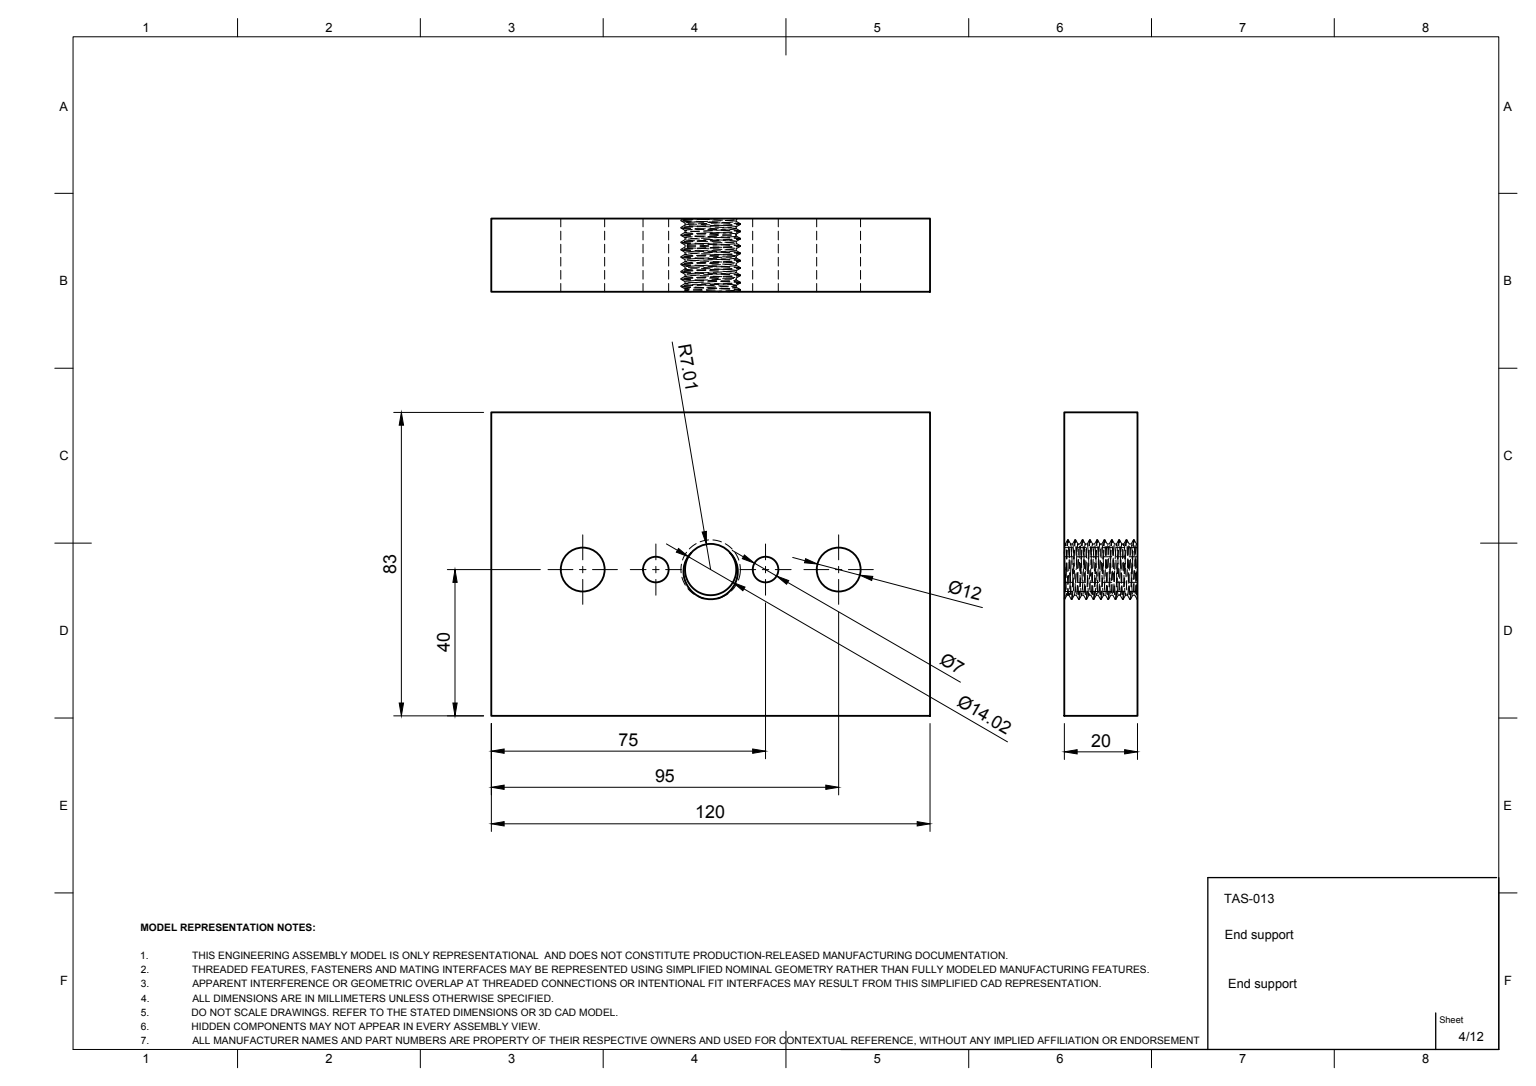
ISO-10303-21;
HEADER;
/* Generated by software containing ST-Developer
 * from STEP Tools, Inc. (www.steptools.com) 
 */

FILE_DESCRIPTION(
/* description */ (
'Independent guided parallel-jaw bracket clamp. Two12mm guide rods, re
placeable bronze sleeves, captured swiveling spindle, replaceable jaw 
pads and modeled M16x2 screw. Native slider/revolute joints linked2mm 
per revolution. Nominal opening0..122 with initial28mm. Base and two i
dentical supports welded. Standard fits, weld details and clamp load r
equire engineering selection.'),
/* implementation_level */ '2;1');

FILE_NAME(
/* name */ 'End support.step',
/* time_stamp */ '2026-11-14T09:15:44-08:00',
/* author */ (''),
/* organization */ (''),
/* preprocessor_version */ 'ST-DEVELOPER v20.2',
/* originating_system */ 'Autodesk Translation Framework v15.17.0.0',
/* authorisation */ '');

FILE_SCHEMA (('AUTOMOTIVE_DESIGN { 1 0 10303 214 3 1 1 }'));
ENDSEC;

DATA;
#10=MECHANICAL_DESIGN_GEOMETRIC_PRESENTATION_REPRESENTATION('',(#920),#105806);
#97=B_SPLINE_SURFACE_WITH_KNOTS('',3,3,((#78284,#78285,#78286,#78287,#78288,
#78289,#78290,#78291,#78292,#78293,#78294,#78295,#78296,#78297,#78298,#78299,
#78300,#78301,#78302,#78303,#78304,#78305,#78306,#78307,#78308,#78309,#78310,
#78311,#78312,#78313,#78314,#78315,#78316,#78317,#78318,#78319,#78320,#78321,
#78322,#78323,#78324,#78325,#78326,#78327,#78328,#78329,#78330,#78331,#78332,
#78333,#78334,#78335,#78336,#78337,#78338,#78339,#78340,#78341,#78342,#78343,
#78344,#78345,#78346,#78347,#78348,#78349,#78350,#78351,#78352,#78353,#78354,
#78355,#78356,#78357,#78358,#78359,#78360,#78361,#78362,#78363,#78364,#78365,
#78366,#78367,#78368,#78369,#78370,#78371,#78372,#78373,#78374,#78375,#78376,
#78377,#78378,#78379,#78380,#78381,#78382,#78383,#78384,#78385,#78386,#78387,
#78388,#78389,#78390,#78391,#78392,#78393,#78394,#78395,#78396,#78397,#78398,
#78399,#78400,#78401,#78402,#78403,#78404,#78405,#78406,#78407,#78408,#78409,
#78410,#78411,#78412,#78413,#78414,#78415,#78416),(#78417,#78418,#78419,
#78420,#78421,#78422,#78423,#78424,#78425,#78426,#78427,#78428,#78429,#78430,
#78431,#78432,#78433,#78434,#78435,#78436,#78437,#78438,#78439,#78440,#78441,
#78442,#78443,#78444,#78445,#78446,#78447,#78448,#78449,#78450,#78451,#78452,
#78453,#78454,#78455,#78456,#78457,#78458,#78459,#78460,#78461,#78462,#78463,
#78464,#78465,#78466,#78467,#78468,#78469,#78470,#78471,#78472,#78473,#78474,
#78475,#78476,#78477,#78478,#78479,#78480,#78481,#78482,#78483,#78484,#78485,
#78486,#78487,#78488,#78489,#78490,#78491,#78492,#78493,#78494,#78495,#78496,
#78497,#78498,#78499,#78500,#78501,#78502,#78503,#78504,#78505,#78506,#78507,
#78508,#78509,#78510,#78511,#78512,#78513,#78514,#78515,#78516,#78517,#78518,
#78519,#78520,#78521,#78522,#78523,#78524,#78525,#78526,#78527,#78528,#78529,
#78530,#78531,#78532,#78533,#78534,#78535,#78536,#78537,#78538,#78539,#78540,
#78541,#78542,#78543,#78544,#78545,#78546,#78547,#78548,#78549),(#78550,
#78551,#78552,#78553,#78554,#78555,#78556,#78557,#78558,#78559,#78560,#78561,
#78562,#78563,#78564,#78565,#78566,#78567,#78568,#78569,#78570,#78571,#78572,
#78573,#78574,#78575,#78576,#78577,#78578,#78579,#78580,#78581,#78582,#78583,
#78584,#78585,#78586,#78587,#78588,#78589,#78590,#78591,#78592,#78593,#78594,
#78595,#78596,#78597,#78598,#78599,#78600,#78601,#78602,#78603,#78604,#78605,
#78606,#78607,#78608,#78609,#78610,#78611,#78612,#78613,#78614,#78615,#78616,
#78617,#78618,#78619,#78620,#78621,#78622,#78623,#78624,#78625,#78626,#78627,
#78628,#78629,#78630,#78631,#78632,#78633,#78634,#78635,#78636,#78637,#78638,
#78639,#78640,#78641,#78642,#78643,#78644,#78645,#78646,#78647,#78648,#78649,
#78650,#78651,#78652,#78653,#78654,#78655,#78656,#78657,#78658,#78659,#78660,
#78661,#78662,#78663,#78664,#78665,#78666,#78667,#78668,#78669,#78670,#78671,
#78672,#78673,#78674,#78675,#78676,#78677,#78678,#78679,#78680,#78681,#78682),
(#78683,#78684,#78685,#78686,#78687,#78688,#78689,#78690,#78691,#78692,
#78693,#78694,#78695,#78696,#78697,#78698,#78699,#78700,#78701,#78702,#78703,
#78704,#78705,#78706,#78707,#78708,#78709,#78710,#78711,#78712,#78713,#78714,
#78715,#78716,#78717,#78718,#78719,#78720,#78721,#78722,#78723,#78724,#78725,
#78726,#78727,#78728,#78729,#78730,#78731,#78732,#78733,#78734,#78735,#78736,
#78737,#78738,#78739,#78740,#78741,#78742,#78743,#78744,#78745,#78746,#78747,
#78748,#78749,#78750,#78751,#78752,#78753,#78754,#78755,#78756,#78757,#78758,
#78759,#78760,#78761,#78762,#78763,#78764,#78765,#78766,#78767,#78768,#78769,
#78770,#78771,#78772,#78773,#78774,#78775,#78776,#78777,#78778,#78779,#78780,
#78781,#78782,#78783,#78784,#78785,#78786,#78787,#78788,#78789,#78790,#78791,
#78792,#78793,#78794,#78795,#78796,#78797,#78798,#78799,#78800,#78801,#78802,
#78803,#78804,#78805,#78806,#78807,#78808,#78809,#78810,#78811,#78812,#78813,
#78814,#78815)),.UNSPECIFIED.,.F.,.F.,.F.,(4,4),(4,1,1,1,1,1,1,1,1,1,1,
1,1,1,1,1,1,1,1,1,1,1,1,1,1,1,1,1,1,1,1,1,1,1,1,1,1,1,1,1,1,1,1,1,1,1,1,
1,1,1,1,1,1,1,1,1,1,1,1,1,1,1,1,1,1,1,1,1,1,1,1,1,1,1,1,1,1,1,1,1,1,1,1,
1,1,1,1,1,1,1,1,1,1,1,1,1,1,1,1,1,1,1,1,1,1,1,1,1,1,1,1,1,1,1,1,1,1,1,1,
1,1,1,1,1,1,1,1,1,1,1,4),(-8.529467209505E-5,0.128694174119411),(11.8548225190662,
12.3537726257656,12.8526374377929,13.3515022498203,13.8503670618476,14.3492318738749,
14.8480966859023,15.3469614979296,15.8458263099569,16.3446911219842,16.8435559340116,
17.3424207460389,17.8412855580662,18.3401503700936,18.8390151821209,19.3378799941482,
19.8367448061755,20.3356096182029,20.8344744302302,21.3333392422575,21.8322040542849,
22.3310688663122,22.8299336783395,23.3287984903668,23.8276633023942,24.3265281144215,
24.8253929264488,25.3242577384762,25.8231225505035,26.3219873625308,26.8208521745581,
27.3197169865855,27.8185817986128,28.3174466106401,28.8163114226675,29.3151762346948,
29.8140410467221,30.3129058587495,30.8117706707768,31.3106354828041,31.8095002948314,
32.3083651068588,32.8072299188861,33.3060947309134,33.8049595429408,34.3038243549681,
34.8026891669954,35.3015539790227,35.8004187910501,36.2992836030774,36.7981484151047,
37.2970132271321,37.7958780391594,38.2947428511867,38.793607663214,39.2924724752414,
39.7913372872687,40.290202099296,40.7890669113234,41.2879317233507,41.786796535378,
42.2856613474054,42.7845261594327,43.28339097146,43.7822557834873,44.2811205955147,
44.779985407542,45.2788502195693,45.7777150315967,46.276579843624,46.7754446556513,
47.2743094676786,47.773174279706,48.2720390917333,48.7709039037606,49.269768715788,
49.7686335278153,50.2674983398426,50.76636315187,51.2652279638973,51.7640927759246,
52.2629575879519,52.7618223999793,53.2606872120066,53.7595520240339,54.2584168360613,
54.7572816480886,55.2561464601159,55.7550112721432,56.2538760841706,56.7527408961979,
57.2516057082252,57.7504705202526,58.2493353322799,58.7482001443072,59.2470649563345,
59.7459297683619,60.2447945803892,60.7436593924165,61.2425242044439,61.7413890164712,
62.2402538284985,62.7391186405258,63.2379834525532,63.7368482645805,64.2357130766078,
64.7345778886352,65.2334427006625,65.7323075126898,66.2311723247172,66.7300371367445,
67.2289019487718,67.7277667607991,68.2266315728265,68.7254963848538,69.2243611968811,
69.7232260089085,70.2220908209358,70.7209556329631,71.2198204449904,71.7186852570178,
72.2175500690451,72.7164148810724,73.2152796930998,73.7141445051271,74.2130093171544,
74.7118741291818,75.2107389412091,75.7096037532364,76.2084685652637,76.7073333772911),
 .UNSPECIFIED.);
#98=B_SPLINE_SURFACE_WITH_KNOTS('',3,3,((#79039,#79040,#79041,#79042,#79043,
#79044,#79045,#79046,#79047,#79048,#79049,#79050,#79051,#79052,#79053,#79054,
#79055,#79056,#79057,#79058,#79059,#79060,#79061,#79062,#79063,#79064,#79065,
#79066,#79067,#79068,#79069,#79070,#79071,#79072,#79073,#79074,#79075,#79076,
#79077,#79078,#79079,#79080,#79081,#79082,#79083,#79084,#79085,#79086,#79087,
#79088,#79089,#79090,#79091,#79092,#79093,#79094,#79095,#79096,#79097,#79098,
#79099,#79100,#79101,#79102,#79103,#79104,#79105,#79106,#79107,#79108,#79109,
#79110,#79111,#79112,#79113,#79114,#79115,#79116,#79117,#79118,#79119,#79120,
#79121,#79122,#79123,#79124,#79125,#79126,#79127,#79128,#79129,#79130,#79131,
#79132,#79133,#79134,#79135,#79136,#79137,#79138,#79139,#79140,#79141,#79142,
#79143,#79144,#79145,#79146,#79147,#79148,#79149,#79150,#79151,#79152,#79153,
#79154,#79155,#79156,#79157,#79158,#79159,#79160,#79161,#79162,#79163,#79164,
#79165,#79166,#79167,#79168,#79169,#79170,#79171),(#79172,#79173,#79174,
#79175,#79176,#79177,#79178,#79179,#79180,#79181,#79182,#79183,#79184,#79185,
#79186,#79187,#79188,#79189,#79190,#79191,#79192,#79193,#79194,#79195,#79196,
#79197,#79198,#79199,#79200,#79201,#79202,#79203,#79204,#79205,#79206,#79207,
#79208,#79209,#79210,#79211,#79212,#79213,#79214,#79215,#79216,#79217,#79218,
#79219,#79220,#79221,#79222,#79223,#79224,#79225,#79226,#79227,#79228,#79229,
#79230,#79231,#79232,#79233,#79234,#79235,#79236,#79237,#79238,#79239,#79240,
#79241,#79242,#79243,#79244,#79245,#79246,#79247,#79248,#79249,#79250,#79251,
#79252,#79253,#79254,#79255,#79256,#79257,#79258,#79259,#79260,#79261,#79262,
#79263,#79264,#79265,#79266,#79267,#79268,#79269,#79270,#79271,#79272,#79273,
#79274,#79275,#79276,#79277,#79278,#79279,#79280,#79281,#79282,#79283,#79284,
#79285,#79286,#79287,#79288,#79289,#79290,#79291,#79292,#79293,#79294,#79295,
#79296,#79297,#79298,#79299,#79300,#79301,#79302,#79303,#79304),(#79305,
#79306,#79307,#79308,#79309,#79310,#79311,#79312,#79313,#79314,#79315,#79316,
#79317,#79318,#79319,#79320,#79321,#79322,#79323,#79324,#79325,#79326,#79327,
#79328,#79329,#79330,#79331,#79332,#79333,#79334,#79335,#79336,#79337,#79338,
#79339,#79340,#79341,#79342,#79343,#79344,#79345,#79346,#79347,#79348,#79349,
#79350,#79351,#79352,#79353,#79354,#79355,#79356,#79357,#79358,#79359,#79360,
#79361,#79362,#79363,#79364,#79365,#79366,#79367,#79368,#79369,#79370,#79371,
#79372,#79373,#79374,#79375,#79376,#79377,#79378,#79379,#79380,#79381,#79382,
#79383,#79384,#79385,#79386,#79387,#79388,#79389,#79390,#79391,#79392,#79393,
#79394,#79395,#79396,#79397,#79398,#79399,#79400,#79401,#79402,#79403,#79404,
#79405,#79406,#79407,#79408,#79409,#79410,#79411,#79412,#79413,#79414,#79415,
#79416,#79417,#79418,#79419,#79420,#79421,#79422,#79423,#79424,#79425,#79426,
#79427,#79428,#79429,#79430,#79431,#79432,#79433,#79434,#79435,#79436,#79437),
(#79438,#79439,#79440,#79441,#79442,#79443,#79444,#79445,#79446,#79447,
#79448,#79449,#79450,#79451,#79452,#79453,#79454,#79455,#79456,#79457,#79458,
#79459,#79460,#79461,#79462,#79463,#79464,#79465,#79466,#79467,#79468,#79469,
#79470,#79471,#79472,#79473,#79474,#79475,#79476,#79477,#79478,#79479,#79480,
#79481,#79482,#79483,#79484,#79485,#79486,#79487,#79488,#79489,#79490,#79491,
#79492,#79493,#79494,#79495,#79496,#79497,#79498,#79499,#79500,#79501,#79502,
#79503,#79504,#79505,#79506,#79507,#79508,#79509,#79510,#79511,#79512,#79513,
#79514,#79515,#79516,#79517,#79518,#79519,#79520,#79521,#79522,#79523,#79524,
#79525,#79526,#79527,#79528,#79529,#79530,#79531,#79532,#79533,#79534,#79535,
#79536,#79537,#79538,#79539,#79540,#79541,#79542,#79543,#79544,#79545,#79546,
#79547,#79548,#79549,#79550,#79551,#79552,#79553,#79554,#79555,#79556,#79557,
#79558,#79559,#79560,#79561,#79562,#79563,#79564,#79565,#79566,#79567,#79568,
#79569,#79570)),.UNSPECIFIED.,.F.,.F.,.F.,(4,4),(4,1,1,1,1,1,1,1,1,1,1,
1,1,1,1,1,1,1,1,1,1,1,1,1,1,1,1,1,1,1,1,1,1,1,1,1,1,1,1,1,1,1,1,1,1,1,1,
1,1,1,1,1,1,1,1,1,1,1,1,1,1,1,1,1,1,1,1,1,1,1,1,1,1,1,1,1,1,1,1,1,1,1,1,
1,1,1,1,1,1,1,1,1,1,1,1,1,1,1,1,1,1,1,1,1,1,1,1,1,1,1,1,1,1,1,1,1,1,1,1,
1,1,1,1,1,1,1,1,1,1,1,4),(-6.05230187934505E-5,0.12871890615391),(14.3988535768129,
14.8977183888402,15.3965832008676,15.8954480128949,16.3943128249222,16.8931776369496,
17.3920424489769,17.8909072610042,18.3897720730315,18.8886368850589,19.3875016970862,
19.8863665091135,20.3852313211409,20.8840961331682,21.3829609451955,21.8818257572228,
22.3806905692502,22.8795553812775,23.3784201933048,23.8772850053322,24.3761498173595,
24.8750146293868,25.3738794414141,25.8727442534415,26.3716090654688,26.8704738774961,
27.3693386895235,27.8682035015508,28.3670683135781,28.8659331256054,29.3647979376328,
29.8636627496601,30.3625275616874,30.8613923737148,31.3602571857421,31.8591219977694,
32.3579868097967,32.8568516218241,33.3557164338514,33.8545812458787,34.3534460579061,
34.8523108699334,35.3511756819607,35.8500404939881,36.3489053060154,36.8477701180427,
37.34663493007,37.8454997420974,38.3443645541247,38.843229366152,39.3420941781794,
39.8409589902067,40.339823802234,40.8386886142613,41.3375534262887,41.836418238316,
42.3352830503433,42.8341478623707,43.333012674398,43.8318774864253,44.3307422984526,
44.82960711048,45.3284719225073,45.8273367345346,46.326201546562,46.8250663585893,
47.3239311706166,47.8227959826439,48.3216607946713,48.8205256066986,49.3193904187259,
49.8182552307533,50.3171200427806,50.8159848548079,51.3148496668353,51.8137144788626,
52.3125792908899,52.8114441029172,53.3103089149446,53.8091737269719,54.3080385389992,
54.8069033510266,55.3057681630539,55.8046329750812,56.3034977871085,56.8023625991359,
57.3012274111632,57.8000922231905,58.2989570352179,58.7978218472452,59.2966866592725,
59.7955514712998,60.2944162833272,60.7932810953545,61.2921459073818,61.7910107194092,
62.2898755314365,62.7887403434638,63.2876051554911,63.7864699675185,64.2853347795458,
64.7841995915731,65.2830644036005,65.7819292156278,66.2807940276551,66.7796588396825,
67.2785236517098,67.7773884637371,68.2762532757644,68.7751180877918,69.2739828998191,
69.7728477118464,70.2717125238738,70.7705773359011,71.2694421479284,71.7683069599557,
72.2671717719831,72.7660365840104,73.2649013960377,73.7637662080651,74.2626310200924,
74.7614958321197,75.260360644147,75.7592254561744,76.2580902682017,76.756955080229,
77.2558198922564,77.7546847042837,78.253549516311,78.7524143283383,79.2513644065442),
 .UNSPECIFIED.);
#564=B_SPLINE_CURVE_WITH_KNOTS('',3,(#71903,#71904,#71905,#71906,#71907,
#71908,#71909,#71910),.UNSPECIFIED.,.F.,.F.,(4,1,1,1,1,4),(74.4819856391522,
74.7118741291818,75.2107389412091,75.7096037532364,76.2084685652637,76.7073333772911),
 .UNSPECIFIED.);
#565=B_SPLINE_CURVE_WITH_KNOTS('',3,(#71913,#71914,#71915,#71916,#71917,
#71918,#71919,#71920,#71921),.UNSPECIFIED.,.F.,.F.,(4,1,1,1,1,1,4),(74.4820002615382,
74.7614958321197,75.260360644147,75.7592254561744,76.2580902682017,76.756955080229,
77.2307066486088),.UNSPECIFIED.);
#566=B_SPLINE_CURVE_WITH_KNOTS('',3,(#71927,#71928,#71929,#71930,#71931,
#71932,#71933,#71934,#71935,#71936,#71937,#71938,#71939,#71940,#71941,#71942,
#71943,#71944,#71945,#71946,#71947,#71948,#71949,#71950,#71951,#71952,#71953,
#71954,#71955,#71956,#71957,#71958,#71959,#71960,#71961,#71962,#71963,#71964,
#71965,#71966,#71967,#71968,#71969,#71970,#71971,#71972,#71973,#71974,#71975,
#71976,#71977,#71978,#71979,#71980,#71981,#71982,#71983,#71984,#71985,#71986,
#71987,#71988,#71989,#71990,#71991,#71992,#71993,#71994,#71995,#71996,#71997,
#71998,#71999,#72000,#72001,#72002,#72003,#72004,#72005,#72006,#72007,#72008,
#72009,#72010,#72011,#72012,#72013,#72014,#72015,#72016,#72017,#72018,#72019,
#72020,#72021,#72022,#72023,#72024,#72025,#72026,#72027,#72028,#72029,#72030,
#72031,#72032,#72033,#72034,#72035,#72036,#72037,#72038,#72039,#72040,#72041,
#72042,#72043,#72044,#72045,#72046,#72047,#72048,#72049,#72050,#72051,#72052,
#72053,#72054,#72055,#72056,#72057,#72058,#72059,#72060,#72061,#72062,#72063,
#72064,#72065,#72066,#72067,#72068,#72069,#72070,#72071,#72072,#72073,#72074,
#72075,#72076,#72077,#72078,#72079,#72080,#72081,#72082,#72083,#72084,#72085,
#72086,#72087,#72088,#72089,#72090,#72091,#72092,#72093,#72094,#72095,#72096,
#72097,#72098,#72099,#72100,#72101),.UNSPECIFIED.,.F.,.F.,(4,3,3,3,3,3,
3,3,3,3,3,3,3,3,3,3,3,3,3,3,3,3,3,3,3,3,3,3,3,3,3,3,3,3,3,3,3,3,3,3,3,3,
3,3,3,3,3,3,3,3,3,3,3,3,3,3,3,3,4),(68.1987975186712,68.2266315728265,68.3041236122402,
68.3816013676368,68.4590704189412,68.5365456775087,68.6140206493277,68.6915121862316,
68.7254963848538,68.8029883992075,68.8804661294451,68.9579351555709,69.0354103891201,
69.1128853360578,69.1903768484489,69.2243611968811,69.3018532647296,69.3793310486332,
69.456800128424,69.5342754152362,69.6117504151087,69.6892419796001,69.7232260089085,
69.800717988916,69.8781956847726,69.9556646765945,70.0331398762059,70.1106147894785,
70.1881062688295,70.2220908209358,70.2995828974163,70.3770606897927,70.4545297778736,
70.5320050726442,70.6094800802699,70.6869716521594,70.7209556329631,70.7984477160451,
70.8759255156548,70.9533946115695,71.0308699150024,71.1083449317504,71.1858365133831,
71.2198204449904,71.2973121319933,71.3747895331616,71.4522582295674,71.5297331348839,
71.6072077550478,71.684698944971,71.7186852570178,71.7961782868195,71.8736570365031,
71.9511270827911,72.0286033299696,72.1060792849236,72.1835717903897,72.2175500690451,
72.2566310325652),.UNSPECIFIED.);
#567=B_SPLINE_CURVE_WITH_KNOTS('',3,(#72102,#72103,#72104,#72105,#72106,
#72107,#72108,#72109),.UNSPECIFIED.,.F.,.F.,(4,1,1,1,1,4),(72.2566310687215,
72.7164148810724,73.2152796930998,73.7141445051271,74.2130093171544,74.4819856391522),
 .UNSPECIFIED.);
#568=B_SPLINE_CURVE_WITH_KNOTS('',3,(#72111,#72112,#72113,#72114,#72115,
#72116,#72117,#72118,#72119),.UNSPECIFIED.,.F.,.F.,(4,1,1,1,1,1,4),(72.2566310325652,
72.2671717719831,72.7660365840104,73.2649013960377,73.7637662080651,74.2626310200924,
74.4820002615382),.UNSPECIFIED.);
#569=B_SPLINE_CURVE_WITH_KNOTS('',3,(#72120,#72121,#72122,#72123,#72124,
#72125,#72126,#72127,#72128,#72129,#72130,#72131,#72132,#72133,#72134,#72135,
#72136,#72137,#72138,#72139,#72140,#72141,#72142,#72143,#72144,#72145,#72146,
#72147,#72148,#72149,#72150,#72151,#72152,#72153,#72154,#72155,#72156,#72157,
#72158,#72159,#72160,#72161,#72162,#72163,#72164,#72165,#72166,#72167,#72168,
#72169,#72170,#72171,#72172,#72173,#72174,#72175,#72176,#72177,#72178,#72179,
#72180,#72181,#72182,#72183,#72184,#72185,#72186,#72187,#72188,#72189,#72190,
#72191,#72192,#72193,#72194,#72195,#72196,#72197,#72198,#72199,#72200,#72201,
#72202,#72203,#72204,#72205,#72206,#72207,#72208,#72209,#72210,#72211,#72212,
#72213,#72214,#72215,#72216,#72217,#72218,#72219,#72220,#72221,#72222,#72223,
#72224,#72225,#72226,#72227,#72228,#72229,#72230,#72231,#72232,#72233,#72234,
#72235,#72236,#72237,#72238,#72239,#72240,#72241,#72242,#72243,#72244,#72245,
#72246,#72247,#72248,#72249,#72250,#72251,#72252,#72253,#72254,#72255,#72256,
#72257,#72258,#72259,#72260,#72261,#72262,#72263,#72264,#72265,#72266,#72267,
#72268,#72269,#72270,#72271,#72272,#72273,#72274,#72275,#72276,#72277,#72278,
#72279,#72280,#72281,#72282,#72283,#72284,#72285,#72286,#72287,#72288,#72289,
#72290,#72291),.UNSPECIFIED.,.F.,.F.,(4,3,3,3,3,3,3,3,3,3,3,3,3,3,3,3,3,
3,3,3,3,3,3,3,3,3,3,3,3,3,3,3,3,3,3,3,3,3,3,3,3,3,3,3,3,3,3,3,3,3,3,3,3,
3,3,3,3,4),(68.1987898047183,68.2762532757644,68.3537453085195,68.4312230572261,
68.5086921018308,68.586167353733,68.6636423189185,68.7411338492811,68.7751180877918,
68.8526101196304,68.9300878674179,69.0075569111027,69.0850321620932,69.1625071263726,
69.2399986558434,69.2739828998191,69.3514749330283,69.4289526821889,69.5064217272455,
69.5838969795948,69.6613719452233,69.7388634760199,69.7728477118464,69.8503397438658,
69.9278174918377,70.0052865357114,70.0827617868932,70.1602367513658,70.2377282810308,
70.2717125238738,70.3492045547049,70.4266823014742,70.5041513441335,70.5816265940954,
70.6591015573465,70.736593085796,70.7705773359011,70.8480693754309,70.9255471309442,
71.0030161823662,71.0804914410497,71.1579664129848,71.2354579500022,71.2694421479284,
71.3469341620217,71.4244118919975,71.5018809178624,71.5793561511515,71.6568310978316,
71.7343226099682,71.7683069599557,71.8457247371354,71.9231279927475,72.0005225461464,
72.077923117042,72.15532396466,72.2327409413495,72.2566310325652),
 .UNSPECIFIED.);
#570=B_SPLINE_CURVE_WITH_KNOTS('',3,(#72297,#72298,#72299,#72300,#72301,
#72302,#72303,#72304,#72305,#72306,#72307,#72308),.UNSPECIFIED.,.F.,.F.,
(4,1,1,1,1,1,1,1,1,4),(61.9156408615241,62.2402538284985,62.7391186405258,
63.2379834525532,63.7368482645805,64.2357130766078,64.7345778886352,65.2334427006625,
65.7323075126898,65.9734457190118),.UNSPECIFIED.);
#571=B_SPLINE_CURVE_WITH_KNOTS('',3,(#72309,#72310,#72311,#72312,#72313,
#72314,#72315,#72316,#72317,#72318,#72319,#72320,#72321,#72322,#72323,#72324,
#72325,#72326,#72327,#72328,#72329,#72330,#72331,#72332,#72333,#72334,#72335,
#72336,#72337,#72338,#72339,#72340,#72341,#72342,#72343,#72344,#72345,#72346,
#72347,#72348,#72349,#72350,#72351,#72352,#72353,#72354,#72355,#72356,#72357,
#72358,#72359,#72360,#72361,#72362,#72363,#72364,#72365,#72366,#72367,#72368,
#72369,#72370,#72371,#72372,#72373,#72374,#72375,#72376,#72377,#72378,#72379,
#72380,#72381,#72382,#72383,#72384,#72385,#72386,#72387,#72388,#72389,#72390,
#72391,#72392,#72393,#72394,#72395,#72396,#72397,#72398,#72399,#72400,#72401,
#72402),.UNSPECIFIED.,.F.,.F.,(4,3,3,3,3,3,3,3,3,3,3,3,3,3,3,3,3,3,3,3,
3,3,3,3,3,3,3,3,3,3,3,4),(65.9734457253856,66.051752866185,66.1300656952307,
66.2083969560539,66.2311723247172,66.3086643565655,66.3861421043627,66.4636111480579,
66.5410863990578,66.6185613633469,66.6960528928273,66.7300371367445,66.8075291699426,
66.8850069190923,66.9624759641383,67.0399512164768,67.1174261820946,67.1949177128806,
67.2289019487718,67.3063939807927,67.3838717287663,67.4613407726409,67.5388160238239,
67.6162909882975,67.6937825179636,67.7277667607991,67.8052584948873,67.8827358464432,
67.9617512645002,68.0392239583848,68.119010738528,68.1987975186712),
 .UNSPECIFIED.);
#572=B_SPLINE_CURVE_WITH_KNOTS('',3,(#72404,#72405,#72406,#72407,#72408,
#72409,#72410,#72411,#72412,#72413,#72414,#72415,#72416,#72417,#72418,#72419,
#72420,#72421,#72422,#72423,#72424,#72425,#72426,#72427,#72428,#72429,#72430,
#72431,#72432,#72433,#72434,#72435,#72436,#72437,#72438,#72439,#72440,#72441,
#72442,#72443,#72444,#72445,#72446,#72447,#72448,#72449,#72450,#72451,#72452,
#72453,#72454,#72455,#72456,#72457,#72458,#72459,#72460,#72461,#72462,#72463,
#72464,#72465,#72466,#72467,#72468,#72469,#72470,#72471,#72472,#72473,#72474,
#72475,#72476,#72477,#72478,#72479,#72480,#72481,#72482,#72483,#72484,#72485,
#72486,#72487,#72488,#72489,#72490,#72491,#72492,#72493,#72494,#72495,#72496,
#72497),.UNSPECIFIED.,.F.,.F.,(4,3,3,3,3,3,3,3,3,3,3,3,3,3,3,3,3,3,3,3,
3,3,3,3,3,3,3,3,3,3,3,4),(65.9734457253856,66.05113864352,66.1288303647685,
66.2065431816206,66.2807940276551,66.3582860600736,66.4357638084426,66.5132328527091,
66.5907081042758,66.6681830691279,66.7456745991621,66.7796588396825,66.8571508721125,
66.934628620493,67.0120976647703,67.0895729163482,67.1670478812115,67.2445394112565,
67.2785236517098,67.3560156841782,67.433493432597,67.5109624769137,67.5884377285306,
67.6659126934328,67.7434042235161,67.7773884637371,67.8548798500932,67.9323566782865,
68.0098309919021,68.0873000058441,68.1647781672896,68.1987898047183),
 .UNSPECIFIED.);
#573=B_SPLINE_CURVE_WITH_KNOTS('',3,(#72498,#72499,#72500,#72501,#72502,
#72503,#72504,#72505,#72506,#72507,#72508,#72509),.UNSPECIFIED.,.F.,.F.,
(4,1,1,1,1,1,1,1,1,4),(61.9156464171414,62.2898755314365,62.7887403434638,
63.2876051554911,63.7864699675185,64.2853347795458,64.7841995915731,65.2830644036005,
65.7819292156278,65.9734456898724),.UNSPECIFIED.);
#574=B_SPLINE_CURVE_WITH_KNOTS('',3,(#72515,#72516,#72517,#72518,#72519,
#72520,#72521,#72522,#72523,#72524,#72525,#72526,#72527,#72528,#72529,#72530,
#72531,#72532,#72533,#72534,#72535,#72536,#72537,#72538,#72539,#72540,#72541,
#72542,#72543,#72544,#72545,#72546,#72547,#72548,#72549,#72550,#72551,#72552,
#72553,#72554,#72555,#72556,#72557,#72558,#72559,#72560,#72561,#72562,#72563,
#72564,#72565,#72566,#72567,#72568,#72569,#72570,#72571,#72572,#72573,#72574,
#72575,#72576,#72577,#72578,#72579,#72580,#72581,#72582,#72583,#72584,#72585,
#72586,#72587,#72588,#72589,#72590,#72591,#72592,#72593,#72594,#72595,#72596,
#72597,#72598,#72599,#72600,#72601,#72602,#72603,#72604,#72605,#72606,#72607,
#72608,#72609,#72610,#72611,#72612,#72613,#72614,#72615,#72616,#72617,#72618,
#72619,#72620,#72621,#72622,#72623,#72624,#72625,#72626,#72627,#72628,#72629,
#72630,#72631,#72632,#72633,#72634,#72635,#72636,#72637,#72638,#72639,#72640,
#72641,#72642,#72643,#72644,#72645,#72646,#72647,#72648,#72649,#72650,#72651,
#72652,#72653,#72654,#72655,#72656,#72657,#72658,#72659,#72660,#72661,#72662,
#72663,#72664,#72665,#72666,#72667,#72668,#72669,#72670,#72671,#72672,#72673,
#72674,#72675,#72676,#72677,#72678,#72679,#72680,#72681,#72682,#72683,#72684,
#72685,#72686),.UNSPECIFIED.,.F.,.F.,(4,3,3,3,3,3,3,3,3,3,3,3,3,3,3,3,3,
3,3,3,3,3,3,3,3,3,3,3,3,3,3,3,3,3,3,3,3,3,3,3,3,3,3,3,3,3,3,3,3,3,3,3,3,
3,3,3,3,4),(55.6324185145553,55.7099104487287,55.7550112721432,55.8325033045725,
55.9099810529522,55.9874500972293,56.0649253488068,56.1424003136698,56.2198918437144,
56.2538760841706,56.3313681165998,56.4088458649798,56.4863149092575,56.5637901608348,
56.6412651256974,56.718756655742,56.7527408961979,56.830232928627,56.9077106770066,
56.985179721284,57.0626549728614,57.1401299377238,57.2176214677687,57.2516057082252,
57.3290977406545,57.4065754890343,57.484044533311,57.5615197848885,57.6389947497512,
57.7164862797957,57.7504705202526,57.8279625526819,57.9054403010617,57.9829093453387,
58.0603845969162,58.1378595617786,58.2153510918235,58.2493353322799,58.3268273647091,
58.404305113089,58.4817741573666,58.5592494089439,58.6367243738066,58.7142159038511,
58.7482001443072,58.8256921767366,58.9031699251163,58.9806389693927,59.05811422097,
59.1355891858328,59.2130807158776,59.2470649563345,59.3242792098715,59.4014782880975,
59.4786774007806,59.5558721176712,59.6330828530534,59.6902604182061),
 .UNSPECIFIED.);
#575=B_SPLINE_CURVE_WITH_KNOTS('',3,(#72687,#72688,#72689,#72690,#72691,
#72692,#72693,#72694,#72695),.UNSPECIFIED.,.F.,.F.,(4,1,1,1,1,1,4),(59.6902604182061,
59.7459297683619,60.2447945803892,60.7436593924165,61.2425242044439,61.7413890164712,
61.9156408615241),.UNSPECIFIED.);
#576=B_SPLINE_CURVE_WITH_KNOTS('',3,(#72697,#72698,#72699,#72700,#72701,
#72702,#72703,#72704,#72705),.UNSPECIFIED.,.F.,.F.,(4,1,1,1,1,1,4),(59.6902604182061,
59.7955514712998,60.2944162833272,60.7932810953545,61.2921459073818,61.7910107194092,
61.9156464171414),.UNSPECIFIED.);
#577=B_SPLINE_CURVE_WITH_KNOTS('',3,(#72706,#72707,#72708,#72709,#72710,
#72711,#72712,#72713,#72714,#72715,#72716,#72717,#72718,#72719,#72720,#72721,
#72722,#72723,#72724,#72725,#72726,#72727,#72728,#72729,#72730,#72731,#72732,
#72733,#72734,#72735,#72736,#72737,#72738,#72739,#72740,#72741,#72742,#72743,
#72744,#72745,#72746,#72747,#72748,#72749,#72750,#72751,#72752,#72753,#72754,
#72755,#72756,#72757,#72758,#72759,#72760,#72761,#72762,#72763,#72764,#72765,
#72766,#72767,#72768,#72769,#72770,#72771,#72772,#72773,#72774,#72775,#72776,
#72777,#72778,#72779,#72780,#72781,#72782,#72783,#72784,#72785,#72786,#72787,
#72788,#72789,#72790,#72791,#72792,#72793,#72794,#72795,#72796,#72797,#72798,
#72799,#72800,#72801,#72802,#72803,#72804,#72805,#72806,#72807,#72808,#72809,
#72810,#72811,#72812,#72813,#72814,#72815,#72816,#72817,#72818,#72819,#72820,
#72821,#72822,#72823,#72824,#72825,#72826,#72827,#72828,#72829,#72830,#72831,
#72832,#72833,#72834,#72835,#72836,#72837,#72838,#72839,#72840,#72841,#72842,
#72843,#72844,#72845,#72846,#72847,#72848,#72849,#72850,#72851,#72852,#72853,
#72854,#72855,#72856,#72857,#72858,#72859,#72860,#72861,#72862,#72863,#72864,
#72865,#72866,#72867,#72868,#72869,#72870,#72871,#72872,#72873,#72874,#72875,
#72876,#72877),.UNSPECIFIED.,.F.,.F.,(4,3,3,3,3,3,3,3,3,3,3,3,3,3,3,3,3,
3,3,3,3,3,3,3,3,3,3,3,3,3,3,3,3,3,3,3,3,3,3,3,3,3,3,3,3,3,3,3,3,3,3,3,3,
3,3,3,3,4),(55.6324228066038,55.7098984440576,55.787389714901,55.8046329750812,
55.8821250075104,55.9596027558903,56.0370718001674,56.1145470517449,56.1920220166075,
56.2695135466522,56.3034977871085,56.3809898195378,56.4584675679174,56.5359366121958,
56.6134118637733,56.6908868286361,56.7683783586809,56.8023625991359,56.879854631565,
56.9573323799445,57.0348014242223,57.1122766757997,57.1897516406624,57.2672431707073,
57.3012274111632,57.3787194435924,57.4561971919722,57.5336662362496,57.611141487827,
57.6886164526896,57.7661079827342,57.8000922231905,57.8775842556198,57.9550620039998,
58.0325310482768,58.1100062998543,58.1874812647173,58.2649727947617,58.2989570352179,
58.3764490676469,58.4539268160264,58.5313958603032,58.6088711118807,58.6863460767432,
58.7638376067878,58.7978218472452,58.8753138796745,58.952791628054,59.0302606723321,
59.1077359239092,59.1852108887716,59.262702418816,59.2966866592725,59.3738879299902,
59.4529810520442,59.5301632256214,59.6102118219137,59.6902604182061),
 .UNSPECIFIED.);
#578=B_SPLINE_CURVE_WITH_KNOTS('',3,(#72883,#72884,#72885,#72886,#72887,
#72888,#72889,#72890,#72891,#72892,#72893,#72894,#72895,#72896,#72897,#72898,
#72899,#72900,#72901,#72902,#72903,#72904,#72905,#72906,#72907,#72908,#72909,
#72910,#72911,#72912,#72913,#72914,#72915,#72916,#72917,#72918,#72919,#72920,
#72921,#72922,#72923,#72924,#72925,#72926,#72927,#72928,#72929,#72930,#72931,
#72932,#72933,#72934,#72935,#72936,#72937,#72938,#72939,#72940,#72941,#72942,
#72943,#72944,#72945,#72946,#72947,#72948,#72949,#72950,#72951,#72952,#72953,
#72954,#72955,#72956,#72957,#72958,#72959,#72960,#72961,#72962,#72963,#72964,
#72965,#72966,#72967,#72968,#72969,#72970,#72971,#72972,#72973,#72974,#72975,
#72976,#72977,#72978,#72979,#72980,#72981,#72982,#72983,#72984,#72985,#72986,
#72987,#72988,#72989,#72990,#72991,#72992,#72993,#72994,#72995,#72996,#72997,
#72998,#72999,#73000,#73001,#73002,#73003,#73004,#73005,#73006,#73007,#73008,
#73009,#73010,#73011,#73012,#73013,#73014,#73015,#73016,#73017,#73018,#73019,
#73020,#73021,#73022,#73023,#73024,#73025,#73026,#73027,#73028,#73029,#73030,
#73031,#73032,#73033,#73034,#73035,#73036,#73037,#73038,#73039,#73040,#73041,
#73042,#73043,#73044,#73045,#73046,#73047,#73048,#73049,#73050,#73051,#73052,
#73053,#73054),.UNSPECIFIED.,.F.,.F.,(4,3,3,3,3,3,3,3,3,3,3,3,3,3,3,3,3,
3,3,3,3,3,3,3,3,3,3,3,3,3,3,3,3,3,3,3,3,3,3,3,3,3,3,3,3,3,3,3,3,3,3,3,3,
3,3,3,3,4),(49.3492660090855,49.4267434618947,49.5042123549391,49.5816875286347,
49.6591625602837,49.7366540371569,49.7686335278153,49.8461255602445,49.9236033086243,
50.0010723529015,50.078547604479,50.1560225693416,50.2335140993863,50.2674983398426,
50.3449903722719,50.4224681206516,50.4999371649288,50.5774124165063,50.654887381369,
50.7323789114136,50.76636315187,50.8438551842993,50.921332932679,50.9988019769563,
51.0762772285338,51.1537521933964,51.2312437234411,51.2652279638973,51.3427199963265,
51.4201977447062,51.4976667889834,51.5751420405608,51.6526170054234,51.730108535468,
51.7640927759246,51.8415848083539,51.9190625567337,51.9965316010112,52.0740068525886,
52.1514818174514,52.228973347496,52.2629575879519,52.3404496203811,52.4179273687608,
52.4953964130381,52.5728716646155,52.6503466294781,52.7278381595228,52.7618223999793,
52.8393144324086,52.9167921807885,52.9942612250656,53.0717364766431,53.1492114415058,
53.2267029715505,53.2606872120066,53.3414563463415,53.4070751109153),
 .UNSPECIFIED.);
#579=B_SPLINE_CURVE_WITH_KNOTS('',3,(#73055,#73056,#73057,#73058,#73059,
#73060,#73061,#73062,#73063,#73064,#73065,#73066,#73067,#73068,#73069,#73070,
#73071,#73072,#73073,#73074,#73075,#73076,#73077,#73078,#73079,#73080,#73081,
#73082,#73083,#73084,#73085,#73086,#73087,#73088,#73089,#73090,#73091,#73092,
#73093,#73094,#73095,#73096,#73097,#73098,#73099,#73100,#73101,#73102,#73103,
#73104,#73105,#73106,#73107,#73108,#73109,#73110,#73111,#73112,#73113,#73114,
#73115,#73116,#73117,#73118,#73119,#73120,#73121,#73122,#73123,#73124,#73125,
#73126,#73127,#73128,#73129,#73130,#73131,#73132,#73133,#73134,#73135,#73136,
#73137,#73138,#73139,#73140,#73141,#73142,#73143,#73144,#73145,#73146,#73147,
#73148),.UNSPECIFIED.,.F.,.F.,(4,3,3,3,3,3,3,3,3,3,3,3,3,3,3,3,3,3,3,3,
3,3,3,3,3,3,3,3,3,3,3,4),(53.4070751110265,53.4844112691831,53.5617528045003,
53.6390933869444,53.716451872362,53.7595520240339,53.8370440564632,53.9145218048428,
53.9919908491204,54.0694661006978,54.1469410655606,54.2244325956052,54.2584168360613,
54.3359088684906,54.4133866168704,54.4908556611472,54.5683309127246,54.6458058775878,
54.7232974076326,54.7572816480886,54.8347736805178,54.9122514288974,54.9897204731745,
55.0671957247518,55.1446706896146,55.2221622196592,55.2561464601159,55.3336377293316,
55.4111196629735,55.4885910423118,55.5660683959404,55.6324185145553),
 .UNSPECIFIED.);
#580=B_SPLINE_CURVE_WITH_KNOTS('',3,(#73150,#73151,#73152,#73153,#73154,
#73155,#73156,#73157,#73158,#73159,#73160,#73161,#73162,#73163,#73164,#73165,
#73166,#73167,#73168,#73169,#73170,#73171,#73172,#73173,#73174,#73175,#73176,
#73177,#73178,#73179,#73180,#73181,#73182,#73183,#73184,#73185,#73186,#73187,
#73188,#73189,#73190,#73191,#73192,#73193,#73194,#73195,#73196,#73197,#73198,
#73199,#73200,#73201,#73202,#73203,#73204,#73205,#73206,#73207,#73208,#73209,
#73210,#73211,#73212,#73213,#73214,#73215,#73216,#73217,#73218,#73219,#73220,
#73221,#73222,#73223,#73224,#73225,#73226,#73227,#73228,#73229,#73230,#73231,
#73232,#73233,#73234,#73235,#73236,#73237,#73238,#73239,#73240,#73241,#73242,
#73243,#73244,#73245,#73246),.UNSPECIFIED.,.F.,.F.,(4,3,3,3,3,3,3,3,3,3,
3,3,3,3,3,3,3,3,3,3,3,3,3,3,3,3,3,3,3,3,3,3,4),(53.4070751110912,53.4842508434172,
53.5614165780464,53.638587389558,53.7157587866332,53.7929466274777,53.8091737269719,
53.8866657594011,53.9641435077811,54.0416125520584,54.119087803636,54.1965627684987,
54.2740542985434,54.3080385389992,54.3855305714285,54.4630083198084,54.5404773640861,
54.6179526156636,54.6954275805259,54.7729191105704,54.8069033510266,54.884395383456,
54.9618731318356,55.0393421761127,55.1168174276899,55.1942923925525,55.2717839225971,
55.3057681630539,55.3832595234145,55.4607387422742,55.5382077764871,55.6156767556165,
55.6324228066038),.UNSPECIFIED.);
#581=B_SPLINE_CURVE_WITH_KNOTS('',3,(#73247,#73248,#73249,#73250,#73251,
#73252,#73253,#73254,#73255,#73256,#73257,#73258,#73259,#73260,#73261,#73262,
#73263,#73264,#73265,#73266,#73267,#73268,#73269,#73270,#73271,#73272,#73273,
#73274,#73275,#73276,#73277,#73278,#73279,#73280,#73281,#73282,#73283,#73284,
#73285,#73286,#73287,#73288,#73289,#73290,#73291,#73292,#73293,#73294,#73295,
#73296,#73297,#73298,#73299,#73300,#73301,#73302,#73303,#73304,#73305,#73306,
#73307,#73308,#73309,#73310,#73311,#73312,#73313,#73314,#73315,#73316,#73317,
#73318,#73319,#73320,#73321,#73322,#73323,#73324,#73325,#73326,#73327,#73328,
#73329,#73330,#73331,#73332,#73333,#73334,#73335,#73336,#73337,#73338,#73339,
#73340,#73341,#73342,#73343,#73344,#73345,#73346,#73347,#73348,#73349,#73350,
#73351,#73352,#73353,#73354,#73355,#73356,#73357,#73358,#73359,#73360,#73361,
#73362,#73363,#73364,#73365,#73366,#73367,#73368,#73369,#73370,#73371,#73372,
#73373,#73374,#73375,#73376,#73377,#73378,#73379,#73380,#73381,#73382,#73383,
#73384,#73385,#73386,#73387,#73388,#73389,#73390,#73391,#73392,#73393,#73394,
#73395,#73396,#73397,#73398,#73399,#73400,#73401,#73402,#73403,#73404,#73405,
#73406,#73407,#73408,#73409,#73410,#73411,#73412,#73413,#73414,#73415,#73416,
#73417,#73418),.UNSPECIFIED.,.F.,.F.,(4,3,3,3,3,3,3,3,3,3,3,3,3,3,3,3,3,
3,3,3,3,3,3,3,3,3,3,3,3,3,3,3,3,3,3,3,3,3,3,3,3,3,3,3,3,3,3,3,3,3,3,3,3,
3,3,3,3,4),(49.3492586328116,49.4267444987807,49.5042182319584,49.5827274816571,
49.6602019486695,49.7392285897114,49.8182552307533,49.8957472631825,49.9732250115623,
50.0506940558395,50.128169307417,50.2056442722796,50.2831358023243,50.3171200427806,
50.3946120752099,50.4720898235896,50.5495588678669,50.6270341194443,50.704509084307,
50.7820006143517,50.8159848548079,50.8934768872372,50.970954635617,51.0484236798943,
51.1258989314718,51.2033738963344,51.2808654263791,51.3148496668353,51.3923416992646,
51.4698194476443,51.5472884919217,51.6247637434991,51.7022387083619,51.7797302384065,
51.8137144788626,51.8912065112918,51.9686842596716,52.0461533039487,52.1236285555262,
52.2011035203887,52.2785950504333,52.3125792908899,52.3900713233191,52.467549071699,
52.5450181159764,52.6224933675538,52.6999683324166,52.7774598624612,52.8114441029172,
52.8889361353464,52.966413883726,53.043882928003,53.1213581795804,53.198833144443,
53.2763246744876,53.3103089149446,53.3927667121797,53.4070751110265),
 .UNSPECIFIED.);
#582=B_SPLINE_CURVE_WITH_KNOTS('',3,(#73424,#73425,#73426,#73427,#73428,
#73429,#73430,#73431,#73432,#73433,#73434,#73435,#73436,#73437,#73438,#73439,
#73440,#73441,#73442,#73443,#73444,#73445,#73446,#73447,#73448,#73449,#73450,
#73451,#73452,#73453,#73454,#73455,#73456,#73457,#73458,#73459,#73460,#73461,
#73462,#73463,#73464,#73465,#73466,#73467,#73468,#73469,#73470,#73471,#73472,
#73473,#73474,#73475,#73476,#73477,#73478,#73479,#73480,#73481,#73482,#73483,
#73484,#73485,#73486,#73487,#73488,#73489,#73490,#73491,#73492,#73493,#73494,
#73495,#73496,#73497,#73498,#73499,#73500,#73501,#73502,#73503,#73504,#73505,
#73506,#73507,#73508,#73509,#73510,#73511,#73512,#73513,#73514,#73515,#73516,
#73517,#73518,#73519,#73520,#73521,#73522,#73523,#73524,#73525,#73526,#73527,
#73528,#73529,#73530,#73531,#73532,#73533,#73534,#73535,#73536,#73537,#73538,
#73539,#73540,#73541,#73542,#73543,#73544,#73545,#73546,#73547,#73548,#73549,
#73550,#73551,#73552,#73553,#73554,#73555,#73556,#73557,#73558,#73559,#73560,
#73561,#73562,#73563,#73564,#73565,#73566,#73567,#73568,#73569,#73570,#73571,
#73572,#73573,#73574,#73575,#73576,#73577,#73578,#73579,#73580,#73581,#73582,
#73583,#73584,#73585,#73586,#73587,#73588,#73589,#73590,#73591,#73592,#73593,
#73594,#73595),.UNSPECIFIED.,.F.,.F.,(4,3,3,3,3,3,3,3,3,3,3,3,3,3,3,3,3,
3,3,3,3,3,3,3,3,3,3,3,3,3,3,3,3,3,3,3,3,3,3,3,3,3,3,3,3,3,3,3,3,3,3,3,3,
3,3,3,3,4),(43.066058970899,43.1435333918981,43.2210263208101,43.28339097146,
43.3608830038894,43.4383607522689,43.5158297965461,43.5933050481236,43.6707800129862,
43.7482715430309,43.7822557834873,43.8597478159166,43.9372255642961,44.0146946085731,
44.0921698601506,44.1696448250135,44.247136355058,44.2811205955147,44.3586126279439,
44.4360903763234,44.5135594206003,44.5910346721779,44.6685096370401,44.7460011670846,
44.779985407542,44.8574774399711,44.934955188351,45.0124242326282,45.0898994842056,
45.1673744490675,45.2448659791124,45.2788502195693,45.3563422519987,45.4338200003786,
45.5112890446562,45.5887642962336,45.6662392610963,45.7437307911408,45.7777150315967,
45.8552070640259,45.9326848124057,46.010153856683,46.08762910826,46.1651040731226,
46.2425956031668,46.276579843624,46.354071876053,46.4315496244331,46.5090186687113,
46.5864939202887,46.6639688851504,46.7414604151948,46.7754446556513,46.8528264263137,
46.9301963796882,47.0075557276487,47.0849176157589,47.1238898038469),
 .UNSPECIFIED.);
#583=B_SPLINE_CURVE_WITH_KNOTS('',3,(#73596,#73597,#73598,#73599,#73600,
#73601,#73602,#73603,#73604,#73605,#73606,#73607,#73608,#73609,#73610,#73611,
#73612,#73613,#73614,#73615,#73616,#73617,#73618,#73619,#73620,#73621,#73622,
#73623,#73624,#73625,#73626,#73627,#73628,#73629,#73630,#73631,#73632,#73633,
#73634,#73635,#73636,#73637,#73638,#73639,#73640,#73641,#73642,#73643,#73644,
#73645,#73646,#73647,#73648,#73649,#73650,#73651,#73652,#73653,#73654,#73655,
#73656,#73657,#73658,#73659,#73660,#73661,#73662,#73663,#73664,#73665,#73666,
#73667,#73668,#73669,#73670,#73671,#73672,#73673,#73674,#73675,#73676,#73677,
#73678,#73679,#73680,#73681,#73682,#73683,#73684,#73685,#73686,#73687,#73688,
#73689),.UNSPECIFIED.,.F.,.F.,(4,3,3,3,3,3,3,3,3,3,3,3,3,3,3,3,3,3,3,3,
3,3,3,3,3,3,3,3,3,3,3,4),(47.1238898039682,47.2045406527714,47.2743094676786,
47.3518015001079,47.4292792484876,47.5067482927648,47.5842235443423,47.661698509205,
47.7391900392496,47.773174279706,47.8506663121353,47.928144060515,48.005613104792,
48.0830883563694,48.1605633212322,48.2380548512768,48.2720390917333,48.3495311241625,
48.4270088725422,48.5044779168194,48.5819531683968,48.6594281332595,48.7369196633042,
48.7709039037606,48.8483959361898,48.9258736845696,49.0033427288469,49.0808179804244,
49.158292945287,49.2357844753317,49.269768715788,49.3492660090855),
 .UNSPECIFIED.);
#584=B_SPLINE_CURVE_WITH_KNOTS('',3,(#73691,#73692,#73693,#73694,#73695,
#73696,#73697,#73698,#73699,#73700,#73701,#73702,#73703,#73704,#73705,#73706,
#73707,#73708,#73709,#73710,#73711,#73712,#73713,#73714,#73715,#73716,#73717,
#73718,#73719,#73720,#73721,#73722,#73723,#73724,#73725,#73726,#73727,#73728,
#73729,#73730,#73731,#73732,#73733,#73734,#73735,#73736,#73737,#73738,#73739,
#73740,#73741,#73742,#73743,#73744,#73745,#73746,#73747,#73748,#73749,#73750,
#73751,#73752,#73753,#73754,#73755,#73756,#73757,#73758,#73759,#73760,#73761,
#73762,#73763,#73764,#73765,#73766,#73767,#73768,#73769,#73770,#73771,#73772,
#73773,#73774,#73775,#73776,#73777,#73778,#73779,#73780,#73781,#73782,#73783,
#73784,#73785,#73786,#73787),.UNSPECIFIED.,.F.,.F.,(4,3,3,3,3,3,3,3,3,3,
3,3,3,3,3,3,3,3,3,3,3,3,3,3,3,3,3,3,3,3,3,3,4),(47.1238898039176,47.2032584038848,
47.2826529753093,47.3239311706166,47.4014232030459,47.4789009514257,47.5563699957031,
47.6338452472805,47.7113202121431,47.7888117421879,47.8227959826439,47.9002880150732,
47.9777657634529,48.05523480773,48.1327100593075,48.2101850241701,48.2876765542147,
48.3216607946713,48.3991528271006,48.4766305754802,48.5540996197574,48.6315748713349,
48.7090498361976,48.7865413662423,48.8205256066986,48.8980176391279,48.9754953875076,
49.0529644317848,49.1304396833623,49.207914648225,49.2854061782696,49.3193904187259,
49.3492586328116),.UNSPECIFIED.);
#585=B_SPLINE_CURVE_WITH_KNOTS('',3,(#73788,#73789,#73790,#73791,#73792,
#73793,#73794,#73795,#73796,#73797,#73798,#73799,#73800,#73801,#73802,#73803,
#73804,#73805,#73806,#73807,#73808,#73809,#73810,#73811,#73812,#73813,#73814,
#73815,#73816,#73817,#73818,#73819,#73820,#73821,#73822,#73823,#73824,#73825,
#73826,#73827,#73828,#73829,#73830,#73831,#73832,#73833,#73834,#73835,#73836,
#73837,#73838,#73839,#73840,#73841,#73842,#73843,#73844,#73845,#73846,#73847,
#73848,#73849,#73850,#73851,#73852,#73853,#73854,#73855,#73856,#73857,#73858,
#73859,#73860,#73861,#73862,#73863,#73864,#73865,#73866,#73867,#73868,#73869,
#73870,#73871,#73872,#73873,#73874,#73875,#73876,#73877,#73878,#73879,#73880,
#73881,#73882,#73883,#73884,#73885,#73886,#73887,#73888,#73889,#73890,#73891,
#73892,#73893,#73894,#73895,#73896,#73897,#73898,#73899,#73900,#73901,#73902,
#73903,#73904,#73905,#73906,#73907,#73908,#73909,#73910,#73911,#73912,#73913,
#73914,#73915,#73916,#73917,#73918,#73919,#73920,#73921,#73922,#73923,#73924,
#73925,#73926,#73927,#73928,#73929,#73930,#73931,#73932,#73933,#73934,#73935,
#73936,#73937,#73938,#73939,#73940,#73941,#73942,#73943,#73944,#73945,#73946,
#73947,#73948,#73949,#73950,#73951,#73952,#73953,#73954,#73955,#73956,#73957,
#73958,#73959),.UNSPECIFIED.,.F.,.F.,(4,3,3,3,3,3,3,3,3,3,3,3,3,3,3,3,3,
3,3,3,3,3,3,3,3,3,3,3,3,3,3,3,3,3,3,3,3,3,3,3,3,3,3,3,3,3,3,3,3,3,3,3,3,
3,3,3,3,4),(43.0660676533433,43.143542925694,43.2210178738762,43.2985094186679,
43.333012674398,43.4105047068272,43.4879824552068,43.5654514994841,43.6429267510615,
43.720401715924,43.7978932459686,43.8318774864253,43.9093695188546,43.9868472672343,
44.0643163115116,44.1417915630891,44.2192665279518,44.2967580579965,44.3307422984526,
44.4082343308818,44.4857120792616,44.5631811235388,44.6406563751163,44.718131339979,
44.7956228700236,44.82960711048,44.9070991429092,44.984576891289,45.0620459355663,
45.1395211871438,45.2169961520065,45.2944876820511,45.3284719225073,45.4059639549365,
45.4834417033163,45.5609107475936,45.6383859991711,45.7158609640337,45.7933524940783,
45.8273367345346,45.9048287669638,45.9823065153436,46.0597755596211,46.1372508111986,
46.2147257760612,46.2922173061059,46.326201546562,46.4036935789912,46.481171327371,
46.5586403716484,46.6361156232258,46.7135905880888,46.7910821181334,46.8250663585893,
46.9028676038855,46.9806524488782,47.058431481866,47.1238898038469),
 .UNSPECIFIED.);
#586=B_SPLINE_CURVE_WITH_KNOTS('',3,(#73965,#73966,#73967,#73968,#73969,
#73970,#73971,#73972,#73973,#73974,#73975,#73976,#73977),.UNSPECIFIED.,
 .F.,.F.,(4,1,1,1,1,1,1,1,1,1,4),(36.7828738679604,36.7981484151047,37.2970132271321,
37.7958780391594,38.2947428511867,38.793607663214,39.2924724752414,39.7913372872687,
40.290202099296,40.7890669113234,40.8407044966673),.UNSPECIFIED.);
#587=B_SPLINE_CURVE_WITH_KNOTS('',3,(#73978,#73979,#73980,#73981,#73982,
#73983,#73984,#73985,#73986,#73987,#73988,#73989,#73990,#73991,#73992,#73993,
#73994,#73995,#73996,#73997,#73998,#73999,#74000,#74001,#74002,#74003,#74004,
#74005,#74006,#74007,#74008,#74009,#74010,#74011,#74012,#74013,#74014,#74015,
#74016,#74017,#74018,#74019,#74020,#74021,#74022,#74023,#74024,#74025,#74026,
#74027,#74028,#74029,#74030,#74031,#74032,#74033,#74034,#74035,#74036,#74037,
#74038,#74039,#74040,#74041,#74042,#74043,#74044,#74045,#74046,#74047,#74048,
#74049,#74050,#74051,#74052,#74053,#74054,#74055,#74056,#74057,#74058,#74059,
#74060,#74061,#74062,#74063,#74064,#74065,#74066,#74067,#74068,#74069,#74070,
#74071),.UNSPECIFIED.,.F.,.F.,(4,3,3,3,3,3,3,3,3,3,3,3,3,3,3,3,3,3,3,3,
3,3,3,3,3,3,3,3,3,3,3,4),(40.8407044966673,40.9179251802868,40.995132453893,
41.0723426888697,41.149549938454,41.2267761550704,41.2879317233507,41.36542375578,
41.4429015041596,41.5203705484367,41.5978458000141,41.6753207648766,41.7528122949213,
41.786796535378,41.8642885678073,41.9417663161871,42.0192353604645,42.0967106120418,
42.1741855769045,42.2516771069493,42.2856613474054,42.3631533798346,42.4406311282143,
42.5181001724917,42.5955754240691,42.673050388932,42.7505419189767,42.7845261594327,
42.8620191530837,42.9394967034995,43.0169700726562,43.066058970899),
 .UNSPECIFIED.);
#588=B_SPLINE_CURVE_WITH_KNOTS('',3,(#74073,#74074,#74075,#74076,#74077,
#74078,#74079,#74080,#74081,#74082,#74083,#74084,#74085,#74086,#74087,#74088,
#74089,#74090,#74091,#74092,#74093,#74094,#74095,#74096,#74097,#74098,#74099,
#74100,#74101,#74102,#74103,#74104,#74105,#74106,#74107,#74108,#74109,#74110,
#74111,#74112,#74113,#74114,#74115,#74116,#74117,#74118,#74119,#74120,#74121,
#74122,#74123,#74124,#74125,#74126,#74127,#74128,#74129,#74130,#74131,#74132,
#74133,#74134,#74135,#74136,#74137,#74138,#74139,#74140,#74141,#74142,#74143,
#74144,#74145,#74146,#74147,#74148,#74149,#74150,#74151,#74152,#74153,#74154,
#74155,#74156,#74157,#74158,#74159,#74160,#74161,#74162,#74163,#74164,#74165,
#74166),.UNSPECIFIED.,.F.,.F.,(4,3,3,3,3,3,3,3,3,3,3,3,3,3,3,3,3,3,3,3,
3,3,3,3,3,3,3,3,3,3,3,4),(40.8407044966673,40.9181815167146,40.9956442072441,
41.073098197011,41.1505583692719,41.2280183712181,41.3054948721939,41.3375534262887,
41.415045458718,41.4925232070977,41.5699922513747,41.6474675029522,41.7249424678148,
41.8024339978594,41.836418238316,41.9139102707452,41.991388019125,42.0688570634023,
42.1463323149798,42.2238072798424,42.3012988098871,42.3352830503433,42.4127750827726,
42.4902528311523,42.5677218754295,42.6451971270069,42.7226720918697,42.8001636219143,
42.8341478623707,42.9116395331415,42.9891221306656,43.0660676533433),
 .UNSPECIFIED.);
#589=B_SPLINE_CURVE_WITH_KNOTS('',3,(#74167,#74168,#74169,#74170,#74171,
#74172,#74173,#74174,#74175,#74176,#74177,#74178,#74179,#74180,#74181,#74182,
#74183,#74184,#74185,#74186,#74187,#74188,#74189,#74190,#74191,#74192,#74193,
#74194,#74195,#74196,#74197,#74198,#74199,#74200,#74201,#74202,#74203,#74204,
#74205,#74206,#74207,#74208,#74209,#74210,#74211,#74212,#74213,#74214,#74215,
#74216,#74217,#74218,#74219,#74220,#74221,#74222,#74223,#74224,#74225,#74226,
#74227,#74228,#74229,#74230,#74231,#74232,#74233,#74234,#74235,#74236,#74237,
#74238,#74239,#74240,#74241,#74242,#74243,#74244,#74245,#74246,#74247,#74248,
#74249,#74250,#74251,#74252,#74253,#74254,#74255,#74256,#74257,#74258,#74259,
#74260,#74261,#74262,#74263,#74264,#74265,#74266,#74267,#74268,#74269,#74270,
#74271,#74272,#74273,#74274,#74275,#74276,#74277,#74278,#74279,#74280,#74281,
#74282,#74283,#74284,#74285,#74286,#74287,#74288,#74289,#74290,#74291,#74292,
#74293,#74294,#74295,#74296,#74297,#74298,#74299,#74300,#74301,#74302,#74303,
#74304,#74305,#74306,#74307,#74308,#74309,#74310,#74311,#74312,#74313,#74314,
#74315,#74316,#74317,#74318,#74319,#74320,#74321,#74322,#74323,#74324,#74325,
#74326,#74327,#74328,#74329,#74330,#74331,#74332,#74333,#74334,#74335,#74336,
#74337,#74338,#74339,#74340,#74341),.UNSPECIFIED.,.F.,.F.,(4,3,3,3,3,3,
3,3,3,3,3,3,3,3,3,3,3,3,3,3,3,3,3,3,3,3,3,3,3,3,3,3,3,3,3,3,3,3,3,3,3,3,
3,3,3,3,3,3,3,3,3,3,3,3,3,3,3,3,4),(36.782864454183,36.8477701180427,36.925262150472,
37.0027398988517,37.0802089431291,37.1576841947065,37.235159159569,37.3126506896138,
37.34663493007,37.4241269624992,37.501604710879,37.5790737551564,37.6565490067337,
37.7340239715966,37.8115155016411,37.8454997420974,37.9229917745268,38.0004695229064,
38.0779385671842,38.1554138187617,38.2328887836243,38.310380313669,38.3443645541247,
38.4218565865539,38.499334334934,38.5768033792115,38.6542786307892,38.7317535956524,
38.8092451256973,38.843229366152,38.9207213985812,38.998199146961,39.0756681912389,
39.1531434428164,39.2306184076787,39.3081099377237,39.3420941781794,39.4195862106086,
39.4970639589884,39.5745330032661,39.6520082548436,39.7294832197065,39.8069747497514,
39.8409589902067,39.9184510226361,39.9959287710154,40.0733978152927,40.1508730668702,
40.2283480317326,40.3058395617773,40.339823802234,40.4173158346631,40.4947935830427,
40.5722626273201,40.6497378788975,40.7272128437605,40.8047043738045,40.8386886142613,
40.8407044964987),.UNSPECIFIED.);
#590=B_SPLINE_CURVE_WITH_KNOTS('',3,(#74347,#74348,#74349,#74350,#74351,
#74352,#74353,#74354,#74355,#74356,#74357,#74358,#74359,#74360,#74361,#74362,
#74363,#74364,#74365,#74366,#74367,#74368,#74369,#74370,#74371,#74372,#74373,
#74374,#74375,#74376,#74377,#74378,#74379,#74380,#74381,#74382,#74383,#74384,
#74385,#74386,#74387,#74388,#74389,#74390,#74391,#74392,#74393,#74394,#74395,
#74396,#74397,#74398,#74399,#74400,#74401,#74402,#74403,#74404,#74405,#74406,
#74407,#74408,#74409,#74410,#74411,#74412,#74413,#74414,#74415,#74416,#74417,
#74418,#74419,#74420,#74421,#74422,#74423,#74424,#74425,#74426,#74427,#74428,
#74429,#74430,#74431,#74432,#74433,#74434,#74435,#74436,#74437,#74438,#74439,
#74440,#74441,#74442,#74443,#74444,#74445,#74446,#74447,#74448,#74449,#74450,
#74451,#74452,#74453,#74454,#74455,#74456,#74457,#74458,#74459,#74460,#74461,
#74462,#74463,#74464,#74465,#74466,#74467,#74468,#74469,#74470,#74471,#74472,
#74473,#74474,#74475,#74476,#74477,#74478,#74479,#74480,#74481,#74482,#74483,
#74484,#74485,#74486,#74487,#74488,#74489,#74490,#74491,#74492,#74493,#74494,
#74495,#74496,#74497,#74498,#74499,#74500,#74501,#74502,#74503,#74504,#74505,
#74506,#74507,#74508,#74509,#74510,#74511,#74512,#74513,#74514,#74515,#74516,
#74517,#74518),.UNSPECIFIED.,.F.,.F.,(4,3,3,3,3,3,3,3,3,3,3,3,3,3,3,3,3,
3,3,3,3,3,3,3,3,3,3,3,3,3,3,3,3,3,3,3,3,3,3,3,3,3,3,3,3,3,3,3,3,3,3,3,3,
3,3,3,3,4),(30.4997043503953,30.5777209304906,30.6551953822583,30.7334830265175,
30.8117706707768,30.889262703206,30.9667404515857,31.0442094958629,31.1216847474403,
31.1991597123029,31.2766512423475,31.3106354828041,31.3881275152334,31.4656052636131,
31.5430743078904,31.6205495594679,31.6980245243305,31.7755160543752,31.8095002948314,
31.8869923272607,31.9644700756404,32.0419391199176,32.1194143714951,32.1968893363578,
32.2743808664024,32.3083651068588,32.385857139288,32.4633348876678,32.5408039319451,
32.6182791835225,32.6957541483852,32.7732456784298,32.8072299188861,32.8847219513153,
32.9621996996951,33.0396687439724,33.1171439955498,33.1946189604125,33.2721104904572,
33.3060947309134,33.3835867633426,33.4610645117224,33.5385335559996,33.6160088075771,
33.6934837724398,33.7709753024844,33.8049595429408,33.8824515753701,33.9599293237497,
34.0373983680268,34.1148736196042,34.1923485844669,34.2698401145116,34.3038243549681,
34.3822177070359,34.4605943978029,34.5389569593193,34.5575191894877),
 .UNSPECIFIED.);
#591=B_SPLINE_CURVE_WITH_KNOTS('',3,(#74519,#74520,#74521,#74522,#74523,
#74524,#74525,#74526),.UNSPECIFIED.,.F.,.F.,(4,1,1,1,1,4),(34.5575191926081,
34.8026891669954,35.3015539790227,35.8004187910501,36.2992836030774,36.7828738679604),
 .UNSPECIFIED.);
#592=B_SPLINE_CURVE_WITH_KNOTS('',3,(#74528,#74529,#74530,#74531,#74532,
#74533,#74534,#74535,#74536,#74537,#74538,#74539,#74540,#74541,#74542,#74543,
#74544,#74545,#74546,#74547,#74548,#74549,#74550,#74551,#74552,#74553,#74554,
#74555,#74556,#74557,#74558,#74559,#74560,#74561,#74562,#74563,#74564,#74565,
#74566,#74567,#74568,#74569,#74570,#74571,#74572,#74573,#74574,#74575,#74576,
#74577,#74578,#74579,#74580,#74581,#74582,#74583,#74584,#74585,#74586,#74587,
#74588,#74589,#74590,#74591,#74592,#74593,#74594,#74595,#74596,#74597,#74598,
#74599,#74600,#74601,#74602,#74603,#74604,#74605,#74606,#74607,#74608,#74609,
#74610,#74611,#74612,#74613,#74614,#74615,#74616,#74617,#74618,#74619,#74620,
#74621),.UNSPECIFIED.,.F.,.F.,(4,3,3,3,3,3,3,3,3,3,3,3,3,3,3,3,3,3,3,3,
3,3,3,3,3,3,3,3,3,3,3,4),(34.5575191894877,34.6353433852827,34.7131680802738,
34.7910131120779,34.8523108699334,34.9298029023626,35.0072806507426,35.0847496950204,
35.1622249465979,35.2396999114606,35.3171914415054,35.3511756819607,35.4286677143899,
35.5061454627699,35.5836145070471,35.6610897586247,35.7385647234876,35.8160562535323,
35.8500404939881,35.9275325264173,36.0050102747971,36.0824793190741,36.1599545706517,
36.2374295355144,36.314921065559,36.3489053060154,36.4263967590605,36.5038736983943,
36.5813489641976,36.6588188367758,36.7362996359494,36.782864454183),
 .UNSPECIFIED.);
#593=B_SPLINE_CURVE_WITH_KNOTS('',3,(#74622,#74623,#74624,#74625,#74626,
#74627,#74628,#74629,#74630,#74631,#74632,#74633,#74634,#74635,#74636,#74637,
#74638,#74639,#74640,#74641,#74642,#74643,#74644,#74645,#74646,#74647,#74648,
#74649,#74650,#74651,#74652,#74653,#74654,#74655,#74656,#74657,#74658,#74659,
#74660,#74661,#74662,#74663,#74664,#74665,#74666,#74667,#74668,#74669,#74670,
#74671,#74672,#74673,#74674,#74675,#74676,#74677,#74678,#74679,#74680,#74681,
#74682,#74683,#74684,#74685,#74686,#74687,#74688,#74689,#74690,#74691,#74692,
#74693,#74694,#74695,#74696,#74697,#74698,#74699,#74700,#74701,#74702,#74703,
#74704,#74705,#74706,#74707,#74708,#74709,#74710,#74711,#74712,#74713,#74714,
#74715,#74716,#74717,#74718,#74719,#74720,#74721,#74722,#74723,#74724,#74725,
#74726,#74727,#74728,#74729,#74730,#74731,#74732,#74733,#74734,#74735,#74736,
#74737,#74738,#74739,#74740,#74741,#74742,#74743,#74744,#74745,#74746,#74747,
#74748,#74749,#74750,#74751,#74752,#74753,#74754,#74755,#74756,#74757,#74758,
#74759,#74760,#74761,#74762,#74763,#74764,#74765,#74766,#74767,#74768,#74769,
#74770,#74771,#74772,#74773,#74774,#74775,#74776,#74777,#74778,#74779,#74780,
#74781,#74782,#74783,#74784,#74785,#74786,#74787,#74788,#74789,#74790,#74791,
#74792,#74793),.UNSPECIFIED.,.F.,.F.,(4,3,3,3,3,3,3,3,3,3,3,3,3,3,3,3,3,
3,3,3,3,3,3,3,3,3,3,3,3,3,3,3,3,3,3,3,3,3,3,3,3,3,3,3,3,3,3,3,3,3,3,3,3,
3,3,3,3,4),(30.4997098142701,30.5771803637444,30.6546564701863,30.732131006469,
30.8096232719206,30.8613923737148,30.9388844061442,31.016362154524,31.0938311988014,
31.1713064503789,31.2487814152417,31.3262729452865,31.3602571857421,31.4377492181713,
31.5152269665509,31.5926960108281,31.6701712624054,31.747646227268,31.8251377573126,
31.8591219977694,31.9366140301987,32.0140917785784,32.0915608228557,32.1690360744331,
32.2465110392958,32.3240025693406,32.3579868097967,32.4354788422259,32.5129565906057,
32.590425634883,32.6679008864605,32.7453758513231,32.8228673813677,32.8568516218241,
32.9343436542533,33.0118214026331,33.0892904469103,33.1667656984877,33.2442406633505,
33.3217321933952,33.3557164338514,33.4332084662806,33.5106862146603,33.5881552589374,
33.6656305105148,33.7431054753776,33.8205970054223,33.8545812458787,33.9320732783079,
34.0095510266875,34.0870200709647,34.1644953225422,34.2419702874047,34.3194618174493,
34.3534460579061,34.4327535366758,34.5120401040698,34.5575191894205),
 .UNSPECIFIED.);
#594=B_SPLINE_CURVE_WITH_KNOTS('',3,(#74799,#74800,#74801,#74802,#74803,
#74804,#74805,#74806,#74807,#74808,#74809,#74810),.UNSPECIFIED.,.F.,.F.,
(4,1,1,1,1,1,1,1,1,4),(24.2164828558523,24.3265281144215,24.8253929264488,
25.3242577384762,25.8231225505035,26.3219873625308,26.8208521745581,27.3197169865855,
27.8185817986128,28.2743338450134),.UNSPECIFIED.);
#595=B_SPLINE_CURVE_WITH_KNOTS('',3,(#74811,#74812,#74813,#74814,#74815,
#74816,#74817,#74818,#74819,#74820,#74821,#74822,#74823,#74824,#74825,#74826,
#74827,#74828,#74829,#74830,#74831,#74832,#74833,#74834,#74835,#74836,#74837,
#74838,#74839,#74840,#74841,#74842,#74843,#74844,#74845,#74846,#74847,#74848,
#74849,#74850,#74851,#74852,#74853,#74854,#74855,#74856,#74857,#74858,#74859,
#74860,#74861,#74862,#74863,#74864,#74865,#74866,#74867,#74868,#74869,#74870,
#74871,#74872,#74873,#74874,#74875,#74876,#74877,#74878,#74879,#74880,#74881,
#74882,#74883,#74884,#74885,#74886,#74887,#74888,#74889,#74890,#74891,#74892,
#74893,#74894,#74895,#74896,#74897,#74898,#74899,#74900,#74901,#74902,#74903,
#74904,#74905,#74906,#74907),.UNSPECIFIED.,.F.,.F.,(4,3,3,3,3,3,3,3,3,3,
3,3,3,3,3,3,3,3,3,3,3,3,3,3,3,3,3,3,3,3,3,3,4),(28.2743338823081,28.3174466106401,
28.3949386430695,28.4724163914493,28.5498854357268,28.6273606873043,28.7048356521673,
28.7823271822121,28.8163114226675,28.8938034550967,28.9712812034763,29.0487502477537,
29.1262254993311,29.2037004641937,29.2811919942383,29.3151762346948,29.3926682671241,
29.4701460155037,29.547615059781,29.6250903113584,29.7025652762211,29.7800568062657,
29.8140410467221,29.8915330791514,29.969010827531,30.0464798718082,30.1239551233857,
30.2014300882484,30.2789216182931,30.3129058587495,30.3903971270004,30.4678751330957,
30.4997043503953),.UNSPECIFIED.);
#596=B_SPLINE_CURVE_WITH_KNOTS('',3,(#74909,#74910,#74911,#74912,#74913,
#74914,#74915,#74916,#74917,#74918,#74919,#74920,#74921,#74922,#74923,#74924,
#74925,#74926,#74927,#74928,#74929,#74930,#74931,#74932,#74933,#74934,#74935,
#74936,#74937,#74938,#74939,#74940,#74941,#74942,#74943,#74944,#74945,#74946,
#74947,#74948,#74949,#74950,#74951,#74952,#74953,#74954,#74955,#74956,#74957,
#74958,#74959,#74960,#74961,#74962,#74963,#74964,#74965,#74966,#74967,#74968,
#74969,#74970,#74971,#74972,#74973,#74974,#74975,#74976,#74977,#74978,#74979,
#74980,#74981,#74982,#74983,#74984,#74985,#74986,#74987,#74988,#74989,#74990,
#74991,#74992,#74993,#74994,#74995,#74996,#74997,#74998,#74999,#75000,#75001,
#75002,#75003,#75004,#75005),.UNSPECIFIED.,.F.,.F.,(4,3,3,3,3,3,3,3,3,3,
3,3,3,3,3,3,3,3,3,3,3,3,3,3,3,3,3,3,3,3,3,3,4),(28.2743338823081,28.3569496379083,
28.3670683135781,28.4445603460099,28.5220380943922,28.5995071386723,28.6769823902524,
28.7544573551178,28.8319488851651,28.8659331256054,28.9434251580338,29.0209029064128,
29.098371950689,29.1758472022655,29.2533221671273,29.3308136971711,29.3647979376328,
29.4422899700621,29.5197677184421,29.5972367627195,29.674712014297,29.7521869791598,
29.8296785092045,29.8636627496601,29.9411547820895,30.0186325304694,30.0961015747468,
30.1735768263243,30.2510517911872,30.328543321232,30.3625275616874,30.4400203072111,
30.4997098142701),.UNSPECIFIED.);
#597=B_SPLINE_CURVE_WITH_KNOTS('',3,(#75006,#75007,#75008,#75009,#75010,
#75011,#75012,#75013,#75014,#75015,#75016,#75017,#75018,#75019,#75020,#75021,
#75022,#75023,#75024,#75025,#75026,#75027,#75028,#75029,#75030,#75031,#75032,
#75033,#75034,#75035,#75036,#75037,#75038,#75039,#75040,#75041,#75042,#75043,
#75044,#75045,#75046,#75047,#75048,#75049,#75050,#75051,#75052,#75053,#75054,
#75055,#75056,#75057,#75058,#75059,#75060,#75061,#75062,#75063,#75064,#75065,
#75066,#75067,#75068,#75069,#75070,#75071,#75072,#75073,#75074,#75075,#75076,
#75077,#75078,#75079,#75080,#75081,#75082,#75083,#75084,#75085,#75086,#75087,
#75088,#75089,#75090,#75091,#75092,#75093,#75094,#75095,#75096,#75097,#75098,
#75099,#75100,#75101,#75102,#75103,#75104,#75105,#75106,#75107,#75108,#75109,
#75110,#75111,#75112,#75113,#75114,#75115,#75116,#75117,#75118,#75119,#75120,
#75121,#75122,#75123,#75124,#75125,#75126,#75127,#75128,#75129,#75130,#75131,
#75132,#75133,#75134,#75135,#75136,#75137,#75138,#75139,#75140,#75141,#75142,
#75143,#75144,#75145,#75146,#75147,#75148,#75149,#75150,#75151,#75152,#75153,
#75154,#75155,#75156,#75157,#75158,#75159,#75160,#75161,#75162,#75163,#75164,
#75165,#75166,#75167,#75168,#75169,#75170,#75171,#75172,#75173,#75174,#75175,
#75176,#75177),.UNSPECIFIED.,.F.,.F.,(4,3,3,3,3,3,3,3,3,3,3,3,3,3,3,3,3,
3,3,3,3,3,3,3,3,3,3,3,3,3,3,3,3,3,3,3,3,3,3,3,3,3,3,3,3,3,3,3,3,3,3,3,3,
3,3,3,3,4),(24.2164947951915,24.2963223062755,24.3761498173595,24.4536418492143,
24.5311195970121,24.6085886407024,24.6860638916884,24.7635388559585,24.8410303854126,
24.8750146293868,24.9525066621344,25.0299844108363,25.1074534554392,25.1849287073434,
25.2624036725332,25.3398952029039,25.3738794414141,25.4513714737075,25.5288492219499,
25.6063182660886,25.6837935175271,25.7612684822504,25.8387600121567,25.8727442534415,
25.9502362859097,26.0277140343293,26.1051830786465,26.1826583302636,26.2601332951656,
26.3376248252496,26.3716090654688,26.4491010978985,26.5265788462786,26.6040478905561,
26.6815231421342,26.7589981069978,26.8364896370432,26.8704738774961,26.9479659099148,
27.0254436582844,27.1029127025519,27.1803879541189,27.2578629189705,27.3353544490048,
27.3693386895235,27.4468307219618,27.5243084703507,27.6017775146373,27.679252766224,
27.756727731096,27.83421926115,27.8682035015508,27.9453872774562,28.0225556395814,
28.0997214532917,28.1768831987141,28.2540554491615,28.2743338822298),
 .UNSPECIFIED.);
#598=B_SPLINE_CURVE_WITH_KNOTS('',3,(#75183,#75184,#75185,#75186,#75187,
#75188,#75189,#75190,#75191),.UNSPECIFIED.,.F.,.F.,(4,1,1,1,1,1,4),(15.7079632679489,
15.8954480128949,16.3943128249222,16.8931776369496,17.3920424489769,17.8909072610042,
17.9333372203403),.UNSPECIFIED.);
#599=B_SPLINE_CURVE_WITH_KNOTS('',3,(#75193,#75194,#75195,#75196,#75197,
#75198),.UNSPECIFIED.,.F.,.F.,(4,1,1,4),(14.3988535768129,14.8977183888402,
15.3965832008676,15.7079632679489),.UNSPECIFIED.);
#600=B_SPLINE_CURVE_WITH_KNOTS('',3,(#75202,#75203,#75204,#75205,#75206,
#75207,#75208),.UNSPECIFIED.,.F.,.F.,(4,1,1,1,4),(13.8754803054952,14.3492318738749,
14.8480966859023,15.3469614979296,15.7079632679489),.UNSPECIFIED.);
#601=B_SPLINE_CURVE_WITH_KNOTS('',3,(#75209,#75210,#75211,#75212,#75213,
#75214,#75215,#75216,#75217),.UNSPECIFIED.,.F.,.F.,(4,1,1,1,1,1,4),(15.7079632679489,
15.8458263099569,16.3446911219842,16.8435559340116,17.3424207460389,17.8412855580662,
17.9333477466581),.UNSPECIFIED.);
#602=B_SPLINE_CURVE_WITH_KNOTS('',3,(#75223,#75224,#75225,#75226,#75227,
#75228,#75229,#75230),.UNSPECIFIED.,.F.,.F.,(4,2,2,4),(-0.249826015691648,
-0.174054989991414,-0.112681174836296,-5.98438861682063E-5),
 .UNSPECIFIED.);
#603=B_SPLINE_CURVE_WITH_KNOTS('',3,(#75233,#75234,#75235,#75236,#75237,
#75238,#75239,#75240,#75241,#75242,#75243,#75244,#75245,#75246,#75247,#75248,
#75249,#75250,#75251,#75252,#75253,#75254,#75255,#75256,#75257,#75258,#75259,
#75260,#75261,#75262,#75263,#75264,#75265,#75266,#75267,#75268,#75269,#75270,
#75271,#75272,#75273,#75274,#75275,#75276),.UNSPECIFIED.,.F.,.F.,(4,2,2,
2,2,2,2,2,2,2,2,2,2,2,2,2,2,2,2,2,2,4),(-6.11671048338158,-5.96153956264804,
-5.84115877786849,-5.80007352684886,-5.76536661656876,-5.67608165850516,
-5.61674511723677,-5.47922466329569,-5.43073195824578,-5.37491543409902,
-5.30049496163558,-5.27011467092952,-5.19890052636434,-5.12206091177934,
-5.10075658906977,-5.06249072850121,-4.97963646160468,-4.90348514082996,
-4.81921126869143,-4.74227675282595,-4.70012783424564,-4.66100346190723),
 .UNSPECIFIED.);
#604=B_SPLINE_CURVE_WITH_KNOTS('',3,(#75281,#75282,#75283,#75284,#75285,
#75286,#75287,#75288,#75289,#75290,#75291,#75292,#75293,#75294,#75295,#75296,
#75297,#75298,#75299,#75300,#75301,#75302,#75303,#75304,#75305,#75306,#75307,
#75308,#75309,#75310,#75311,#75312,#75313,#75314,#75315,#75316,#75317,#75318,
#75319,#75320,#75321,#75322,#75323,#75324,#75325,#75326,#75327,#75328,#75329,
#75330,#75331,#75332,#75333,#75334,#75335,#75336,#75337,#75338,#75339,#75340,
#75341,#75342,#75343,#75344,#75345,#75346,#75347,#75348,#75349,#75350,#75351,
#75352,#75353,#75354,#75355,#75356,#75357,#75358,#75359,#75360,#75361,#75362,
#75363,#75364,#75365,#75366,#75367,#75368,#75369,#75370,#75371,#75372,#75373,
#75374,#75375,#75376,#75377,#75378,#75379,#75380,#75381,#75382,#75383,#75384,
#75385,#75386,#75387,#75388,#75389,#75390,#75391,#75392,#75393,#75394,#75395,
#75396,#75397,#75398,#75399,#75400,#75401,#75402,#75403,#75404),
 .UNSPECIFIED.,.F.,.F.,(4,2,2,2,2,2,2,2,2,2,2,2,2,2,2,2,2,2,2,2,2,2,2,2,
2,2,2,2,2,2,2,2,2,2,2,2,2,2,2,2,2,2,2,2,2,2,2,2,2,2,2,2,2,2,2,2,2,2,2,2,
2,4),(-4.661040529428,-4.59250079239981,-4.5588280390274,-4.51925590365334,
-4.43950198910759,-4.38022384530102,-4.25820358191914,-4.20180510591333,
-4.12533749912705,-4.03567785246762,-3.96195778728872,-3.89280199334527,
-3.8472816427279,-3.77297244856651,-3.68479577805155,-3.54299662275098,
-3.49717304314424,-3.42207112732758,-3.32867078560331,-3.20988293964267,
-3.15147510198992,-3.07331444426717,-2.98453912420175,-2.91189784048555,
-2.81952245029366,-2.78141079113058,-2.69821153880586,-2.62153686814335,
-2.52615111761924,-2.45542875263231,-2.40669530834557,-2.26969074547352,
-2.18194656422033,-2.1068040420648,-2.06129408857846,-1.99216352691328,
-1.91846521303171,-1.82948024871057,-1.75180578992144,-1.69202736926351,
-1.58198232863079,-1.50512564938352,-1.42139742612079,-1.38353349166211,
-1.29151110712416,-1.21814585852054,-1.15910144667136,-1.07820422203281,
-1.03844509860151,-0.999978242961427,-0.872257699284099,-0.841905751085272,
-0.77267566309266,-0.703753678947113,-0.652879246690581,-0.52137716917312,
-0.491309869279923,-0.421533932405962,-0.357554499970899,-0.324129770168331,
-0.273276533780277,-0.249826015691648),.UNSPECIFIED.);
#605=B_SPLINE_CURVE_WITH_KNOTS('',3,(#75405,#75406,#75407,#75408,#75409,
#75410,#75411,#75412,#75413,#75414,#75415,#75416,#75417,#75418,#75419,#75420,
#75421,#75422,#75423,#75424,#75425,#75426,#75427,#75428,#75429,#75430,#75431,
#75432,#75433,#75434,#75435,#75436,#75437,#75438,#75439,#75440,#75441,#75442,
#75443,#75444,#75445,#75446,#75447,#75448,#75449,#75450,#75451,#75452,#75453,
#75454,#75455,#75456,#75457,#75458,#75459,#75460,#75461,#75462,#75463,#75464,
#75465,#75466,#75467,#75468,#75469,#75470,#75471,#75472,#75473,#75474,#75475,
#75476,#75477,#75478,#75479,#75480,#75481,#75482,#75483,#75484,#75485,#75486,
#75487,#75488,#75489,#75490,#75491,#75492,#75493,#75494,#75495,#75496,#75497,
#75498,#75499,#75500,#75501,#75502,#75503,#75504,#75505,#75506,#75507,#75508,
#75509,#75510,#75511,#75512,#75513,#75514,#75515,#75516,#75517,#75518,#75519,
#75520,#75521,#75522,#75523,#75524,#75525,#75526,#75527,#75528),
 .UNSPECIFIED.,.F.,.F.,(4,2,2,2,2,2,2,2,2,2,2,2,2,2,2,2,2,2,2,2,2,2,2,2,
2,2,2,2,2,2,2,2,2,2,2,2,2,2,2,2,2,2,2,2,2,2,2,2,2,2,2,2,2,2,2,2,2,2,2,2,
2,4),(-4.66100346190723,-4.62037419810526,-4.5611047479869,-4.43901396909629,
-4.38266566505239,-4.30620877569181,-4.21653926920206,-4.14280707990123,
-4.07379689549356,-4.02819886674058,-3.9537384540495,-3.86101999543191,
-3.73754481172534,-3.68200933338862,-3.60630718776622,-3.51625588941678,
-3.44270748925475,-3.35041373882792,-3.31227071068859,-3.22916600496052,
-3.152630467389,-3.05870243760212,-2.98464627030377,-2.93070219305535,-2.80439495350426,
-2.7743415054773,-2.70479137599409,-2.63583136164712,-2.58599116243935,
-2.45147919427703,-2.42137023471592,-2.35121774453874,-2.28694477035531,
-2.23994077889129,-2.19423332184233,-2.11283929689295,-2.03650221126673,
-1.95350491978024,-1.91531982736376,-1.82271481509619,-1.74911013529705,
-1.65920040265371,-1.58322961500161,-1.52738154155305,-1.40443151681069,
-1.37438276335948,-1.34002301095097,-1.25833941339007,-1.21907386153295,
-1.18046317812505,-1.05285490106838,-0.961457005362473,-0.886851249105894,
-0.841215261431666,-0.772329900198776,-0.698570457072661,-0.609018057937201,
-0.532354612408258,-0.475745252674886,-0.354073539092338,-0.294795850899468,
-0.249839284278359),.UNSPECIFIED.);
#606=B_SPLINE_CURVE_WITH_KNOTS('',3,(#75534,#75535,#75536,#75537,#75538,
#75539,#75540,#75541,#75542,#75543,#75544,#75545,#75546,#75547,#75548),
 .UNSPECIFIED.,.F.,.F.,(4,1,1,1,1,1,1,1,1,1,1,1,4),(51.9303482698305,52.3808052628696,
52.8796700748969,53.3785348869242,53.8773996989515,54.3762645109789,54.8751293230062,
55.3739941350335,55.8728589470609,56.3717237590882,56.8705885711155,57.3694533831428,
57.8577774402384),.UNSPECIFIED.);
#607=B_SPLINE_CURVE_WITH_KNOTS('',3,(#75549,#75550,#75551,#75552,#75553,
#75554,#75555,#75556,#75557,#75558,#75559,#75560),.UNSPECIFIED.,.F.,.F.,
(4,2,2,2,2,4),(-4.91076763008672,-4.89054942255246,-4.79539761919939,-4.7359292169242,
-4.67338213757578,-4.661040529428),.UNSPECIFIED.);
#608=B_SPLINE_CURVE_WITH_KNOTS('',3,(#75562,#75563,#75564,#75565,#75566,
#75567,#75568,#75569,#75570,#75571,#75572,#75573),.UNSPECIFIED.,.F.,.F.,
(4,2,2,2,2,4),(-0.249839284278359,-0.192910272014258,-0.153865892167779,
-0.098709197194812,-0.0384561197471015,-0.000114506416299162),
 .UNSPECIFIED.);
#609=B_SPLINE_CURVE_WITH_KNOTS('',3,(#75574,#75575,#75576,#75577,#75578,
#75579,#75580,#75581,#75582,#75583,#75584,#75585,#75586,#75587,#75588,#75589,
#75590,#75591,#75592,#75593,#75594,#75595,#75596,#75597,#75598,#75599,#75600,
#75601,#75602,#75603,#75604,#75605,#75606,#75607,#75608,#75609,#75610,#75611,
#75612,#75613,#75614,#75615,#75616,#75617,#75618,#75619,#75620,#75621,#75622,
#75623,#75624,#75625,#75626,#75627,#75628,#75629,#75630,#75631,#75632,#75633,
#75634,#75635,#75636,#75637,#75638,#75639,#75640,#75641,#75642,#75643,#75644,
#75645,#75646,#75647,#75648,#75649,#75650,#75651,#75652,#75653,#75654,#75655,
#75656,#75657,#75658,#75659,#75660,#75661,#75662,#75663,#75664,#75665,#75666,
#75667,#75668,#75669,#75670,#75671,#75672,#75673,#75674,#75675,#75676,#75677,
#75678,#75679,#75680,#75681,#75682,#75683,#75684,#75685,#75686,#75687,#75688,
#75689,#75690,#75691,#75692,#75693,#75694,#75695,#75696,#75697,#75698,#75699,
#75700,#75701,#75702,#75703,#75704,#75705,#75706,#75707,#75708,#75709,#75710,
#75711,#75712,#75713,#75714,#75715,#75716,#75717,#75718,#75719,#75720,#75721,
#75722,#75723,#75724,#75725,#75726,#75727,#75728,#75729,#75730,#75731,#75732,
#75733,#75734,#75735,#75736,#75737,#75738,#75739,#75740,#75741,#75742,#75743,
#75744,#75745,#75746,#75747,#75748,#75749,#75750,#75751,#75752,#75753,#75754,
#75755,#75756,#75757,#75758,#75759,#75760,#75761,#75762,#75763,#75764,#75765,
#75766,#75767,#75768,#75769,#75770,#75771,#75772,#75773,#75774,#75775,#75776,
#75777,#75778,#75779,#75780,#75781,#75782,#75783,#75784,#75785,#75786,#75787,
#75788,#75789,#75790,#75791,#75792,#75793,#75794,#75795,#75796,#75797,#75798,
#75799,#75800,#75801,#75802,#75803,#75804,#75805,#75806,#75807,#75808,#75809,
#75810,#75811,#75812,#75813,#75814,#75815,#75816,#75817,#75818,#75819,#75820,
#75821,#75822,#75823),.UNSPECIFIED.,.F.,.F.,(4,3,3,3,3,3,3,3,3,3,3,3,3,
3,3,3,3,3,3,3,3,3,3,3,3,3,3,3,3,3,3,3,3,3,3,3,3,3,3,3,3,3,3,3,3,3,3,3,3,
3,3,3,3,3,3,3,3,3,3,3,3,3,3,3,3,3,3,3,3,3,3,3,3,3,3,3,3,3,3,3,3,3,3,4),
(-54.1185379116474,-54.0370154397113,-53.9554652497997,-53.8773996989515,
-53.7969976029293,-53.7166107711432,-53.6320918000885,-53.5517075662432,
-53.4713225283434,-53.3909212255061,-53.3785348869242,-53.2981327907243,
-53.2177459587585,-53.1332269877931,-53.0528427537661,-52.9724577156843,
-52.8920564126664,-52.8796700748969,-52.7992679787358,-52.7188811468092,
-52.6343621758243,-52.5539779418364,-52.4735929037938,-52.3931916008148,
-52.3808052628695,-52.3004031667197,-52.2200163348046,-52.135497363814,
-52.0551131298381,-51.9747280918076,-51.8943267888406,-51.8819404508422,
-51.8015383546724,-51.721151522737,-51.6366325517565,-51.55624831776,-51.4758632797088,
-51.3954619767211,-51.3830756388149,-51.3026735426601,-51.2222867107398,
-51.1377677397518,-51.0573835057707,-50.9769984677349,-50.8965971647625,
-50.8842108267876,-50.8038087306244,-50.7234218986957,-50.6389029277118,
-50.5585186937222,-50.4781336556778,-50.3977323526969,-50.3853460147602,
-50.3049439186006,-50.2245570866755,-50.1400381156899,-50.0596538817039,
-49.9792688436632,-49.8988675406859,-49.8864812027329,-49.8060791065723,
-49.7256922746463,-49.6411733036611,-49.5607890696742,-49.4804040316324,
-49.4000027286542,-49.3876163907056,-49.307214294545,-49.226827462619,-49.1423084916338,
-49.0619242576469,-48.9815392196051,-48.9011379166269,-48.8887515786783,
-48.8083494825178,-48.7279626505919,-48.6434436796066,-48.5630594456198,
-48.4826744075783,-48.4022731045999,-48.3898867666509,-48.3094854295042,
-48.2290975551199,-48.1910843038492),.UNSPECIFIED.);
#610=B_SPLINE_CURVE_WITH_KNOTS('',3,(#75829,#75830,#75831,#75832,#75833,
#75834,#75835,#75836,#75837,#75838,#75839,#75840,#75841,#75842,#75843,#75844,
#75845,#75846,#75847,#75848,#75849,#75850,#75851,#75852,#75853,#75854,#75855,
#75856,#75857,#75858,#75859,#75860,#75861,#75862,#75863,#75864,#75865,#75866,
#75867,#75868,#75869,#75870,#75871,#75872,#75873,#75874,#75875,#75876,#75877,
#75878,#75879,#75880,#75881,#75882,#75883,#75884,#75885,#75886,#75887,#75888,
#75889,#75890,#75891,#75892,#75893,#75894,#75895,#75896,#75897,#75898,#75899,
#75900,#75901,#75902,#75903,#75904,#75905,#75906,#75907,#75908,#75909,#75910,
#75911,#75912,#75913,#75914,#75915,#75916,#75917,#75918,#75919,#75920,#75921,
#75922,#75923,#75924,#75925,#75926,#75927,#75928,#75929,#75930,#75931,#75932,
#75933,#75934,#75935,#75936,#75937,#75938,#75939,#75940,#75941,#75942,#75943,
#75944,#75945,#75946,#75947,#75948,#75949,#75950,#75951,#75952,#75953,#75954,
#75955,#75956,#75957,#75958,#75959,#75960,#75961,#75962,#75963,#75964,#75965,
#75966,#75967,#75968,#75969,#75970,#75971,#75972,#75973,#75974,#75975,#75976,
#75977,#75978,#75979,#75980,#75981,#75982,#75983,#75984,#75985,#75986,#75987,
#75988,#75989,#75990,#75991,#75992,#75993,#75994,#75995,#75996,#75997,#75998,
#75999,#76000,#76001,#76002,#76003,#76004,#76005,#76006,#76007,#76008,#76009,
#76010,#76011,#76012,#76013,#76014,#76015,#76016,#76017,#76018,#76019,#76020,
#76021,#76022,#76023,#76024,#76025,#76026,#76027,#76028,#76029,#76030,#76031,
#76032,#76033,#76034,#76035,#76036,#76037,#76038,#76039,#76040,#76041,#76042,
#76043,#76044,#76045,#76046,#76047,#76048,#76049,#76050,#76051,#76052,#76053,
#76054,#76055,#76056,#76057,#76058,#76059,#76060,#76061,#76062,#76063,#76064,
#76065,#76066,#76067,#76068,#76069,#76070,#76071,#76072,#76073,#76074,#76075,
#76076,#76077,#76078),.UNSPECIFIED.,.F.,.F.,(4,3,3,3,3,3,3,3,3,3,3,3,3,
3,3,3,3,3,3,3,3,3,3,3,3,3,3,3,3,3,3,3,3,3,3,3,3,3,3,3,3,3,3,3,3,3,3,3,3,
3,3,3,3,3,3,3,3,3,3,3,3,3,3,3,3,3,3,3,3,3,3,3,3,3,3,3,3,3,3,3,3,3,3,4),
(45.6471469631167,45.7275310616107,45.8115468840625,45.8955627065143,45.9759648026746,
46.0563516346004,46.1408706055857,46.2212548395724,46.3016398776137,46.3820411805914,
46.3944275185416,46.474829614702,46.5552164466278,46.6397354176131,46.7201196515999,
46.8005046896415,46.8809059926195,46.8932923305689,46.9736944267296,47.0540812586556,
47.1386002296408,47.2189844636279,47.2993695016697,47.3797708046479,47.3921571425963,
47.4725592387567,47.5529460706825,47.6374650416678,47.7178492756546,47.7982343136961,
47.878635616674,47.8910219546236,47.9714240507842,48.0518108827102,48.1363298536954,
48.2167140876824,48.297099125724,48.3775004287023,48.3898867666509,48.4702888628112,
48.5506756947369,48.6351946657222,48.7155788997089,48.7959639377504,48.8763652407283,
48.8887515786782,48.969153674839,49.0495405067652,49.1340594777503,49.2144437117374,
49.2948287497792,49.3752300527577,49.3876163907056,49.4680184868661,49.5484053187922,
49.6329242897774,49.7133085237644,49.793693561806,49.874094864784,49.8864812027329,
49.9668832988924,50.0472701308175,50.1317891018032,50.212173335789,50.2925583738295,
50.3729596768067,50.3853460147602,50.4657481109236,50.5461349428522,50.6306539138361,
50.7110381478257,50.7914231858703,50.871824488851,50.8842108267876,50.9646129229422,
51.0449997548621,51.1295187258503,51.2099029598313,51.290287997867,51.3706893008394,
51.3830756388149,51.4656515093945,51.5482033685856,51.5745921485727),
 .UNSPECIFIED.);
#611=B_SPLINE_CURVE_WITH_KNOTS('',3,(#76079,#76080,#76081,#76082,#76083),
 .UNSPECIFIED.,.F.,.F.,(4,1,4),(51.5745921485727,51.8819404508422,51.9303482698305),
 .UNSPECIFIED.);
#612=B_SPLINE_CURVE_WITH_KNOTS('',3,(#76085,#76086,#76087,#76088,#76089,
#76090,#76091,#76092,#76093,#76094,#76095,#76096,#76097,#76098,#76099,#76100),
 .UNSPECIFIED.,.F.,.F.,(4,3,3,3,3,4),(-48.1910843038492,-48.1106976837031,
-48.030313872139,-47.9499108869887,-47.8910219546236,-47.8353526044678),
 .UNSPECIFIED.);
#613=B_SPLINE_CURVE_WITH_KNOTS('',3,(#76101,#76102,#76103,#76104,#76105,
#76106,#76107,#76108,#76109,#76110,#76111,#76112,#76113,#76114,#76115,#76116,
#76117,#76118,#76119,#76120,#76121,#76122,#76123,#76124,#76125,#76126,#76127,
#76128,#76129,#76130,#76131,#76132,#76133,#76134,#76135,#76136,#76137,#76138,
#76139,#76140,#76141,#76142,#76143,#76144,#76145,#76146,#76147,#76148,#76149,
#76150,#76151,#76152,#76153,#76154,#76155,#76156,#76157,#76158,#76159,#76160,
#76161,#76162,#76163,#76164,#76165,#76166,#76167,#76168,#76169,#76170,#76171,
#76172,#76173,#76174,#76175,#76176,#76177,#76178,#76179,#76180,#76181,#76182,
#76183,#76184,#76185,#76186,#76187,#76188,#76189,#76190,#76191,#76192,#76193,
#76194,#76195,#76196,#76197,#76198,#76199,#76200,#76201,#76202,#76203,#76204,
#76205,#76206,#76207,#76208,#76209,#76210,#76211,#76212),.UNSPECIFIED.,
 .F.,.F.,(4,2,2,2,2,2,2,2,2,2,2,2,2,2,2,2,2,2,2,2,2,2,2,2,2,2,2,2,2,2,2,
2,2,2,2,2,2,2,2,2,2,2,2,2,2,2,2,2,2,2,2,2,2,2,2,4),(-8.82308834836121,-8.69631405692605,
-8.66999828107067,-8.54091357144238,-8.50792268417827,-8.43201046834799,
-8.338862235828,-8.21679152542147,-8.16041651382544,-8.08395624499135,-7.99428699052817,
-7.92057172446897,-7.85131090598304,-7.80584059133933,-7.73170485979139,
-7.63942132907712,-7.5135137114328,-7.47436040599107,-7.43534619183455,
-7.35113770563209,-7.291786734327,-7.15768916435272,-7.10765366824809,-7.03840883283788,
-6.9692180267347,-6.93916039717996,-6.81228266182114,-6.75864265335129,
-6.68492027824907,-6.6174717547749,-6.58742052764269,-6.46581143634332,
-6.40915891083922,-6.33245179385895,-6.24291004586388,-6.16913900776438,
-6.06814460197658,-6.0259275516604,-5.94620168726619,-5.88691766352201,
-5.76524317810062,-5.70862762352981,-5.63195257300178,-5.54239176883554,
-5.46862692200963,-5.39974181860447,-5.35410188266291,-5.27948505219832,
-5.18652146927599,-5.06438139706198,-5.00804798984591,-4.93162521274094,
-4.84193673418545,-4.76822994855434,-4.69885186192799,-4.66124588486828),
 .UNSPECIFIED.);
#614=B_SPLINE_CURVE_WITH_KNOTS('',3,(#76218,#76219,#76220,#76221,#76222,
#76223,#76224,#76225,#76226,#76227,#76228,#76229,#76230,#76231,#76232,#76233,
#76234,#76235,#76236,#76237,#76238,#76239,#76240,#76241,#76242,#76243,#76244,
#76245,#76246,#76247,#76248,#76249,#76250,#76251,#76252,#76253,#76254,#76255,
#76256,#76257,#76258,#76259,#76260,#76261,#76262,#76263,#76264,#76265,#76266,
#76267,#76268,#76269,#76270,#76271,#76272,#76273,#76274,#76275,#76276,#76277,
#76278,#76279,#76280,#76281,#76282,#76283,#76284,#76285,#76286,#76287,#76288,
#76289,#76290,#76291,#76292,#76293,#76294,#76295,#76296,#76297,#76298,#76299,
#76300,#76301,#76302,#76303,#76304,#76305,#76306,#76307,#76308,#76309,#76310,
#76311,#76312,#76313,#76314,#76315,#76316,#76317,#76318,#76319,#76320,#76321,
#76322,#76323,#76324,#76325,#76326,#76327,#76328,#76329,#76330,#76331),
 .UNSPECIFIED.,.F.,.F.,(4,2,2,2,2,2,2,2,2,2,2,2,2,2,2,2,2,2,2,2,2,2,2,2,
2,2,2,2,2,2,2,2,2,2,2,2,2,2,2,2,2,2,2,2,2,2,2,2,2,2,2,2,2,2,2,2,4),(-4.16167409877826,
-4.14888454665581,-4.11080878728497,-4.01816330560154,-3.94527840833286,
-3.91504806802662,-3.84264795681711,-3.78287916929053,-3.73471581770899,
-3.60099813523087,-3.50826304914553,-3.43415092475662,-3.38868875064578,
-3.3194187215629,-3.24570792663102,-3.15604587741013,-3.07959623958393,
-3.02322670589989,-2.90115708907312,-2.80795727498646,-2.73364439917479,
-2.68811150026171,-2.61897598470416,-2.54525427184331,-2.45561283870726,
-2.37911898605323,-2.32270069107514,-2.20070879838926,-2.17065969565455,
-2.13637842611587,-2.05480989617438,-2.01540853311985,-1.97705260970872,
-1.84989807897117,-1.75770150776069,-1.68280150972009,-1.63706104876533,
-1.49460844929561,-1.40530489135814,-1.32815945043843,-1.2709924151342,
-1.15023580496727,-1.05696856452268,-0.982305019221087,-0.936648409373202,
-0.867832919528015,-0.794053713764026,-0.704542709873163,-0.627795627335843,
-0.571091675400024,-0.449573467515136,-0.390294377617773,-0.288476142994649,
-0.249335000370875,-0.114036524571827,-0.0706819242005296,-0.000108410259028435),
 .UNSPECIFIED.);
#615=B_SPLINE_CURVE_WITH_KNOTS('',3,(#76332,#76333,#76334,#76335,#76336,
#76337,#76338,#76339,#76340,#76341,#76342,#76343,#76344,#76345,#76346,#76347,
#76348,#76349,#76350),.UNSPECIFIED.,.F.,.F.,(4,3,3,3,3,3,4),(45.2914068413931,
45.3766260457133,45.3966978944869,45.4771000160926,45.5574858748033,45.637864107376,
45.6471469631167),.UNSPECIFIED.);
#616=B_SPLINE_CURVE_WITH_KNOTS('',3,(#76351,#76352,#76353,#76354,#76355,
#76356,#76357,#76358,#76359,#76360,#76361,#76362,#76363,#76364,#76365,#76366,
#76367,#76368,#76369,#76370,#76371,#76372,#76373,#76374,#76375,#76376,#76377,
#76378,#76379,#76380,#76381,#76382,#76383,#76384,#76385,#76386,#76387,#76388,
#76389,#76390,#76391,#76392,#76393,#76394,#76395,#76396,#76397,#76398,#76399,
#76400,#76401,#76402,#76403,#76404,#76405,#76406,#76407,#76408,#76409,#76410,
#76411,#76412,#76413,#76414,#76415,#76416,#76417,#76418,#76419,#76420,#76421,
#76422,#76423,#76424,#76425,#76426,#76427,#76428,#76429,#76430,#76431,#76432,
#76433,#76434,#76435,#76436,#76437,#76438,#76439,#76440,#76441,#76442,#76443,
#76444,#76445,#76446,#76447,#76448,#76449,#76450,#76451,#76452,#76453,#76454,
#76455,#76456,#76457,#76458,#76459,#76460,#76461,#76462,#76463,#76464,#76465,
#76466,#76467,#76468,#76469,#76470),.UNSPECIFIED.,.F.,.F.,(4,2,2,2,2,2,
2,2,2,2,2,2,2,2,2,2,2,2,2,2,2,2,2,2,2,2,2,2,2,2,2,2,2,2,2,2,2,2,2,2,2,2,
2,2,2,2,2,2,2,2,2,2,2,2,2,2,2,2,2,4),(-4.66124588486828,-4.65344182834346,
-4.57947860386115,-4.48869940087069,-4.41147586212013,-4.32801044803778,
-4.28994307687754,-4.24560544594292,-4.13722203158076,-4.05809115658597,
-3.96022500483084,-3.90631313505404,-3.77993448887484,-3.68712977428591,
-3.60884781406385,-3.55026396953155,-3.43174175045692,-3.3382346457669,
-3.2631698219336,-3.21736953987103,-3.07535718732895,-2.9868208205041,-2.90817316169504,
-2.84909713122432,-2.73132982588684,-2.63447581380076,-2.55859404202909,
-2.50284231628825,-2.37971692288725,-2.32044065727856,-2.24058148245293,
-2.19861559446752,-2.18067847794665,-2.12669884520124,-2.03759783927625,
-1.96140012860537,-1.8784789597153,-1.84025601220625,-1.74728669698988,
-1.67371290461062,-1.58372363507163,-1.50789987830291,-1.45220897795329,
-1.3289842823785,-1.26970952277594,-1.1898420329682,-1.14789481369276,-1.12995121607658,
-1.07593299471434,-0.986902782999391,-0.910709935639108,-0.827792353068139,
-0.789569337301891,-0.696593795183355,-0.623022349692111,-0.533033224461751,
-0.457214579369248,-0.401528548325178,-0.280196426907405,-0.249814737108548),
 .UNSPECIFIED.);
#617=B_SPLINE_CURVE_WITH_KNOTS('',3,(#76475,#76476,#76477,#76478,#76479,
#76480,#76481,#76482,#76483,#76484,#76485,#76486,#76487,#76488,#76489,#76490,
#76491,#76492,#76493,#76494,#76495,#76496,#76497,#76498,#76499,#76500,#76501,
#76502,#76503,#76504,#76505,#76506,#76507,#76508,#76509,#76510,#76511,#76512,
#76513,#76514,#76515,#76516,#76517,#76518,#76519,#76520,#76521,#76522,#76523,
#76524,#76525,#76526,#76527,#76528,#76529,#76530,#76531,#76532,#76533,#76534,
#76535,#76536,#76537,#76538,#76539,#76540,#76541,#76542,#76543,#76544,#76545,
#76546,#76547,#76548,#76549,#76550,#76551,#76552,#76553,#76554,#76555,#76556,
#76557,#76558,#76559,#76560,#76561,#76562,#76563,#76564,#76565,#76566,#76567,
#76568,#76569,#76570,#76571,#76572,#76573,#76574,#76575,#76576,#76577,#76578,
#76579,#76580,#76581,#76582,#76583,#76584,#76585,#76586,#76587,#76588,#76589,
#76590),.UNSPECIFIED.,.F.,.F.,(4,2,2,2,2,2,2,2,2,2,2,2,2,2,2,2,2,2,2,2,
2,2,2,2,2,2,2,2,2,2,2,2,2,2,2,2,2,2,2,2,2,2,2,2,2,2,2,2,2,2,2,2,2,2,2,2,
2,4),(-8.57312334748902,-8.53068440591889,-8.4654296892502,-8.3748028049429,
-8.32771669325542,-8.26328253987196,-8.19317209872651,-8.16306359739018,
-8.02872601189461,-7.97880430771087,-7.90972087403233,-7.84032131490915,
-7.81026567485648,-7.68371741211631,-7.62990290151605,-7.55598834015279,
-7.48859632118536,-7.45854586530168,-7.33728694601201,-7.2804261156745,
-7.20353791991617,-7.11409370843184,-7.04028315253009,-6.97158618850328,
-6.92589708093375,-6.85113848639895,-6.7578405474679,-6.63747357215866,
-6.58006645651545,-6.50271548725764,-6.41351209753925,-6.27111868167746,
-6.22537060865583,-6.15044581089919,-6.05708645490686,-5.93749777875824,
-5.87960385331488,-5.80185639149972,-5.71285790968482,-5.57058277654793,
-5.52481997348399,-5.44985356946362,-5.35715840607209,-5.23506542432103,
-5.17871172553286,-5.10227213746364,-5.01260018449415,-4.93889309841728,
-4.86958586254518,-4.82414441152635,-4.75008766188793,-4.65834226292778,
-4.52079689347961,-4.47443898077894,-4.41144438421492,-4.30925568253923,
-4.23223994902498,-4.16167409877826),.UNSPECIFIED.);
#618=B_SPLINE_CURVE_WITH_KNOTS('',3,(#76592,#76593,#76594,#76595,#76596,
#76597,#76598,#76599,#76600,#76601),.UNSPECIFIED.,.F.,.F.,(4,2,2,2,4),(-0.249814737108548,
-0.220876598911715,-0.110400142751405,-0.0942961602729965,-6.03191603578172E-5),
 .UNSPECIFIED.);
#619=B_SPLINE_CURVE_WITH_KNOTS('',3,(#76602,#76603,#76604,#76605,#76606,
#76607,#76608,#76609,#76610,#76611,#76612,#76613,#76614,#76615,#76616,#76617),
 .UNSPECIFIED.,.F.,.F.,(4,1,1,1,1,1,1,1,1,1,1,1,1,4),(-35.2689819901086,
-34.920536841913,-34.4216720298857,-33.9228072178584,-33.4239424058311,
-32.9250775938037,-32.4262127817764,-31.9273479697491,-31.4284831577217,
-30.9296183456944,-30.4307535336671,-29.9318887216397,-29.4330239096124,
-29.3415126415508),.UNSPECIFIED.);
#620=B_SPLINE_CURVE_WITH_KNOTS('',3,(#76623,#76624,#76625,#76626,#76627,
#76628,#76629,#76630,#76631,#76632,#76633,#76634,#76635,#76636,#76637,#76638,
#76639,#76640,#76641,#76642,#76643,#76644,#76645,#76646,#76647,#76648,#76649,
#76650,#76651,#76652,#76653,#76654,#76655,#76656,#76657,#76658,#76659,#76660,
#76661,#76662,#76663,#76664,#76665,#76666,#76667,#76668,#76669,#76670,#76671,
#76672,#76673,#76674,#76675,#76676,#76677,#76678,#76679,#76680,#76681,#76682,
#76683,#76684,#76685,#76686,#76687,#76688,#76689,#76690,#76691,#76692,#76693,
#76694,#76695,#76696,#76697,#76698,#76699,#76700,#76701,#76702,#76703,#76704,
#76705,#76706,#76707,#76708,#76709,#76710,#76711,#76712,#76713,#76714,#76715,
#76716,#76717,#76718,#76719,#76720,#76721,#76722,#76723,#76724,#76725,#76726,
#76727,#76728,#76729,#76730,#76731,#76732,#76733,#76734,#76735,#76736,#76737,
#76738,#76739,#76740,#76741,#76742,#76743,#76744,#76745,#76746),
 .UNSPECIFIED.,.F.,.F.,(4,2,2,2,2,2,2,2,2,2,2,2,2,2,2,2,2,2,2,2,2,2,2,2,
2,2,2,2,2,2,2,2,2,2,2,2,2,2,2,2,2,2,2,2,2,2,2,2,2,2,2,2,2,2,2,2,2,2,2,2,
2,4),(-4.16167874312325,-4.13977816237221,-4.06388049611118,-4.00811359479904,
-3.88500006385136,-3.8257199464703,-3.74585757730773,-3.70388552452625,
-3.68594859760857,-3.63197326719183,-3.54285304205606,-3.46664983935468,
-3.38372298659274,-3.34549775091462,-3.25252395247419,-3.17894528630053,
-3.08895064772496,-3.01312119614296,-2.95742594007616,-2.83419463348202,
-2.77491606531558,-2.69504356719102,-2.65309339842942,-2.63514875108143,
-2.58112766114741,-2.49209066550481,-2.41589291548282,-2.33296997835701,
-2.29474451174723,-2.20176298173821,-2.12818680192912,-2.03819197996319,
-1.96236827599743,-1.90667856023484,-1.78344247663634,-1.72416520137181,
-1.64429369072946,-1.60234572141077,-1.5844009584494,-1.53037812481442,
-1.44134808067491,-1.36515220491252,-1.28223118400461,-1.24400647602509,
-1.15102635292996,-1.07745181290136,-0.987458799240072,-0.91163698014631,
-0.855948729445594,-0.732714845060695,-0.673438847420675,-0.593569012083775,
-0.551622025519284,-0.533677618286453,-0.479655770120658,-0.392556161143309,
-0.33232033472783,-0.244435098865594,-0.204569805683055,-0.171101035364585,
-0.0522159782253246,-6.02492052133978E-5),.UNSPECIFIED.);
#621=B_SPLINE_CURVE_WITH_KNOTS('',3,(#76747,#76748,#76749,#76750,#76751,
#76752,#76753,#76754,#76755,#76756),.UNSPECIFIED.,.F.,.F.,(4,2,2,2,4),(-8.82288650888697,
-8.71171349505023,-8.67904854995692,-8.59378203487709,-8.57312334748902),
 .UNSPECIFIED.);
#622=B_SPLINE_CURVE_WITH_KNOTS('',3,(#76758,#76759,#76760,#76761),
 .UNSPECIFIED.,.F.,.F.,(4,4),(-29.3415126415508,-28.9857967263874),
 .UNSPECIFIED.);
#623=B_SPLINE_CURVE_WITH_KNOTS('',3,(#76762,#76763,#76764,#76765,#76766,
#76767,#76768,#76769,#76770,#76771,#76772,#76773,#76774,#76775,#76776,#76777,
#76778,#76779,#76780,#76781,#76782,#76783,#76784,#76785,#76786,#76787,#76788,
#76789,#76790,#76791,#76792,#76793,#76794,#76795,#76796,#76797,#76798,#76799,
#76800,#76801,#76802,#76803,#76804,#76805,#76806,#76807,#76808,#76809,#76810,
#76811,#76812,#76813,#76814,#76815,#76816,#76817,#76818,#76819,#76820,#76821,
#76822,#76823,#76824,#76825,#76826,#76827,#76828,#76829,#76830,#76831,#76832,
#76833,#76834,#76835,#76836,#76837,#76838,#76839,#76840,#76841,#76842,#76843,
#76844,#76845,#76846,#76847,#76848,#76849,#76850,#76851,#76852,#76853,#76854,
#76855,#76856,#76857,#76858,#76859,#76860,#76861,#76862,#76863,#76864,#76865,
#76866,#76867,#76868,#76869,#76870,#76871,#76872,#76873,#76874,#76875,#76876,
#76877,#76878,#76879,#76880,#76881,#76882,#76883,#76884,#76885,#76886,#76887,
#76888,#76889,#76890,#76891,#76892,#76893,#76894,#76895,#76896,#76897,#76898,
#76899,#76900,#76901,#76902,#76903,#76904,#76905,#76906,#76907,#76908,#76909,
#76910,#76911,#76912,#76913,#76914,#76915,#76916,#76917,#76918,#76919,#76920,
#76921,#76922,#76923,#76924,#76925,#76926,#76927,#76928,#76929,#76930,#76931,
#76932,#76933,#76934,#76935,#76936,#76937,#76938,#76939,#76940,#76941,#76942,
#76943,#76944,#76945,#76946,#76947,#76948,#76949,#76950,#76951,#76952,#76953,
#76954,#76955,#76956,#76957,#76958,#76959,#76960,#76961,#76962,#76963,#76964,
#76965,#76966,#76967,#76968,#76969,#76970,#76971,#76972,#76973,#76974,#76975,
#76976,#76977,#76978,#76979,#76980,#76981,#76982,#76983,#76984,#76985,#76986,
#76987,#76988,#76989,#76990,#76991,#76992,#76993,#76994,#76995,#76996,#76997,
#76998,#76999,#77000,#77001,#77002,#77003,#77004,#77005,#77006,#77007,#77008,
#77009,#77010,#77011),.UNSPECIFIED.,.F.,.F.,(4,3,3,3,3,3,3,3,3,3,3,3,3,
3,3,3,3,3,3,3,3,3,3,3,3,3,3,3,3,3,3,3,3,3,3,3,3,3,3,3,3,3,3,3,3,3,3,3,3,
3,3,3,3,3,3,3,3,3,3,3,3,3,3,3,3,3,3,3,3,3,3,3,3,3,3,3,3,3,3,3,3,3,3,4),
(-28.985796682929,-28.9341590975851,-28.8537570014243,-28.7733701694982,
-28.6888511985131,-28.608466964526,-28.5280819264842,-28.4476806235058,
-28.4352942855578,-28.3548921893973,-28.2745053574713,-28.1899863864861,
-28.1096021524991,-28.0292171144574,-27.9488158114792,-27.9364294735304,
-27.8560273773699,-27.775640545444,-27.6911215744588,-27.6107373404719,
-27.5303523024302,-27.4499509994519,-27.4375646615031,-27.3571625653427,
-27.2767757334169,-27.1922567624316,-27.1118725284448,-27.0314874904033,
-26.9510861874253,-26.9386998494758,-26.8582977533151,-26.7779109213891,
-26.6933919504039,-26.6130077164169,-26.5326226783752,-26.4522213753969,
-26.4398350374484,-26.3594329412879,-26.279046109362,-26.1945271383768,
-26.1141429043899,-26.0337578663484,-25.9533565633703,-25.9409702254211,
-25.8605681292606,-25.7801812973347,-25.6956623263495,-25.6152780923626,
-25.534893054321,-25.4544917513429,-25.4421054133938,-25.3617033172334,
-25.2813164853074,-25.1967975143222,-25.1164132803353,-25.0360282422938,
-24.9556269393158,-24.9432406013665,-24.8628385052059,-24.7824516732798,
-24.6979327022946,-24.6175484683076,-24.5371634302657,-24.4567621272875,
-24.4443757893391,-24.3639736931787,-24.2835868612527,-24.1990678902675,
-24.1186836562807,-24.0382986182391,-23.9578973152611,-23.9455109773118,
-23.8651088811514,-23.7847220492255,-23.7002030782402,-23.6198188442535,
-23.5394338062118,-23.4590325032338,-23.4466461652845,-23.3662448479451,
-23.285852924114,-23.2054721193945,-23.1250839303849,-23.0583686585911),
 .UNSPECIFIED.);
#624=B_SPLINE_CURVE_WITH_KNOTS('',3,(#77016,#77017,#77018,#77019,#77020,
#77021,#77022,#77023,#77024,#77025,#77026,#77027,#77028,#77029,#77030,#77031,
#77032,#77033,#77034,#77035,#77036,#77037,#77038,#77039,#77040,#77041,#77042,
#77043,#77044,#77045,#77046,#77047,#77048,#77049,#77050,#77051,#77052,#77053,
#77054,#77055,#77056,#77057,#77058,#77059,#77060,#77061,#77062,#77063,#77064,
#77065,#77066,#77067,#77068,#77069,#77070,#77071,#77072,#77073,#77074,#77075,
#77076,#77077,#77078,#77079,#77080,#77081,#77082,#77083,#77084,#77085,#77086,
#77087,#77088,#77089,#77090,#77091,#77092,#77093,#77094,#77095,#77096,#77097,
#77098,#77099,#77100,#77101,#77102,#77103,#77104,#77105,#77106,#77107,#77108,
#77109,#77110,#77111,#77112,#77113,#77114,#77115,#77116,#77117,#77118,#77119,
#77120,#77121,#77122,#77123,#77124,#77125,#77126,#77127,#77128,#77129,#77130,
#77131,#77132,#77133,#77134,#77135),.UNSPECIFIED.,.F.,.F.,(4,2,2,2,2,2,
2,2,2,2,2,2,2,2,2,2,2,2,2,2,2,2,2,2,2,2,2,2,2,2,2,2,2,2,2,2,2,2,2,2,2,2,
2,2,2,2,2,2,2,2,2,2,2,2,2,2,2,2,2,4),(-8.57349042528258,-8.50240203114283,
-8.44311233837328,-8.32177381469027,-8.26494522658923,-8.18808157627475,
-8.09860869091554,-8.02479679024485,-7.95606253684597,-7.91037569565218,
-7.83563020571102,-7.74246179007927,-7.62144835948341,-7.5644236567328,
-7.48739142584248,-7.39800775582466,-7.32415808945513,-7.255568507469,-7.20984296726339,
-7.13498747216309,-7.04250844937971,-6.9192083019533,-6.86355308775394,
-6.78775701139477,-6.70050107791662,-6.62925888618261,-6.55243899098011,
-6.53113648448967,-6.49290220350523,-6.40998705866415,-6.33381030377695,
-6.24537862779375,-6.17187471117095,-6.1290007426219,-6.04156739607458,
-6.0099834571062,-5.94349244325072,-5.85577273817698,-5.80927108606505,
-5.73226979830522,-5.64224811960476,-5.51616143268776,-5.4620834394515,
-5.38788160507939,-5.32056152450713,-5.29050788914231,-5.16974614834047,
-5.11256874790466,-5.03540705044408,-4.94609198457278,-4.80362475543783,
-4.75787902692566,-4.68296669317975,-4.59075784987658,-4.46663687636836,
-4.41145636881902,-4.3956249802366,-4.30333527342906,-4.22974040858213,
-4.16167874312325),.UNSPECIFIED.);
#625=B_SPLINE_CURVE_WITH_KNOTS('',3,(#77137,#77138,#77139,#77140,#77141,
#77142,#77143,#77144,#77145,#77146,#77147,#77148,#77149,#77150,#77151,#77152),
 .UNSPECIFIED.,.F.,.F.,(4,3,3,3,3,4),(-23.0583686585911,-22.9779671089007,
-22.9477813532571,-22.8663024476233,-22.7844569116864,-22.7026113757494),
 .UNSPECIFIED.);
#626=B_SPLINE_CURVE_WITH_KNOTS('',3,(#77153,#77154,#77155,#77156,#77157,
#77158,#77159,#77160,#77161,#77162,#77163,#77164,#77165,#77166,#77167,#77168),
 .UNSPECIFIED.,.F.,.F.,(4,1,1,1,1,1,1,1,1,1,1,1,1,4),(-22.7026113757494,
-22.4489165412298,-21.9500517292025,-21.4511869171751,-20.9523221051478,
-20.4534572931205,-19.9545924810932,-19.4557276690658,-18.9568628570385,
-18.4579980450112,-17.9591332329838,-17.4602684209565,-16.9614036089292,
-16.7751485430145),.UNSPECIFIED.);
#627=B_SPLINE_CURVE_WITH_KNOTS('',3,(#77174,#77175,#77176,#77177,#77178,
#77179,#77180,#77181,#77182,#77183,#77184,#77185,#77186,#77187,#77188,#77189,
#77190,#77191,#77192,#77193,#77194,#77195,#77196,#77197,#77198,#77199,#77200,
#77201,#77202,#77203,#77204,#77205,#77206,#77207,#77208,#77209,#77210,#77211,
#77212,#77213,#77214,#77215,#77216,#77217,#77218,#77219,#77220,#77221,#77222,
#77223,#77224,#77225,#77226,#77227,#77228,#77229,#77230,#77231,#77232,#77233,
#77234,#77235,#77236,#77237,#77238,#77239,#77240,#77241,#77242,#77243,#77244,
#77245,#77246,#77247,#77248,#77249,#77250,#77251,#77252,#77253,#77254,#77255,
#77256,#77257,#77258,#77259,#77260,#77261,#77262,#77263,#77264,#77265,#77266,
#77267,#77268,#77269,#77270,#77271,#77272,#77273,#77274,#77275,#77276,#77277,
#77278,#77279,#77280,#77281,#77282,#77283,#77284,#77285,#77286,#77287),
 .UNSPECIFIED.,.F.,.F.,(4,2,2,2,2,2,2,2,2,2,2,2,2,2,2,2,2,2,2,2,2,2,2,2,
2,2,2,2,2,2,2,2,2,2,2,2,2,2,2,2,2,2,2,2,2,2,2,2,2,2,2,2,2,2,2,2,4),(-4.16151590151851,
-4.0760948985585,-4.00123840793195,-3.95551321653237,-3.88694412086877,
-3.8130973004708,-3.72373618742032,-3.64669644708721,-3.58965455941888,
-3.46868919783547,-3.40940726048669,-3.32975477505438,-3.2874224169687,
-3.2696219553045,-3.2164269161219,-3.12595598025145,-3.04968479711686,-2.966724037557,
-2.92852260043549,-2.83575016541184,-2.76216092585789,-2.67221648331477,
-2.59631384592066,-2.54053874000987,-2.4174649850203,-2.38741627088776,
-2.35304615139757,-2.27134755770366,-2.23209950901699,-2.19345460782918,
-2.06595660720629,-1.97365271457811,-1.89516962604998,-1.83631426962606,
-1.71822474841647,-1.62467705543961,-1.54955199322482,-1.5037315584742,
-1.36190743973524,-1.27367653035868,-1.19947794667645,-1.15398541021193,
-1.08477368485643,-1.01105839226976,-0.92140554879589,-0.844936999934219,
-0.788546545693046,-0.666510947040339,-0.57375356441514,-0.498854038590726,
-0.45311362129568,-0.369065778336818,-0.301465506272486,-0.240428505417184,
-0.145854057242879,-0.113723193842431,-6.03189471992543E-5),
 .UNSPECIFIED.);
#628=B_SPLINE_CURVE_WITH_KNOTS('',3,(#77288,#77289,#77290,#77291,#77292,
#77293,#77294,#77295,#77296,#77297),.UNSPECIFIED.,.F.,.F.,(4,2,2,2,4),(-8.82332564681183,
-8.77464235640149,-8.64341940293209,-8.60415258924592,-8.57349042528258),
 .UNSPECIFIED.);
#629=B_SPLINE_CURVE_WITH_KNOTS('',3,(#77299,#77300,#77301,#77302,#77303),
 .UNSPECIFIED.,.F.,.F.,(4,1,4),(-16.7751485430145,-16.4625387969019,-16.4194260685698),
 .UNSPECIFIED.);
#630=B_SPLINE_CURVE_WITH_KNOTS('',3,(#77304,#77305,#77306,#77307,#77308,
#77309,#77310,#77311,#77312,#77313,#77314,#77315,#77316,#77317,#77318,#77319,
#77320,#77321,#77322,#77323,#77324,#77325,#77326,#77327,#77328,#77329,#77330,
#77331,#77332,#77333,#77334,#77335,#77336,#77337,#77338,#77339,#77340,#77341,
#77342,#77343,#77344,#77345,#77346,#77347,#77348,#77349,#77350,#77351,#77352,
#77353,#77354,#77355,#77356,#77357,#77358,#77359,#77360,#77361,#77362,#77363,
#77364,#77365,#77366,#77367,#77368,#77369,#77370,#77371,#77372,#77373,#77374,
#77375,#77376,#77377,#77378,#77379,#77380,#77381,#77382,#77383,#77384,#77385,
#77386,#77387,#77388,#77389,#77390,#77391,#77392,#77393,#77394,#77395,#77396,
#77397,#77398,#77399,#77400,#77401,#77402,#77403,#77404,#77405,#77406,#77407,
#77408,#77409,#77410,#77411,#77412,#77413,#77414,#77415,#77416,#77417,#77418,
#77419,#77420,#77421,#77422,#77423,#77424,#77425,#77426,#77427,#77428,#77429,
#77430,#77431,#77432,#77433,#77434,#77435,#77436,#77437,#77438,#77439,#77440,
#77441,#77442,#77443,#77444,#77445,#77446,#77447,#77448,#77449,#77450,#77451,
#77452,#77453,#77454,#77455,#77456,#77457,#77458,#77459,#77460,#77461,#77462,
#77463,#77464,#77465,#77466,#77467,#77468,#77469,#77470,#77471,#77472,#77473,
#77474,#77475,#77476,#77477,#77478,#77479,#77480,#77481,#77482,#77483,#77484,
#77485,#77486,#77487,#77488,#77489,#77490,#77491,#77492,#77493,#77494,#77495,
#77496,#77497,#77498,#77499,#77500,#77501,#77502,#77503,#77504,#77505,#77506,
#77507,#77508,#77509,#77510,#77511,#77512,#77513,#77514,#77515,#77516,#77517,
#77518,#77519,#77520,#77521,#77522,#77523,#77524,#77525,#77526,#77527,#77528,
#77529,#77530,#77531,#77532,#77533,#77534,#77535,#77536,#77537,#77538,#77539,
#77540,#77541,#77542,#77543,#77544,#77545,#77546,#77547,#77548,#77549,#77550),
 .UNSPECIFIED.,.F.,.F.,(4,3,3,3,3,3,3,3,3,3,3,3,3,3,3,3,3,3,3,3,3,3,3,3,
3,3,3,3,3,3,3,3,3,3,3,3,3,3,3,3,3,3,3,3,3,3,3,3,3,3,3,3,3,3,3,3,3,3,3,3,
3,3,3,3,3,3,3,3,3,3,3,3,3,3,3,3,3,3,3,3,3,3,4),(-16.4194260628912,-16.3392758127687,
-16.259140303397,-16.1790020076008,-16.0988669317824,-16.0187124343916,
-15.9636739848745,-15.8832718887138,-15.8028850567879,-15.7183660858027,
-15.6379818518158,-15.5575968137742,-15.4771955107962,-15.4648091728472,
-15.3844070766868,-15.3040202447606,-15.2195012737754,-15.1391170397884,
-15.0587320017468,-14.9783306987688,-14.9659443608199,-14.8855422646602,
-14.8051554327346,-14.7206364617491,-14.640252227763,-14.5598671897221,
-14.4794658867447,-14.4670795487925,-14.3866774526294,-14.3062906207008,
-14.2217716497169,-14.1413874157274,-14.0610023776838,-13.9806010747033,
-13.9682147367652,-13.8878126406106,-13.8074258086903,-13.7229068377022,
-13.6425226037211,-13.5621375656852,-13.4817362627123,-13.4693499247379,
-13.3889478285678,-13.3085609966321,-13.2240420256517,-13.1436577916554,
-13.0632727536049,-12.9828714506176,-12.9704851127106,-12.890083016561,
-12.8096961846458,-12.7251772136551,-12.6447929796791,-12.5644079416484,
-12.4840066386806,-12.4716203006832,-12.391218204522,-12.3108313725956,
-12.2263124016107,-12.1459281676232,-12.065543129581,-11.9851418266027,
-11.9727554886559,-11.8923533924557,-11.8119665604902,-11.7274475895248,
-11.647063355498,-11.5666783174163,-11.4862770143991,-11.4738906766286,
-11.3934885806086,-11.3131017488229,-11.2285827777675,-11.1481985439209,
-11.0678135060188,-10.9874122031781,-10.9750258646012,-10.8946239524111,
-10.8142373647188,-10.7336745609209,-10.6532917024683,-10.5726389259978,
-10.4919861495273),.UNSPECIFIED.);
#631=B_SPLINE_CURVE_WITH_KNOTS('',3,(#77556,#77557,#77558,#77559,#77560,
#77561,#77562,#77563,#77564,#77565,#77566,#77567,#77568,#77569,#77570,#77571,
#77572,#77573,#77574,#77575,#77576,#77577,#77578,#77579,#77580,#77581,#77582,
#77583,#77584,#77585,#77586,#77587,#77588,#77589,#77590,#77591,#77592,#77593,
#77594,#77595,#77596,#77597,#77598,#77599,#77600,#77601,#77602,#77603,#77604,
#77605,#77606,#77607,#77608,#77609,#77610,#77611,#77612,#77613,#77614,#77615,
#77616,#77617,#77618,#77619,#77620,#77621,#77622,#77623,#77624,#77625,#77626,
#77627,#77628,#77629,#77630,#77631,#77632,#77633),.UNSPECIFIED.,.F.,.F.,
(4,2,2,2,2,2,2,2,2,2,2,2,2,2,2,2,2,2,2,2,2,2,2,2,2,2,2,2,2,2,2,2,2,2,2,
2,2,2,4),(5.98638844770362E-5,0.112872266003416,0.17427999276801,0.26938684905027,
0.322521957986195,0.353461345058414,0.432508794039687,0.525454262701712,
0.642595895792396,0.701573004104969,0.778521202305748,0.86855015668362,
1.00913121847656,1.05572572809319,1.13026329894176,1.22281910204197,1.3487438846434,
1.40270123548857,1.47894075605843,1.568867084826,1.70711663583873,1.75540521681487,
1.83515681926088,1.92042700563513,2.05966626718135,2.10632096964438,2.17059611351698,
2.24074969883762,2.27086609193784,2.40513588310623,2.45508146207408,2.52395462171003,
2.59276459723876,2.62283023188887,2.7517686900946,2.789975913623,2.82944959587034,
2.91095381420802,2.95510205588621),.UNSPECIFIED.);
#632=B_SPLINE_CURVE_WITH_KNOTS('',3,(#77637,#77638,#77639,#77640,#77641,
#77642,#77643,#77644,#77645,#77646,#77647,#77648,#77649,#77650,#77651,#77652,
#77653,#77654,#77655,#77656,#77657,#77658,#77659,#77660,#77661,#77662,#77663,
#77664,#77665,#77666,#77667,#77668,#77669,#77670,#77671,#77672,#77673,#77674,
#77675,#77676,#77677,#77678,#77679,#77680,#77681,#77682,#77683,#77684,#77685,
#77686,#77687,#77688,#77689,#77690,#77691,#77692,#77693,#77694,#77695,#77696,
#77697,#77698,#77699,#77700,#77701,#77702,#77703,#77704,#77705,#77706,#77707,
#77708,#77709,#77710,#77711,#77712,#77713,#77714,#77715,#77716,#77717,#77718,
#77719,#77720,#77721,#77722,#77723,#77724,#77725,#77726,#77727,#77728,#77729,
#77730,#77731,#77732,#77733,#77734,#77735,#77736,#77737,#77738,#77739,#77740,
#77741,#77742,#77743,#77744,#77745,#77746,#77747,#77748,#77749,#77750,#77751,
#77752,#77753,#77754,#77755,#77756,#77757,#77758,#77759,#77760,#77761,#77762,
#77763,#77764,#77765,#77766,#77767,#77768,#77769,#77770,#77771,#77772,#77773,
#77774,#77775,#77776,#77777,#77778,#77779,#77780,#77781,#77782,#77783,#77784,
#77785,#77786,#77787,#77788,#77789,#77790,#77791,#77792,#77793,#77794,#77795,
#77796,#77797,#77798,#77799,#77800,#77801,#77802,#77803,#77804,#77805,#77806,
#77807,#77808,#77809,#77810,#77811,#77812,#77813,#77814,#77815,#77816,#77817,
#77818,#77819,#77820,#77821,#77822,#77823,#77824,#77825,#77826,#77827,#77828,
#77829,#77830,#77831,#77832,#77833,#77834,#77835,#77836,#77837,#77838,#77839,
#77840,#77841,#77842,#77843,#77844,#77845,#77846,#77847,#77848,#77849,#77850,
#77851,#77852,#77853,#77854,#77855,#77856,#77857,#77858,#77859,#77860,#77861,
#77862,#77863,#77864,#77865,#77866,#77867,#77868,#77869,#77870,#77871),
 .UNSPECIFIED.,.F.,.F.,(4,3,3,3,3,3,3,3,3,3,3,3,3,3,3,3,3,3,3,3,3,3,3,3,
3,3,3,3,3,3,3,3,3,3,3,3,3,3,3,3,3,3,3,3,3,3,3,3,3,3,3,3,3,3,3,3,3,3,3,3,
3,3,3,3,3,3,3,3,3,3,3,3,3,3,3,3,3,3,4),(2.02057256326897,2.10082259985238,
2.1810574358235,2.26129496682187,2.34152807110776,2.4217816632337,2.49432406013665,
2.57472542136099,2.65511153505957,2.73963086933567,2.82001443873895,2.90039883353079,
2.98079952696405,2.99318887216398,3.07358729627662,3.15397039737693,3.23849121908052,
3.3188716377365,3.39925284699051,3.47965032437132,3.4920536841913,3.57245925188446,
3.6528496035864,3.73736682674446,3.8177546421867,3.89814326818861,3.97854814754071,
3.99091849621863,4.071318441516,4.15170309472865,4.23622314810798,4.31660517019189,
4.39698799400358,4.47738709226745,4.48978330824596,4.57018642790357,4.65057429574128,
4.73509275187428,4.81547803548217,4.89586412354026,4.97626647102544,4.98864812027329,
5.06904985871735,5.14943632904741,5.23395547986071,5.31433934859764,5.39472402163805,
5.47512496207277,5.48751293230062,5.56791508317406,5.64830197006663,5.73282091363196,
5.81320520230256,5.89359029470323,5.97399165126986,5.98637774432795,6.06677988419513,
6.14716676060536,6.23168570954284,6.3120699892127,6.39245507316294,6.4728564221019,
6.48524255635528,6.56564459930079,6.64603137725135,6.73055037503416,6.81093455404784,
6.89131953699836,6.97172078503834,6.98410736838261,7.06450950077892,7.14489636941888,
7.22941532216664,7.30979959344878,7.39018466883242,7.47058600900235,7.48297218040994,
7.56803809318229,7.59229499831558),.UNSPECIFIED.);
#633=B_SPLINE_CURVE_WITH_KNOTS('',3,(#77872,#77873,#77874,#77875,#77876,
#77877,#77878,#77879,#77880,#77881),.UNSPECIFIED.,.F.,.F.,(4,2,2,2,4),(-8.82240336587914,
-8.75464221200688,-8.71131988181848,-8.5760612850891,-8.57259242800733),
 .UNSPECIFIED.);
#634=B_SPLINE_CURVE_WITH_KNOTS('',3,(#77883,#77884,#77885,#77886,#77887,
#77888,#77889,#77890,#77891,#77892,#77893,#77894,#77895,#77896,#77897,#77898,
#77899,#77900,#77901,#77902,#77903,#77904,#77905,#77906,#77907,#77908,#77909,
#77910,#77911,#77912,#77913,#77914,#77915,#77916,#77917,#77918,#77919,#77920,
#77921,#77922,#77923,#77924,#77925,#77926,#77927,#77928,#77929,#77930,#77931,
#77932,#77933,#77934,#77935,#77936,#77937,#77938,#77939,#77940,#77941,#77942,
#77943,#77944,#77945,#77946,#77947,#77948,#77949,#77950,#77951,#77952,#77953,
#77954,#77955,#77956,#77957,#77958,#77959,#77960,#77961,#77962,#77963,#77964,
#77965,#77966,#77967,#77968,#77969,#77970,#77971,#77972,#77973,#77974,#77975,
#77976,#77977,#77978,#77979,#77980,#77981,#77982,#77983,#77984,#77985,#77986,
#77987,#77988,#77989,#77990,#77991,#77992,#77993,#77994,#77995,#77996,#77997,
#77998,#77999,#78000,#78001,#78002,#78003,#78004),.UNSPECIFIED.,.F.,.F.,
(4,2,2,2,2,2,2,2,2,2,2,2,2,2,2,2,2,2,2,2,2,2,2,2,2,2,2,2,2,2,2,2,2,2,2,
2,2,2,2,2,2,2,2,2,2,2,2,2,2,2,2,2,2,2,2,2,2,2,2,2,4),(-8.57259242800733,
-8.53729965094587,-8.43520820880102,-8.37593118628754,-8.25380929012716,
-8.19747433468778,-8.12105231428395,-8.03137279657271,-7.95767040886687,
-7.88831042464076,-7.8428969754146,-7.76891951015125,-7.67588154933796,
-7.55225135353314,-7.49680633626482,-7.42121497421589,-7.33369877963596,
-7.26237150015515,-7.18572502564829,-7.16444605238263,-7.12621153300411,
-7.04331970134402,-6.96717415540716,-6.88292187172238,-6.80598449312008,
-6.76381982603942,-6.6840742636716,-6.62479665950097,-6.50284700212666,
-6.44640880715542,-6.36989366829346,-6.28026205719654,-6.20653855628664,
-6.13747365600876,-6.09190808188494,-6.01749692196664,-5.92495083604497,
-5.80074844958054,-5.76104140745546,-5.7222491520745,-5.64011050399418,
-5.58055857778821,-5.50752992928515,-5.4149653039514,-5.3768796683347,-5.29357358862069,
-5.21665981691337,-5.11823587924998,-5.04848179424069,-4.94719446510772,
-4.86795408371006,-4.79510534412133,-4.71155856194044,-4.67307790121227,
-4.58820042118712,-4.51396150418326,-4.41127049403132,-4.34748944243495,
-4.29183640423953,-4.1685528105975,-4.16151590151851),.UNSPECIFIED.);
#635=B_SPLINE_CURVE_WITH_KNOTS('',3,(#78006,#78007,#78008,#78009,#78010,
#78011,#78012,#78013,#78014,#78015,#78016,#78017,#78018,#78019,#78020,#78021,
#78022,#78023,#78024),.UNSPECIFIED.,.F.,.F.,(4,3,3,3,3,3,4),(-10.4919861495273,
-10.4761610525739,-10.3958161762845,-10.3154846813862,-10.2351643727366,
-10.1548434234609,-10.1362407613902),.UNSPECIFIED.);
#636=B_SPLINE_CURVE_WITH_KNOTS('',3,(#78025,#78026,#78027,#78028,#78029,
#78030,#78031,#78032,#78033,#78034,#78035,#78036,#78037,#78038,#78039,#78040,
#78041,#78042,#78043,#78044,#78045,#78046,#78047,#78048,#78049,#78050,#78051,
#78052,#78053,#78054,#78055,#78056,#78057,#78058,#78059,#78060,#78061,#78062,
#78063,#78064,#78065,#78066,#78067,#78068,#78069,#78070,#78071,#78072,#78073,
#78074,#78075,#78076,#78077,#78078,#78079,#78080,#78081,#78082,#78083,#78084,
#78085,#78086,#78087,#78088,#78089,#78090,#78091,#78092,#78093,#78094,#78095,
#78096,#78097,#78098,#78099,#78100,#78101,#78102,#78103,#78104,#78105,#78106,
#78107,#78108,#78109,#78110,#78111,#78112,#78113,#78114,#78115,#78116,#78117,
#78118,#78119,#78120,#78121,#78122,#78123,#78124,#78125,#78126,#78127,#78128,
#78129,#78130,#78131,#78132,#78133,#78134,#78135,#78136,#78137,#78138,#78139,
#78140,#78141,#78142),.UNSPECIFIED.,.F.,.F.,(4,2,2,2,2,2,2,2,2,2,2,2,2,
2,2,2,2,2,2,2,2,2,2,2,2,2,2,2,2,2,2,2,2,2,2,2,2,2,2,2,2,2,2,2,2,2,2,2,2,
2,2,2,2,2,2,2,2,2,4),(2.95510205588621,2.97035363036219,3.10736320582023,
3.15609175226186,3.22339274075777,3.29265531967367,3.32273466702341,3.45362622282612,
3.50519056950469,3.55844947430104,3.67978864312186,3.73906508705386,3.81875203655083,
3.86102586139961,3.87884392100704,3.93214053233551,4.02242288404177,4.09868923957733,
4.1816464942187,4.21985009140902,4.31262834795997,4.38621338445752,4.47615734771452,
4.55206305528035,4.6078319546552,4.73090708109962,4.76095566059319,4.79532696224168,
4.87702784019752,4.91627446572275,4.95491957120443,5.08240563930163,5.17462078794299,
5.25322582800885,5.31224286836276,5.43007617379252,5.5273886842897,5.60261488919278,
5.65768693245673,5.78196344984821,5.81201248750418,5.88290559383789,5.95079825585252,
5.99991511847723,6.1360309526222,6.1661595287973,6.23675661414532,6.29956647113604,
6.34583513868145,6.48478600973137,6.51486821003581,6.5843340908246,6.65092249030151,
6.69922257791544,6.79604535805604,6.86019450396185,6.96870586689564,7.00937776730152,
7.11659720232867),.UNSPECIFIED.);
#637=B_SPLINE_CURVE_WITH_KNOTS('',3,(#78145,#78146,#78147,#78148,#78149,
#78150,#78151,#78152,#78153,#78154,#78155,#78156),.UNSPECIFIED.,.F.,.F.,
(4,1,1,1,1,1,1,1,1,4),(17.9333477466581,18.3401503700936,18.8390151821209,
19.3378799941482,19.8367448061755,20.3356096182029,20.8344744302302,21.3333392422575,
21.8322040542849,21.9911485751285),.UNSPECIFIED.);
#638=B_SPLINE_CURVE_WITH_KNOTS('',3,(#78157,#78158,#78159,#78160,#78161,
#78162,#78163,#78164),.UNSPECIFIED.,.F.,.F.,(4,1,1,1,1,4),(21.9911485751285,
22.3310688663122,22.8299336783395,23.3287984903668,23.8276633023942,24.2164828558523),
 .UNSPECIFIED.);
#639=B_SPLINE_CURVE_WITH_KNOTS('',3,(#78166,#78167,#78168,#78169,#78170,
#78171,#78172,#78173,#78174,#78175,#78176,#78177,#78178,#78179,#78180,#78181,
#78182,#78183,#78184,#78185,#78186,#78187,#78188,#78189,#78190,#78191,#78192,
#78193,#78194,#78195,#78196,#78197,#78198,#78199,#78200,#78201,#78202,#78203,
#78204,#78205,#78206,#78207,#78208,#78209,#78210,#78211,#78212,#78213,#78214,
#78215,#78216,#78217,#78218,#78219,#78220,#78221,#78222,#78223,#78224,#78225,
#78226,#78227,#78228,#78229,#78230,#78231,#78232,#78233,#78234,#78235,#78236,
#78237,#78238,#78239,#78240,#78241,#78242,#78243,#78244,#78245,#78246,#78247,
#78248,#78249,#78250,#78251,#78252,#78253,#78254,#78255,#78256,#78257,#78258,
#78259),.UNSPECIFIED.,.F.,.F.,(4,3,3,3,3,3,3,3,3,3,3,3,3,3,3,3,3,3,3,3,
3,3,3,3,3,3,3,3,3,3,3,4),(21.9911485751285,22.068343866769,22.1464305423893,
22.2236230042503,22.3021567867503,22.3806905692502,22.4581826086602,22.5356603640975,
22.6131294154855,22.6906046742007,22.7680796462036,22.8455711833453,22.8795553812775,
22.9570474121103,23.0345251588809,23.1119942015404,23.1894694515018,23.2669444147519,
23.3444359431996,23.3784201933048,23.4559122253536,23.5333899733441,23.6108590172257,
23.6883342683997,23.7658092328552,23.8433007624899,23.8772850053322,23.9547763215957,
24.0322561410154,24.1097256822953,24.1871964328171,24.2164947951915),
 .UNSPECIFIED.);
#640=B_SPLINE_CURVE_WITH_KNOTS('',3,(#78260,#78261,#78262,#78263,#78264,
#78265,#78266,#78267,#78268,#78269,#78270,#78271),.UNSPECIFIED.,.F.,.F.,
(4,1,1,1,1,1,1,1,1,4),(17.9333372203403,18.3897720730315,18.8886368850589,
19.3875016970862,19.8863665091135,20.3852313211409,20.8840961331682,21.3829609451955,
21.8818257572228,21.9911485751285),.UNSPECIFIED.);
#641=B_SPLINE_CURVE_WITH_KNOTS('',3,(#78817,#78818,#78819,#78820,#78821,
#78822,#78823,#78824,#78825,#78826,#78827,#78828,#78829,#78830,#78831,#78832,
#78833,#78834,#78835,#78836,#78837,#78838,#78839,#78840,#78841,#78842,#78843,
#78844,#78845,#78846,#78847,#78848,#78849,#78850,#78851,#78852,#78853,#78854,
#78855,#78856,#78857,#78858,#78859,#78860,#78861,#78862,#78863,#78864,#78865,
#78866,#78867,#78868,#78869,#78870,#78871,#78872,#78873,#78874,#78875,#78876,
#78877,#78878,#78879,#78880,#78881,#78882,#78883,#78884,#78885,#78886,#78887,
#78888,#78889,#78890,#78891,#78892,#78893,#78894,#78895,#78896,#78897,#78898,
#78899,#78900,#78901,#78902,#78903,#78904,#78905,#78906,#78907,#78908,#78909,
#78910,#78911,#78912,#78913,#78914,#78915,#78916,#78917,#78918,#78919,#78920,
#78921,#78922,#78923,#78924,#78925),.UNSPECIFIED.,.F.,.F.,(4,3,3,3,3,3,
3,3,3,3,3,3,3,3,3,3,3,3,3,3,3,3,3,3,3,3,3,3,3,3,3,3,3,3,3,3,4),(0.,0.0625522493162699,
0.125874299720649,0.189091179003679,0.251402665927997,0.304861832460781,
0.312371519783548,0.319581198043962,0.381443894429711,0.400771352782656,
0.462797545190397,0.524803898749766,0.586273327225432,0.612528497889583,
0.622823345007737,0.683558995678567,0.743895619283012,0.78830142952157,
0.848926514486215,0.905948440174609,0.913190739602521,0.920001699659024,
0.979766588587133,1.0391809686788,1.09912111202513,1.15906125537146,1.16229775674676,
1.19633653842214,1.2080220062924,1.26652171470092,1.32480529034897,1.36956433288647,
1.37830538556316,1.43585682539719,1.49260862883067,1.52200397117569,1.53973642054051),
 .UNSPECIFIED.);
#642=B_SPLINE_CURVE_WITH_KNOTS('',3,(#78926,#78927,#78928,#78929,#78930,
#78931,#78932,#78933,#78934,#78935,#78936,#78937,#78938,#78939,#78940,#78941,
#78942,#78943,#78944,#78945,#78946,#78947,#78948,#78949,#78950,#78951,#78952,
#78953,#78954,#78955,#78956,#78957,#78958,#78959,#78960,#78961,#78962,#78963,
#78964,#78965,#78966,#78967,#78968,#78969,#78970,#78971,#78972,#78973,#78974,
#78975,#78976,#78977,#78978,#78979,#78980,#78981,#78982,#78983,#78984,#78985,
#78986,#78987,#78988,#78989,#78990,#78991,#78992,#78993,#78994,#78995,#78996,
#78997,#78998,#78999,#79000,#79001,#79002,#79003,#79004,#79005,#79006,#79007,
#79008,#79009,#79010,#79011,#79012,#79013,#79014,#79015,#79016,#79017,#79018,
#79019,#79020,#79021,#79022,#79023,#79024,#79025,#79026,#79027,#79028,#79029,
#79030,#79031,#79032,#79033,#79034),.UNSPECIFIED.,.F.,.F.,(4,3,3,3,3,3,
3,3,3,3,3,3,3,3,3,3,3,3,3,3,3,3,3,3,3,3,3,3,3,3,3,3,3,3,3,3,4),(8.90323594776316E-15,
0.0558396431186415,0.113060832821276,0.170735773687653,0.22842886876104,
0.270961174530826,0.278040176691813,0.336849357119395,0.358599321240352,
0.416882186454614,0.475694476083339,0.534694628727055,0.561661453860504,
0.569038253759618,0.628817425890107,0.689165334561057,0.730812179732138,
0.790964330629484,0.850856995814571,0.860790218443922,0.921184370420933,
0.98262723491039,1.04424837715007,1.10546557987407,1.11637421967215,1.14126170877834,
1.15446357064426,1.16482862059503,1.22654809014449,1.28893143939649,1.32131544761034,
1.33677901974891,1.35296500609063,1.3818151014266,1.44819457339889,1.51457404537117,
1.53495742839389),.UNSPECIFIED.);
#643=B_SPLINE_CURVE_WITH_KNOTS('',3,(#79035,#79036,#79037,#79038),
 .UNSPECIFIED.,.F.,.F.,(4,4),(-0.00103132579068994,0.),.UNSPECIFIED.);
#644=B_SPLINE_CURVE_WITH_KNOTS('',3,(#79571,#79572,#79573,#79574,#79575,
#79576,#79577,#79578,#79579,#79580,#79581,#79582,#79583,#79584,#79585,#79586,
#79587,#79588,#79589,#79590,#79591,#79592,#79593,#79594,#79595,#79596,#79597,
#79598,#79599,#79600,#79601,#79602,#79603,#79604,#79605,#79606,#79607,#79608,
#79609,#79610,#79611,#79612,#79613,#79614,#79615,#79616,#79617,#79618,#79619,
#79620,#79621,#79622,#79623,#79624,#79625,#79626,#79627,#79628,#79629,#79630,
#79631,#79632,#79633,#79634,#79635,#79636,#79637,#79638,#79639,#79640,#79641,
#79642,#79643,#79644,#79645,#79646,#79647,#79648,#79649,#79650,#79651,#79652,
#79653,#79654,#79655,#79656,#79657,#79658,#79659,#79660,#79661,#79662,#79663,
#79664,#79665,#79666,#79667,#79668,#79669,#79670,#79671,#79672,#79673,#79674,
#79675,#79676,#79677,#79678,#79679,#79680,#79681,#79682),.UNSPECIFIED.,
 .F.,.F.,(4,3,3,3,3,3,3,3,3,3,3,3,3,3,3,3,3,3,3,3,3,3,3,3,3,3,3,3,3,3,3,
3,3,3,3,3,3,4),(0.,0.0558126623480815,0.11299849537912,0.170655392453315,
0.228379672699063,0.260934534205675,0.270961389638314,0.278040383899749,
0.336849596436437,0.358599321240349,0.416882127265502,0.475694380857889,
0.534694534057781,0.561660852466186,0.569038190842159,0.628817317058425,
0.689165218184891,0.730812179732113,0.790889891999659,0.831575432958716,
0.850857020400834,0.862299587265291,0.925818245366998,0.987287649254916,
1.05183093446352,1.11300183721899,1.11637421967212,1.15284176874186,1.16300105616543,
1.22467697484842,1.28717878211968,1.33420062353113,1.34388635491295,1.35388326449023,
1.4171375655674,1.48044101623512,1.51457404537113,1.53495742827616),
 .UNSPECIFIED.);
#645=B_SPLINE_CURVE_WITH_KNOTS('',3,(#79683,#79684,#79685,#79686,#79687,
#79688,#79689,#79690,#79691,#79692,#79693,#79694,#79695,#79696,#79697,#79698,
#79699,#79700,#79701,#79702,#79703,#79704,#79705,#79706,#79707,#79708,#79709,
#79710,#79711,#79712,#79713,#79714,#79715,#79716,#79717,#79718,#79719,#79720,
#79721,#79722,#79723,#79724,#79725,#79726,#79727,#79728,#79729,#79730,#79731,
#79732,#79733,#79734,#79735,#79736,#79737,#79738,#79739,#79740,#79741,#79742,
#79743,#79744,#79745,#79746,#79747,#79748,#79749,#79750,#79751,#79752,#79753,
#79754,#79755,#79756,#79757,#79758,#79759,#79760,#79761,#79762,#79763,#79764,
#79765,#79766,#79767,#79768,#79769,#79770,#79771,#79772,#79773,#79774,#79775,
#79776,#79777,#79778,#79779,#79780,#79781,#79782,#79783,#79784,#79785,#79786,
#79787,#79788,#79789,#79790,#79791,#79792,#79793,#79794,#79795,#79796,#79797,
#79798,#79799,#79800,#79801,#79802,#79803),.UNSPECIFIED.,.F.,.F.,(4,3,3,
3,3,3,3,3,3,3,3,3,3,3,3,3,3,3,3,3,3,3,3,3,3,3,3,3,3,3,3,3,3,3,3,3,3,3,3,
3,4),(0.,0.0627294749945631,0.125990888525662,0.189264306022852,0.251655622871188,
0.288934555349053,0.304522706022472,0.312082966773186,0.319531623860181,
0.345855736736584,0.400771352782651,0.462797530992162,0.52480388993571,
0.586273333423623,0.604978113100597,0.616083231103068,0.625115386768979,
0.685851984651888,0.746175682300948,0.788301429521589,0.848926515362853,
0.905948442014449,0.913190741906353,0.936167503816501,0.995683676192635,
1.05501285749589,1.11339979822315,1.15906127253955,1.16229775674677,1.18477939514858,
1.1980518199991,1.20870860039415,1.26720629382776,1.32564380364759,1.35222581692638,
1.37013678512747,1.38085187373706,1.43838931773557,1.49511977718729,1.52200397117572,
1.53973642054053),.UNSPECIFIED.);
#896=SHAPE_REPRESENTATION_RELATIONSHIP('SRR','None',#105864,#908);
#908=ADVANCED_BREP_SHAPE_REPRESENTATION('',(#932),#105799);
#920=STYLED_ITEM('',(#105931),#932);
#932=MANIFOLD_SOLID_BREP('Body1',#7207);
#973=FACE_BOUND('',#1534,.T.);
#974=FACE_BOUND('',#1535,.T.);
#975=FACE_BOUND('',#1536,.T.);
#976=FACE_BOUND('',#1537,.T.);
#977=FACE_BOUND('',#1538,.T.);
#978=FACE_BOUND('',#1546,.T.);
#979=FACE_BOUND('',#1547,.T.);
#980=FACE_BOUND('',#1548,.T.);
#981=FACE_BOUND('',#1549,.T.);
#982=FACE_BOUND('',#1550,.T.);
#1030=PLANE('',#7571);
#1031=PLANE('',#7578);
#1032=PLANE('',#7579);
#1033=PLANE('',#7580);
#1034=PLANE('',#7581);
#1035=PLANE('',#7582);
#1201=FACE_OUTER_BOUND('',#1507,.T.);
#1202=FACE_OUTER_BOUND('',#1508,.T.);
#1203=FACE_OUTER_BOUND('',#1509,.T.);
#1204=FACE_OUTER_BOUND('',#1510,.T.);
#1205=FACE_OUTER_BOUND('',#1511,.T.);
#1206=FACE_OUTER_BOUND('',#1512,.T.);
#1207=FACE_OUTER_BOUND('',#1513,.T.);
#1208=FACE_OUTER_BOUND('',#1514,.T.);
#1209=FACE_OUTER_BOUND('',#1515,.T.);
#1210=FACE_OUTER_BOUND('',#1516,.T.);
#1211=FACE_OUTER_BOUND('',#1517,.T.);
#1212=FACE_OUTER_BOUND('',#1518,.T.);
#1213=FACE_OUTER_BOUND('',#1519,.T.);
#1214=FACE_OUTER_BOUND('',#1520,.T.);
#1215=FACE_OUTER_BOUND('',#1521,.T.);
#1216=FACE_OUTER_BOUND('',#1522,.T.);
#1217=FACE_OUTER_BOUND('',#1523,.T.);
#1218=FACE_OUTER_BOUND('',#1524,.T.);
#1219=FACE_OUTER_BOUND('',#1525,.T.);
#1220=FACE_OUTER_BOUND('',#1526,.T.);
#1221=FACE_OUTER_BOUND('',#1527,.T.);
#1222=FACE_OUTER_BOUND('',#1528,.T.);
#1223=FACE_OUTER_BOUND('',#1529,.T.);
#1224=FACE_OUTER_BOUND('',#1530,.T.);
#1225=FACE_OUTER_BOUND('',#1531,.T.);
#1226=FACE_OUTER_BOUND('',#1532,.T.);
#1227=FACE_OUTER_BOUND('',#1533,.T.);
#1228=FACE_OUTER_BOUND('',#1539,.T.);
#1229=FACE_OUTER_BOUND('',#1540,.T.);
#1230=FACE_OUTER_BOUND('',#1541,.T.);
#1231=FACE_OUTER_BOUND('',#1542,.T.);
#1232=FACE_OUTER_BOUND('',#1543,.T.);
#1233=FACE_OUTER_BOUND('',#1544,.T.);
#1234=FACE_OUTER_BOUND('',#1545,.T.);
#1507=EDGE_LOOP('',(#5719,#5720,#5721,#5722));
#1508=EDGE_LOOP('',(#5723,#5724,#5725,#5726,#5727,#5728));
#1509=EDGE_LOOP('',(#5729,#5730,#5731,#5732,#5733,#5734));
#1510=EDGE_LOOP('',(#5735,#5736,#5737,#5738,#5739,#5740));
#1511=EDGE_LOOP('',(#5741,#5742,#5743,#5744,#5745,#5746));
#1512=EDGE_LOOP('',(#5747,#5748,#5749,#5750,#5751,#5752));
#1513=EDGE_LOOP('',(#5753,#5754,#5755,#5756,#5757,#5758));
#1514=EDGE_LOOP('',(#5759,#5760,#5761,#5762,#5763,#5764));
#1515=EDGE_LOOP('',(#5765,#5766,#5767,#5768,#5769,#5770));
#1516=EDGE_LOOP('',(#5771,#5772,#5773,#5774,#5775,#5776));
#1517=EDGE_LOOP('',(#5777,#5778,#5779,#5780));
#1518=EDGE_LOOP('',(#5781,#5782,#5783,#5784));
#1519=EDGE_LOOP('',(#5785,#5786,#5787,#5788,#5789,#5790));
#1520=EDGE_LOOP('',(#5791,#5792,#5793,#5794,#5795,#5796));
#1521=EDGE_LOOP('',(#5797,#5798,#5799,#5800,#5801));
#1522=EDGE_LOOP('',(#5802,#5803,#5804,#5805,#5806));
#1523=EDGE_LOOP('',(#5807,#5808,#5809,#5810,#5811,#5812));
#1524=EDGE_LOOP('',(#5813,#5814,#5815,#5816,#5817));
#1525=EDGE_LOOP('',(#5818,#5819,#5820,#5821,#5822,#5823));
#1526=EDGE_LOOP('',(#5824,#5825,#5826,#5827,#5828));
#1527=EDGE_LOOP('',(#5829,#5830,#5831,#5832,#5833));
#1528=EDGE_LOOP('',(#5834,#5835,#5836,#5837,#5838,#5839));
#1529=EDGE_LOOP('',(#5840,#5841,#5842,#5843));
#1530=EDGE_LOOP('',(#5844,#5845,#5846,#5847));
#1531=EDGE_LOOP('',(#5848,#5849,#5850,#5851,#5852,#5853,#5854,#5855,#5856,
#5857,#5858,#5859,#5860,#5861,#5862,#5863,#5864,#5865,#5866,#5867,#5868,
#5869,#5870,#5871,#5872,#5873,#5874,#5875,#5876,#5877,#5878,#5879,#5880,
#5881,#5882,#5883,#5884,#5885,#5886,#5887,#5888,#5889));
#1532=EDGE_LOOP('',(#5890,#5891,#5892,#5893,#5894,#5895,#5896,#5897,#5898,
#5899,#5900,#5901,#5902,#5903,#5904,#5905,#5906,#5907,#5908,#5909,#5910,
#5911,#5912,#5913,#5914,#5915,#5916,#5917,#5918,#5919,#5920,#5921,#5922,
#5923,#5924,#5925,#5926,#5927,#5928,#5929));
#1533=EDGE_LOOP('',(#5930,#5931,#5932,#5933));
#1534=EDGE_LOOP('',(#5934));
#1535=EDGE_LOOP('',(#5935));
#1536=EDGE_LOOP('',(#5936));
#1537=EDGE_LOOP('',(#5937));
#1538=EDGE_LOOP('',(#5938,#5939,#5940,#5941));
#1539=EDGE_LOOP('',(#5942,#5943,#5944,#5945));
#1540=EDGE_LOOP('',(#5946,#5947,#5948,#5949));
#1541=EDGE_LOOP('',(#5950,#5951,#5952,#5953));
#1542=EDGE_LOOP('',(#5954,#5955,#5956,#5957));
#1543=EDGE_LOOP('',(#5958,#5959,#5960,#5961));
#1544=EDGE_LOOP('',(#5962,#5963,#5964,#5965));
#1545=EDGE_LOOP('',(#5966,#5967,#5968,#5969));
#1546=EDGE_LOOP('',(#5970));
#1547=EDGE_LOOP('',(#5971));
#1548=EDGE_LOOP('',(#5972,#5973,#5974,#5975,#5976));
#1549=EDGE_LOOP('',(#5977));
#1550=EDGE_LOOP('',(#5978));
#1815=LINE('',#71901,#2095);
#1816=LINE('',#71925,#2096);
#1817=LINE('',#72295,#2097);
#1818=LINE('',#72513,#2098);
#1819=LINE('',#72881,#2099);
#1820=LINE('',#73422,#2100);
#1821=LINE('',#73963,#2101);
#1822=LINE('',#74345,#2102);
#1823=LINE('',#74797,#2103);
#1824=LINE('',#75181,#2104);
#1825=LINE('',#75221,#2105);
#1826=LINE('',#75280,#2106);
#1827=LINE('',#75532,#2107);
#1828=LINE('',#75827,#2108);
#1829=LINE('',#76216,#2109);
#1830=LINE('',#76474,#2110);
#1831=LINE('',#76621,#2111);
#1832=LINE('',#77015,#2112);
#1833=LINE('',#77172,#2113);
#1834=LINE('',#77554,#2114);
#1835=LINE('',#78276,#2115);
#1836=LINE('',#78282,#2116);
#1837=LINE('',#79807,#2117);
#1838=LINE('',#79809,#2118);
#1839=LINE('',#79811,#2119);
#1840=LINE('',#79812,#2120);
#1841=LINE('',#79819,#2121);
#1842=LINE('',#79823,#2122);
#1843=LINE('',#79828,#2123);
#1844=LINE('',#79829,#2124);
#1845=LINE('',#79830,#2125);
#1846=LINE('',#79833,#2126);
#1847=LINE('',#79834,#2127);
#1848=LINE('',#79837,#2128);
#1849=LINE('',#79838,#2129);
#1850=LINE('',#79840,#2130);
#2095=VECTOR('',#8276,8.12525);
#2096=VECTOR('',#8281,8.12525);
#2097=VECTOR('',#8284,8.12525);
#2098=VECTOR('',#8287,8.12525);
#2099=VECTOR('',#8290,8.12525);
#2100=VECTOR('',#8293,8.12525);
#2101=VECTOR('',#8296,8.12525);
#2102=VECTOR('',#8299,8.12525);
#2103=VECTOR('',#8302,8.12525);
#2104=VECTOR('',#8305,8.12525);
#2105=VECTOR('',#8310,7.01125);
#2106=VECTOR('',#8315,7.01125);
#2107=VECTOR('',#8318,7.01125);
#2108=VECTOR('',#8321,7.01125);
#2109=VECTOR('',#8324,7.01125);
#2110=VECTOR('',#8327,7.01125);
#2111=VECTOR('',#8330,7.01125);
#2112=VECTOR('',#8333,7.01125);
#2113=VECTOR('',#8336,7.01125);
#2114=VECTOR('',#8339,7.01125);
#2115=VECTOR('',#8350,3.5);
#2116=VECTOR('',#8357,3.5);
#2117=VECTOR('',#8362,10.);
#2118=VECTOR('',#8363,10.);
#2119=VECTOR('',#8364,10.);
#2120=VECTOR('',#8365,10.);
#2121=VECTOR('',#8372,6.);
#2122=VECTOR('',#8377,6.);
#2123=VECTOR('',#8382,10.);
#2124=VECTOR('',#8383,10.);
#2125=VECTOR('',#8384,10.);
#2126=VECTOR('',#8387,10.);
#2127=VECTOR('',#8388,10.);
#2128=VECTOR('',#8391,10.);
#2129=VECTOR('',#8392,10.);
#2130=VECTOR('',#8395,10.);
#2277=CIRCLE('',#7540,8.12525);
#2278=CIRCLE('',#7550,8.12525);
#2279=CIRCLE('',#7552,7.01125);
#2280=CIRCLE('',#7562,7.01125);
#2281=CIRCLE('',#7566,3.5);
#2282=CIRCLE('',#7567,3.5);
#2283=CIRCLE('',#7569,3.5);
#2284=CIRCLE('',#7570,3.5);
#2285=CIRCLE('',#7572,6.);
#2286=CIRCLE('',#7573,6.);
#2287=CIRCLE('',#7575,6.);
#2288=CIRCLE('',#7577,6.);
#2859=VERTEX_POINT('',#71899);
#2860=VERTEX_POINT('',#71900);
#2861=VERTEX_POINT('',#71902);
#2862=VERTEX_POINT('',#71911);
#2863=VERTEX_POINT('',#71923);
#2864=VERTEX_POINT('',#71924);
#2865=VERTEX_POINT('',#71926);
#2866=VERTEX_POINT('',#72110);
#2867=VERTEX_POINT('',#72293);
#2868=VERTEX_POINT('',#72294);
#2869=VERTEX_POINT('',#72296);
#2870=VERTEX_POINT('',#72403);
#2871=VERTEX_POINT('',#72511);
#2872=VERTEX_POINT('',#72512);
#2873=VERTEX_POINT('',#72514);
#2874=VERTEX_POINT('',#72696);
#2875=VERTEX_POINT('',#72879);
#2876=VERTEX_POINT('',#72880);
#2877=VERTEX_POINT('',#72882);
#2878=VERTEX_POINT('',#73149);
#2879=VERTEX_POINT('',#73420);
#2880=VERTEX_POINT('',#73421);
#2881=VERTEX_POINT('',#73423);
#2882=VERTEX_POINT('',#73690);
#2883=VERTEX_POINT('',#73961);
#2884=VERTEX_POINT('',#73962);
#2885=VERTEX_POINT('',#73964);
#2886=VERTEX_POINT('',#74072);
#2887=VERTEX_POINT('',#74343);
#2888=VERTEX_POINT('',#74344);
#2889=VERTEX_POINT('',#74346);
#2890=VERTEX_POINT('',#74527);
#2891=VERTEX_POINT('',#74795);
#2892=VERTEX_POINT('',#74796);
#2893=VERTEX_POINT('',#74798);
#2894=VERTEX_POINT('',#74908);
#2895=VERTEX_POINT('',#75179);
#2896=VERTEX_POINT('',#75180);
#2897=VERTEX_POINT('',#75182);
#2898=VERTEX_POINT('',#75192);
#2899=VERTEX_POINT('',#75199);
#2900=VERTEX_POINT('',#75201);
#2901=VERTEX_POINT('',#75219);
#2902=VERTEX_POINT('',#75220);
#2903=VERTEX_POINT('',#75222);
#2904=VERTEX_POINT('',#75231);
#2905=VERTEX_POINT('',#75278);
#2906=VERTEX_POINT('',#75279);
#2907=VERTEX_POINT('',#75530);
#2908=VERTEX_POINT('',#75531);
#2909=VERTEX_POINT('',#75533);
#2910=VERTEX_POINT('',#75561);
#2911=VERTEX_POINT('',#75825);
#2912=VERTEX_POINT('',#75826);
#2913=VERTEX_POINT('',#75828);
#2914=VERTEX_POINT('',#76084);
#2915=VERTEX_POINT('',#76214);
#2916=VERTEX_POINT('',#76215);
#2917=VERTEX_POINT('',#76217);
#2918=VERTEX_POINT('',#76472);
#2919=VERTEX_POINT('',#76473);
#2920=VERTEX_POINT('',#76591);
#2921=VERTEX_POINT('',#76619);
#2922=VERTEX_POINT('',#76620);
#2923=VERTEX_POINT('',#76622);
#2924=VERTEX_POINT('',#76757);
#2925=VERTEX_POINT('',#77013);
#2926=VERTEX_POINT('',#77014);
#2927=VERTEX_POINT('',#77136);
#2928=VERTEX_POINT('',#77170);
#2929=VERTEX_POINT('',#77171);
#2930=VERTEX_POINT('',#77173);
#2931=VERTEX_POINT('',#77298);
#2932=VERTEX_POINT('',#77552);
#2933=VERTEX_POINT('',#77553);
#2934=VERTEX_POINT('',#77555);
#2935=VERTEX_POINT('',#77634);
#2936=VERTEX_POINT('',#77636);
#2937=VERTEX_POINT('',#78005);
#2938=VERTEX_POINT('',#78144);
#2939=VERTEX_POINT('',#78165);
#2940=VERTEX_POINT('',#78273);
#2941=VERTEX_POINT('',#78275);
#2942=VERTEX_POINT('',#78279);
#2943=VERTEX_POINT('',#78281);
#2944=VERTEX_POINT('',#78816);
#2945=VERTEX_POINT('',#79805);
#2946=VERTEX_POINT('',#79806);
#2947=VERTEX_POINT('',#79808);
#2948=VERTEX_POINT('',#79810);
#2949=VERTEX_POINT('',#79813);
#2950=VERTEX_POINT('',#79815);
#2951=VERTEX_POINT('',#79818);
#2952=VERTEX_POINT('',#79822);
#2953=VERTEX_POINT('',#79826);
#2954=VERTEX_POINT('',#79827);
#2955=VERTEX_POINT('',#79832);
#2956=VERTEX_POINT('',#79836);
#3904=EDGE_CURVE('',#2859,#2860,#1815,.T.);
#3905=EDGE_CURVE('',#2860,#2861,#564,.T.);
#3906=EDGE_CURVE('',#2862,#2861,#2277,.T.);
#3907=EDGE_CURVE('',#2859,#2862,#565,.T.);
#3908=EDGE_CURVE('',#2863,#2864,#1816,.T.);
#3909=EDGE_CURVE('',#2864,#2865,#566,.T.);
#3910=EDGE_CURVE('',#2865,#2860,#567,.T.);
#3911=EDGE_CURVE('',#2866,#2859,#568,.T.);
#3912=EDGE_CURVE('',#2863,#2866,#569,.T.);
#3913=EDGE_CURVE('',#2867,#2868,#1817,.T.);
#3914=EDGE_CURVE('',#2868,#2869,#570,.T.);
#3915=EDGE_CURVE('',#2869,#2864,#571,.T.);
#3916=EDGE_CURVE('',#2870,#2863,#572,.T.);
#3917=EDGE_CURVE('',#2867,#2870,#573,.T.);
#3918=EDGE_CURVE('',#2871,#2872,#1818,.T.);
#3919=EDGE_CURVE('',#2872,#2873,#574,.T.);
#3920=EDGE_CURVE('',#2873,#2868,#575,.T.);
#3921=EDGE_CURVE('',#2874,#2867,#576,.T.);
#3922=EDGE_CURVE('',#2871,#2874,#577,.T.);
#3923=EDGE_CURVE('',#2875,#2876,#1819,.T.);
#3924=EDGE_CURVE('',#2876,#2877,#578,.T.);
#3925=EDGE_CURVE('',#2877,#2872,#579,.T.);
#3926=EDGE_CURVE('',#2878,#2871,#580,.T.);
#3927=EDGE_CURVE('',#2875,#2878,#581,.T.);
#3928=EDGE_CURVE('',#2879,#2880,#1820,.T.);
#3929=EDGE_CURVE('',#2880,#2881,#582,.T.);
#3930=EDGE_CURVE('',#2881,#2876,#583,.T.);
#3931=EDGE_CURVE('',#2882,#2875,#584,.T.);
#3932=EDGE_CURVE('',#2879,#2882,#585,.T.);
#3933=EDGE_CURVE('',#2883,#2884,#1821,.T.);
#3934=EDGE_CURVE('',#2884,#2885,#586,.T.);
#3935=EDGE_CURVE('',#2885,#2880,#587,.T.);
#3936=EDGE_CURVE('',#2886,#2879,#588,.T.);
#3937=EDGE_CURVE('',#2883,#2886,#589,.T.);
#3938=EDGE_CURVE('',#2887,#2888,#1822,.T.);
#3939=EDGE_CURVE('',#2888,#2889,#590,.T.);
#3940=EDGE_CURVE('',#2889,#2884,#591,.T.);
#3941=EDGE_CURVE('',#2890,#2883,#592,.T.);
#3942=EDGE_CURVE('',#2887,#2890,#593,.T.);
#3943=EDGE_CURVE('',#2891,#2892,#1823,.T.);
#3944=EDGE_CURVE('',#2892,#2893,#594,.T.);
#3945=EDGE_CURVE('',#2893,#2888,#595,.T.);
#3946=EDGE_CURVE('',#2894,#2887,#596,.T.);
#3947=EDGE_CURVE('',#2891,#2894,#597,.T.);
#3948=EDGE_CURVE('',#2895,#2896,#1824,.T.);
#3949=EDGE_CURVE('',#2897,#2895,#598,.T.);
#3950=EDGE_CURVE('',#2898,#2897,#599,.T.);
#3951=EDGE_CURVE('',#2899,#2898,#2278,.T.);
#3952=EDGE_CURVE('',#2899,#2900,#600,.T.);
#3953=EDGE_CURVE('',#2900,#2896,#601,.T.);
#3954=EDGE_CURVE('',#2901,#2902,#1825,.T.);
#3955=EDGE_CURVE('',#2902,#2903,#602,.T.);
#3956=EDGE_CURVE('',#2904,#2903,#2279,.F.);
#3957=EDGE_CURVE('',#2904,#2901,#603,.T.);
#3958=EDGE_CURVE('',#2905,#2906,#1826,.T.);
#3959=EDGE_CURVE('',#2906,#2902,#604,.T.);
#3960=EDGE_CURVE('',#2901,#2905,#605,.T.);
#3961=EDGE_CURVE('',#2907,#2908,#1827,.T.);
#3962=EDGE_CURVE('',#2908,#2909,#606,.T.);
#3963=EDGE_CURVE('',#2909,#2906,#607,.T.);
#3964=EDGE_CURVE('',#2905,#2910,#608,.T.);
#3965=EDGE_CURVE('',#2910,#2907,#609,.T.);
#3966=EDGE_CURVE('',#2911,#2912,#1828,.T.);
#3967=EDGE_CURVE('',#2912,#2913,#610,.T.);
#3968=EDGE_CURVE('',#2913,#2908,#611,.T.);
#3969=EDGE_CURVE('',#2907,#2914,#612,.T.);
#3970=EDGE_CURVE('',#2914,#2911,#613,.T.);
#3971=EDGE_CURVE('',#2915,#2916,#1829,.T.);
#3972=EDGE_CURVE('',#2916,#2917,#614,.T.);
#3973=EDGE_CURVE('',#2917,#2912,#615,.T.);
#3974=EDGE_CURVE('',#2911,#2915,#616,.T.);
#3975=EDGE_CURVE('',#2918,#2919,#1830,.T.);
#3976=EDGE_CURVE('',#2919,#2916,#617,.T.);
#3977=EDGE_CURVE('',#2915,#2920,#618,.T.);
#3978=EDGE_CURVE('',#2920,#2918,#619,.T.);
#3979=EDGE_CURVE('',#2921,#2922,#1831,.T.);
#3980=EDGE_CURVE('',#2922,#2923,#620,.T.);
#3981=EDGE_CURVE('',#2923,#2919,#621,.T.);
#3982=EDGE_CURVE('',#2918,#2924,#622,.T.);
#3983=EDGE_CURVE('',#2924,#2921,#623,.T.);
#3984=EDGE_CURVE('',#2925,#2926,#1832,.T.);
#3985=EDGE_CURVE('',#2926,#2922,#624,.T.);
#3986=EDGE_CURVE('',#2921,#2927,#625,.T.);
#3987=EDGE_CURVE('',#2927,#2925,#626,.T.);
#3988=EDGE_CURVE('',#2928,#2929,#1833,.T.);
#3989=EDGE_CURVE('',#2929,#2930,#627,.T.);
#3990=EDGE_CURVE('',#2930,#2926,#628,.T.);
#3991=EDGE_CURVE('',#2925,#2931,#629,.T.);
#3992=EDGE_CURVE('',#2931,#2928,#630,.T.);
#3993=EDGE_CURVE('',#2932,#2933,#1834,.T.);
#3994=EDGE_CURVE('',#2932,#2934,#631,.F.);
#3995=EDGE_CURVE('',#2935,#2934,#2280,.T.);
#3996=EDGE_CURVE('',#2935,#2936,#632,.T.);
#3997=EDGE_CURVE('',#2936,#2933,#633,.T.);
#3998=EDGE_CURVE('',#2933,#2929,#634,.T.);
#3999=EDGE_CURVE('',#2928,#2937,#635,.T.);
#4000=EDGE_CURVE('',#2937,#2932,#636,.F.);
#4001=EDGE_CURVE('',#2896,#2938,#637,.T.);
#4002=EDGE_CURVE('',#2938,#2892,#638,.T.);
#4003=EDGE_CURVE('',#2939,#2891,#639,.T.);
#4004=EDGE_CURVE('',#2895,#2939,#640,.T.);
#4005=EDGE_CURVE('',#2940,#2940,#2281,.T.);
#4006=EDGE_CURVE('',#2940,#2941,#1835,.T.);
#4007=EDGE_CURVE('',#2941,#2941,#2282,.T.);
#4008=EDGE_CURVE('',#2942,#2942,#2283,.T.);
#4009=EDGE_CURVE('',#2942,#2943,#1836,.T.);
#4010=EDGE_CURVE('',#2943,#2943,#2284,.T.);
#4011=EDGE_CURVE('',#2861,#2944,#641,.T.);
#4012=EDGE_CURVE('',#2934,#2899,#642,.T.);
#4013=EDGE_CURVE('',#2944,#2904,#643,.T.);
#4014=EDGE_CURVE('',#2903,#2862,#644,.T.);
#4015=EDGE_CURVE('',#2898,#2935,#645,.T.);
#4016=EDGE_CURVE('',#2945,#2946,#1837,.T.);
#4017=EDGE_CURVE('',#2946,#2947,#1838,.T.);
#4018=EDGE_CURVE('',#2947,#2948,#1839,.T.);
#4019=EDGE_CURVE('',#2948,#2945,#1840,.F.);
#4020=EDGE_CURVE('',#2949,#2949,#2285,.T.);
#4021=EDGE_CURVE('',#2950,#2950,#2286,.T.);
#4022=EDGE_CURVE('',#2950,#2951,#1841,.T.);
#4023=EDGE_CURVE('',#2951,#2951,#2287,.T.);
#4024=EDGE_CURVE('',#2949,#2952,#1842,.T.);
#4025=EDGE_CURVE('',#2952,#2952,#2288,.T.);
#4026=EDGE_CURVE('',#2953,#2954,#1843,.F.);
#4027=EDGE_CURVE('',#2954,#2945,#1844,.T.);
#4028=EDGE_CURVE('',#2953,#2948,#1845,.F.);
#4029=EDGE_CURVE('',#2955,#2953,#1846,.T.);
#4030=EDGE_CURVE('',#2955,#2947,#1847,.T.);
#4031=EDGE_CURVE('',#2956,#2955,#1848,.T.);
#4032=EDGE_CURVE('',#2956,#2946,#1849,.T.);
#4033=EDGE_CURVE('',#2954,#2956,#1850,.T.);
#5719=ORIENTED_EDGE('',*,*,#3904,.T.);
#5720=ORIENTED_EDGE('',*,*,#3905,.T.);
#5721=ORIENTED_EDGE('',*,*,#3906,.F.);
#5722=ORIENTED_EDGE('',*,*,#3907,.F.);
#5723=ORIENTED_EDGE('',*,*,#3908,.T.);
#5724=ORIENTED_EDGE('',*,*,#3909,.T.);
#5725=ORIENTED_EDGE('',*,*,#3910,.T.);
#5726=ORIENTED_EDGE('',*,*,#3904,.F.);
#5727=ORIENTED_EDGE('',*,*,#3911,.F.);
#5728=ORIENTED_EDGE('',*,*,#3912,.F.);
#5729=ORIENTED_EDGE('',*,*,#3913,.T.);
#5730=ORIENTED_EDGE('',*,*,#3914,.T.);
#5731=ORIENTED_EDGE('',*,*,#3915,.T.);
#5732=ORIENTED_EDGE('',*,*,#3908,.F.);
#5733=ORIENTED_EDGE('',*,*,#3916,.F.);
#5734=ORIENTED_EDGE('',*,*,#3917,.F.);
#5735=ORIENTED_EDGE('',*,*,#3918,.T.);
#5736=ORIENTED_EDGE('',*,*,#3919,.T.);
#5737=ORIENTED_EDGE('',*,*,#3920,.T.);
#5738=ORIENTED_EDGE('',*,*,#3913,.F.);
#5739=ORIENTED_EDGE('',*,*,#3921,.F.);
#5740=ORIENTED_EDGE('',*,*,#3922,.F.);
#5741=ORIENTED_EDGE('',*,*,#3923,.T.);
#5742=ORIENTED_EDGE('',*,*,#3924,.T.);
#5743=ORIENTED_EDGE('',*,*,#3925,.T.);
#5744=ORIENTED_EDGE('',*,*,#3918,.F.);
#5745=ORIENTED_EDGE('',*,*,#3926,.F.);
#5746=ORIENTED_EDGE('',*,*,#3927,.F.);
#5747=ORIENTED_EDGE('',*,*,#3928,.T.);
#5748=ORIENTED_EDGE('',*,*,#3929,.T.);
#5749=ORIENTED_EDGE('',*,*,#3930,.T.);
#5750=ORIENTED_EDGE('',*,*,#3923,.F.);
#5751=ORIENTED_EDGE('',*,*,#3931,.F.);
#5752=ORIENTED_EDGE('',*,*,#3932,.F.);
#5753=ORIENTED_EDGE('',*,*,#3933,.T.);
#5754=ORIENTED_EDGE('',*,*,#3934,.T.);
#5755=ORIENTED_EDGE('',*,*,#3935,.T.);
#5756=ORIENTED_EDGE('',*,*,#3928,.F.);
#5757=ORIENTED_EDGE('',*,*,#3936,.F.);
#5758=ORIENTED_EDGE('',*,*,#3937,.F.);
#5759=ORIENTED_EDGE('',*,*,#3938,.T.);
#5760=ORIENTED_EDGE('',*,*,#3939,.T.);
#5761=ORIENTED_EDGE('',*,*,#3940,.T.);
#5762=ORIENTED_EDGE('',*,*,#3933,.F.);
#5763=ORIENTED_EDGE('',*,*,#3941,.F.);
#5764=ORIENTED_EDGE('',*,*,#3942,.F.);
#5765=ORIENTED_EDGE('',*,*,#3943,.T.);
#5766=ORIENTED_EDGE('',*,*,#3944,.T.);
#5767=ORIENTED_EDGE('',*,*,#3945,.T.);
#5768=ORIENTED_EDGE('',*,*,#3938,.F.);
#5769=ORIENTED_EDGE('',*,*,#3946,.F.);
#5770=ORIENTED_EDGE('',*,*,#3947,.F.);
#5771=ORIENTED_EDGE('',*,*,#3948,.F.);
#5772=ORIENTED_EDGE('',*,*,#3949,.F.);
#5773=ORIENTED_EDGE('',*,*,#3950,.F.);
#5774=ORIENTED_EDGE('',*,*,#3951,.F.);
#5775=ORIENTED_EDGE('',*,*,#3952,.T.);
#5776=ORIENTED_EDGE('',*,*,#3953,.T.);
#5777=ORIENTED_EDGE('',*,*,#3954,.T.);
#5778=ORIENTED_EDGE('',*,*,#3955,.T.);
#5779=ORIENTED_EDGE('',*,*,#3956,.F.);
#5780=ORIENTED_EDGE('',*,*,#3957,.T.);
#5781=ORIENTED_EDGE('',*,*,#3958,.T.);
#5782=ORIENTED_EDGE('',*,*,#3959,.T.);
#5783=ORIENTED_EDGE('',*,*,#3954,.F.);
#5784=ORIENTED_EDGE('',*,*,#3960,.T.);
#5785=ORIENTED_EDGE('',*,*,#3961,.T.);
#5786=ORIENTED_EDGE('',*,*,#3962,.T.);
#5787=ORIENTED_EDGE('',*,*,#3963,.T.);
#5788=ORIENTED_EDGE('',*,*,#3958,.F.);
#5789=ORIENTED_EDGE('',*,*,#3964,.T.);
#5790=ORIENTED_EDGE('',*,*,#3965,.T.);
#5791=ORIENTED_EDGE('',*,*,#3966,.T.);
#5792=ORIENTED_EDGE('',*,*,#3967,.T.);
#5793=ORIENTED_EDGE('',*,*,#3968,.T.);
#5794=ORIENTED_EDGE('',*,*,#3961,.F.);
#5795=ORIENTED_EDGE('',*,*,#3969,.T.);
#5796=ORIENTED_EDGE('',*,*,#3970,.T.);
#5797=ORIENTED_EDGE('',*,*,#3971,.T.);
#5798=ORIENTED_EDGE('',*,*,#3972,.T.);
#5799=ORIENTED_EDGE('',*,*,#3973,.T.);
#5800=ORIENTED_EDGE('',*,*,#3966,.F.);
#5801=ORIENTED_EDGE('',*,*,#3974,.T.);
#5802=ORIENTED_EDGE('',*,*,#3975,.T.);
#5803=ORIENTED_EDGE('',*,*,#3976,.T.);
#5804=ORIENTED_EDGE('',*,*,#3971,.F.);
#5805=ORIENTED_EDGE('',*,*,#3977,.T.);
#5806=ORIENTED_EDGE('',*,*,#3978,.T.);
#5807=ORIENTED_EDGE('',*,*,#3979,.T.);
#5808=ORIENTED_EDGE('',*,*,#3980,.T.);
#5809=ORIENTED_EDGE('',*,*,#3981,.T.);
#5810=ORIENTED_EDGE('',*,*,#3975,.F.);
#5811=ORIENTED_EDGE('',*,*,#3982,.T.);
#5812=ORIENTED_EDGE('',*,*,#3983,.T.);
#5813=ORIENTED_EDGE('',*,*,#3984,.T.);
#5814=ORIENTED_EDGE('',*,*,#3985,.T.);
#5815=ORIENTED_EDGE('',*,*,#3979,.F.);
#5816=ORIENTED_EDGE('',*,*,#3986,.T.);
#5817=ORIENTED_EDGE('',*,*,#3987,.T.);
#5818=ORIENTED_EDGE('',*,*,#3988,.T.);
#5819=ORIENTED_EDGE('',*,*,#3989,.T.);
#5820=ORIENTED_EDGE('',*,*,#3990,.T.);
#5821=ORIENTED_EDGE('',*,*,#3984,.F.);
#5822=ORIENTED_EDGE('',*,*,#3991,.T.);
#5823=ORIENTED_EDGE('',*,*,#3992,.T.);
#5824=ORIENTED_EDGE('',*,*,#3993,.F.);
#5825=ORIENTED_EDGE('',*,*,#3994,.T.);
#5826=ORIENTED_EDGE('',*,*,#3995,.F.);
#5827=ORIENTED_EDGE('',*,*,#3996,.T.);
#5828=ORIENTED_EDGE('',*,*,#3997,.T.);
#5829=ORIENTED_EDGE('',*,*,#3993,.T.);
#5830=ORIENTED_EDGE('',*,*,#3998,.T.);
#5831=ORIENTED_EDGE('',*,*,#3988,.F.);
#5832=ORIENTED_EDGE('',*,*,#3999,.T.);
#5833=ORIENTED_EDGE('',*,*,#4000,.T.);
#5834=ORIENTED_EDGE('',*,*,#3948,.T.);
#5835=ORIENTED_EDGE('',*,*,#4001,.T.);
#5836=ORIENTED_EDGE('',*,*,#4002,.T.);
#5837=ORIENTED_EDGE('',*,*,#3943,.F.);
#5838=ORIENTED_EDGE('',*,*,#4003,.F.);
#5839=ORIENTED_EDGE('',*,*,#4004,.F.);
#5840=ORIENTED_EDGE('',*,*,#4005,.F.);
#5841=ORIENTED_EDGE('',*,*,#4006,.T.);
#5842=ORIENTED_EDGE('',*,*,#4007,.F.);
#5843=ORIENTED_EDGE('',*,*,#4006,.F.);
#5844=ORIENTED_EDGE('',*,*,#4008,.F.);
#5845=ORIENTED_EDGE('',*,*,#4009,.T.);
#5846=ORIENTED_EDGE('',*,*,#4010,.F.);
#5847=ORIENTED_EDGE('',*,*,#4009,.F.);
#5848=ORIENTED_EDGE('',*,*,#4011,.F.);
#5849=ORIENTED_EDGE('',*,*,#3905,.F.);
#5850=ORIENTED_EDGE('',*,*,#3910,.F.);
#5851=ORIENTED_EDGE('',*,*,#3909,.F.);
#5852=ORIENTED_EDGE('',*,*,#3915,.F.);
#5853=ORIENTED_EDGE('',*,*,#3914,.F.);
#5854=ORIENTED_EDGE('',*,*,#3920,.F.);
#5855=ORIENTED_EDGE('',*,*,#3919,.F.);
#5856=ORIENTED_EDGE('',*,*,#3925,.F.);
#5857=ORIENTED_EDGE('',*,*,#3924,.F.);
#5858=ORIENTED_EDGE('',*,*,#3930,.F.);
#5859=ORIENTED_EDGE('',*,*,#3929,.F.);
#5860=ORIENTED_EDGE('',*,*,#3935,.F.);
#5861=ORIENTED_EDGE('',*,*,#3934,.F.);
#5862=ORIENTED_EDGE('',*,*,#3940,.F.);
#5863=ORIENTED_EDGE('',*,*,#3939,.F.);
#5864=ORIENTED_EDGE('',*,*,#3945,.F.);
#5865=ORIENTED_EDGE('',*,*,#3944,.F.);
#5866=ORIENTED_EDGE('',*,*,#4002,.F.);
#5867=ORIENTED_EDGE('',*,*,#4001,.F.);
#5868=ORIENTED_EDGE('',*,*,#3953,.F.);
#5869=ORIENTED_EDGE('',*,*,#3952,.F.);
#5870=ORIENTED_EDGE('',*,*,#4012,.F.);
#5871=ORIENTED_EDGE('',*,*,#3994,.F.);
#5872=ORIENTED_EDGE('',*,*,#4000,.F.);
#5873=ORIENTED_EDGE('',*,*,#3999,.F.);
#5874=ORIENTED_EDGE('',*,*,#3992,.F.);
#5875=ORIENTED_EDGE('',*,*,#3991,.F.);
#5876=ORIENTED_EDGE('',*,*,#3987,.F.);
#5877=ORIENTED_EDGE('',*,*,#3986,.F.);
#5878=ORIENTED_EDGE('',*,*,#3983,.F.);
#5879=ORIENTED_EDGE('',*,*,#3982,.F.);
#5880=ORIENTED_EDGE('',*,*,#3978,.F.);
#5881=ORIENTED_EDGE('',*,*,#3977,.F.);
#5882=ORIENTED_EDGE('',*,*,#3974,.F.);
#5883=ORIENTED_EDGE('',*,*,#3970,.F.);
#5884=ORIENTED_EDGE('',*,*,#3969,.F.);
#5885=ORIENTED_EDGE('',*,*,#3965,.F.);
#5886=ORIENTED_EDGE('',*,*,#3964,.F.);
#5887=ORIENTED_EDGE('',*,*,#3960,.F.);
#5888=ORIENTED_EDGE('',*,*,#3957,.F.);
#5889=ORIENTED_EDGE('',*,*,#4013,.F.);
#5890=ORIENTED_EDGE('',*,*,#4014,.F.);
#5891=ORIENTED_EDGE('',*,*,#3955,.F.);
#5892=ORIENTED_EDGE('',*,*,#3959,.F.);
#5893=ORIENTED_EDGE('',*,*,#3963,.F.);
#5894=ORIENTED_EDGE('',*,*,#3962,.F.);
#5895=ORIENTED_EDGE('',*,*,#3968,.F.);
#5896=ORIENTED_EDGE('',*,*,#3967,.F.);
#5897=ORIENTED_EDGE('',*,*,#3973,.F.);
#5898=ORIENTED_EDGE('',*,*,#3972,.F.);
#5899=ORIENTED_EDGE('',*,*,#3976,.F.);
#5900=ORIENTED_EDGE('',*,*,#3981,.F.);
#5901=ORIENTED_EDGE('',*,*,#3980,.F.);
#5902=ORIENTED_EDGE('',*,*,#3985,.F.);
#5903=ORIENTED_EDGE('',*,*,#3990,.F.);
#5904=ORIENTED_EDGE('',*,*,#3989,.F.);
#5905=ORIENTED_EDGE('',*,*,#3998,.F.);
#5906=ORIENTED_EDGE('',*,*,#3997,.F.);
#5907=ORIENTED_EDGE('',*,*,#3996,.F.);
#5908=ORIENTED_EDGE('',*,*,#4015,.F.);
#5909=ORIENTED_EDGE('',*,*,#3950,.T.);
#5910=ORIENTED_EDGE('',*,*,#3949,.T.);
#5911=ORIENTED_EDGE('',*,*,#4004,.T.);
#5912=ORIENTED_EDGE('',*,*,#4003,.T.);
#5913=ORIENTED_EDGE('',*,*,#3947,.T.);
#5914=ORIENTED_EDGE('',*,*,#3946,.T.);
#5915=ORIENTED_EDGE('',*,*,#3942,.T.);
#5916=ORIENTED_EDGE('',*,*,#3941,.T.);
#5917=ORIENTED_EDGE('',*,*,#3937,.T.);
#5918=ORIENTED_EDGE('',*,*,#3936,.T.);
#5919=ORIENTED_EDGE('',*,*,#3932,.T.);
#5920=ORIENTED_EDGE('',*,*,#3931,.T.);
#5921=ORIENTED_EDGE('',*,*,#3927,.T.);
#5922=ORIENTED_EDGE('',*,*,#3926,.T.);
#5923=ORIENTED_EDGE('',*,*,#3922,.T.);
#5924=ORIENTED_EDGE('',*,*,#3921,.T.);
#5925=ORIENTED_EDGE('',*,*,#3917,.T.);
#5926=ORIENTED_EDGE('',*,*,#3916,.T.);
#5927=ORIENTED_EDGE('',*,*,#3912,.T.);
#5928=ORIENTED_EDGE('',*,*,#3911,.T.);
#5929=ORIENTED_EDGE('',*,*,#3907,.T.);
#5930=ORIENTED_EDGE('',*,*,#4016,.T.);
#5931=ORIENTED_EDGE('',*,*,#4017,.T.);
#5932=ORIENTED_EDGE('',*,*,#4018,.T.);
#5933=ORIENTED_EDGE('',*,*,#4019,.T.);
#5934=ORIENTED_EDGE('',*,*,#4005,.T.);
#5935=ORIENTED_EDGE('',*,*,#4008,.T.);
#5936=ORIENTED_EDGE('',*,*,#4020,.T.);
#5937=ORIENTED_EDGE('',*,*,#4021,.T.);
#5938=ORIENTED_EDGE('',*,*,#4012,.T.);
#5939=ORIENTED_EDGE('',*,*,#3951,.T.);
#5940=ORIENTED_EDGE('',*,*,#4015,.T.);
#5941=ORIENTED_EDGE('',*,*,#3995,.T.);
#5942=ORIENTED_EDGE('',*,*,#4021,.F.);
#5943=ORIENTED_EDGE('',*,*,#4022,.T.);
#5944=ORIENTED_EDGE('',*,*,#4023,.F.);
#5945=ORIENTED_EDGE('',*,*,#4022,.F.);
#5946=ORIENTED_EDGE('',*,*,#4020,.F.);
#5947=ORIENTED_EDGE('',*,*,#4024,.T.);
#5948=ORIENTED_EDGE('',*,*,#4025,.F.);
#5949=ORIENTED_EDGE('',*,*,#4024,.F.);
#5950=ORIENTED_EDGE('',*,*,#4026,.T.);
#5951=ORIENTED_EDGE('',*,*,#4027,.T.);
#5952=ORIENTED_EDGE('',*,*,#4019,.F.);
#5953=ORIENTED_EDGE('',*,*,#4028,.F.);
#5954=ORIENTED_EDGE('',*,*,#4029,.T.);
#5955=ORIENTED_EDGE('',*,*,#4028,.T.);
#5956=ORIENTED_EDGE('',*,*,#4018,.F.);
#5957=ORIENTED_EDGE('',*,*,#4030,.F.);
#5958=ORIENTED_EDGE('',*,*,#4031,.T.);
#5959=ORIENTED_EDGE('',*,*,#4030,.T.);
#5960=ORIENTED_EDGE('',*,*,#4017,.F.);
#5961=ORIENTED_EDGE('',*,*,#4032,.F.);
#5962=ORIENTED_EDGE('',*,*,#4033,.T.);
#5963=ORIENTED_EDGE('',*,*,#4032,.T.);
#5964=ORIENTED_EDGE('',*,*,#4016,.F.);
#5965=ORIENTED_EDGE('',*,*,#4027,.F.);
#5966=ORIENTED_EDGE('',*,*,#4033,.F.);
#5967=ORIENTED_EDGE('',*,*,#4026,.F.);
#5968=ORIENTED_EDGE('',*,*,#4029,.F.);
#5969=ORIENTED_EDGE('',*,*,#4031,.F.);
#5970=ORIENTED_EDGE('',*,*,#4007,.T.);
#5971=ORIENTED_EDGE('',*,*,#4010,.T.);
#5972=ORIENTED_EDGE('',*,*,#4011,.T.);
#5973=ORIENTED_EDGE('',*,*,#4013,.T.);
#5974=ORIENTED_EDGE('',*,*,#3956,.T.);
#5975=ORIENTED_EDGE('',*,*,#4014,.T.);
#5976=ORIENTED_EDGE('',*,*,#3906,.T.);
#5977=ORIENTED_EDGE('',*,*,#4023,.T.);
#5978=ORIENTED_EDGE('',*,*,#4025,.T.);
#6838=CYLINDRICAL_SURFACE('',#7539,8.12525);
#6839=CYLINDRICAL_SURFACE('',#7541,8.12525);
#6840=CYLINDRICAL_SURFACE('',#7542,8.12525);
#6841=CYLINDRICAL_SURFACE('',#7543,8.12525);
#6842=CYLINDRICAL_SURFACE('',#7544,8.12525);
#6843=CYLINDRICAL_SURFACE('',#7545,8.12525);
#6844=CYLINDRICAL_SURFACE('',#7546,8.12525);
#6845=CYLINDRICAL_SURFACE('',#7547,8.12525);
#6846=CYLINDRICAL_SURFACE('',#7548,8.12525);
#6847=CYLINDRICAL_SURFACE('',#7549,8.12525);
#6848=CYLINDRICAL_SURFACE('',#7551,7.01125);
#6849=CYLINDRICAL_SURFACE('',#7553,7.01125);
#6850=CYLINDRICAL_SURFACE('',#7554,7.01125);
#6851=CYLINDRICAL_SURFACE('',#7555,7.01125);
#6852=CYLINDRICAL_SURFACE('',#7556,7.01125);
#6853=CYLINDRICAL_SURFACE('',#7557,7.01125);
#6854=CYLINDRICAL_SURFACE('',#7558,7.01125);
#6855=CYLINDRICAL_SURFACE('',#7559,7.01125);
#6856=CYLINDRICAL_SURFACE('',#7560,7.01125);
#6857=CYLINDRICAL_SURFACE('',#7561,7.01125);
#6858=CYLINDRICAL_SURFACE('',#7563,7.01125);
#6859=CYLINDRICAL_SURFACE('',#7564,8.12525);
#6860=CYLINDRICAL_SURFACE('',#7565,3.5);
#6861=CYLINDRICAL_SURFACE('',#7568,3.5);
#6862=CYLINDRICAL_SURFACE('',#7574,6.);
#6863=CYLINDRICAL_SURFACE('',#7576,6.);
#7066=ADVANCED_FACE('',(#1201),#6838,.F.);
#7067=ADVANCED_FACE('',(#1202),#6839,.F.);
#7068=ADVANCED_FACE('',(#1203),#6840,.F.);
#7069=ADVANCED_FACE('',(#1204),#6841,.F.);
#7070=ADVANCED_FACE('',(#1205),#6842,.F.);
#7071=ADVANCED_FACE('',(#1206),#6843,.F.);
#7072=ADVANCED_FACE('',(#1207),#6844,.F.);
#7073=ADVANCED_FACE('',(#1208),#6845,.F.);
#7074=ADVANCED_FACE('',(#1209),#6846,.F.);
#7075=ADVANCED_FACE('',(#1210),#6847,.F.);
#7076=ADVANCED_FACE('',(#1211),#6848,.F.);
#7077=ADVANCED_FACE('',(#1212),#6849,.F.);
#7078=ADVANCED_FACE('',(#1213),#6850,.F.);
#7079=ADVANCED_FACE('',(#1214),#6851,.F.);
#7080=ADVANCED_FACE('',(#1215),#6852,.F.);
#7081=ADVANCED_FACE('',(#1216),#6853,.F.);
#7082=ADVANCED_FACE('',(#1217),#6854,.F.);
#7083=ADVANCED_FACE('',(#1218),#6855,.F.);
#7084=ADVANCED_FACE('',(#1219),#6856,.F.);
#7085=ADVANCED_FACE('',(#1220),#6857,.F.);
#7086=ADVANCED_FACE('',(#1221),#6858,.F.);
#7087=ADVANCED_FACE('',(#1222),#6859,.F.);
#7088=ADVANCED_FACE('',(#1223),#6860,.F.);
#7089=ADVANCED_FACE('',(#1224),#6861,.F.);
#7090=ADVANCED_FACE('',(#1225),#97,.F.);
#7091=ADVANCED_FACE('',(#1226),#98,.F.);
#7092=ADVANCED_FACE('',(#1227,#973,#974,#975,#976,#977),#1030,.T.);
#7093=ADVANCED_FACE('',(#1228),#6862,.F.);
#7094=ADVANCED_FACE('',(#1229),#6863,.F.);
#7095=ADVANCED_FACE('',(#1230),#1031,.T.);
#7096=ADVANCED_FACE('',(#1231),#1032,.T.);
#7097=ADVANCED_FACE('',(#1232),#1033,.T.);
#7098=ADVANCED_FACE('',(#1233),#1034,.T.);
#7099=ADVANCED_FACE('',(#1234,#978,#979,#980,#981,#982),#1035,.F.);
#7207=CLOSED_SHELL('',(#7066,#7067,#7068,#7069,#7070,#7071,#7072,#7073,
#7074,#7075,#7076,#7077,#7078,#7079,#7080,#7081,#7082,#7083,#7084,#7085,
#7086,#7087,#7088,#7089,#7090,#7091,#7092,#7093,#7094,#7095,#7096,#7097,
#7098,#7099));
#7538=AXIS2_PLACEMENT_3D('',#71897,#8272,#8273);
#7539=AXIS2_PLACEMENT_3D('',#71898,#8274,#8275);
#7540=AXIS2_PLACEMENT_3D('',#71912,#8277,#8278);
#7541=AXIS2_PLACEMENT_3D('',#71922,#8279,#8280);
#7542=AXIS2_PLACEMENT_3D('',#72292,#8282,#8283);
#7543=AXIS2_PLACEMENT_3D('',#72510,#8285,#8286);
#7544=AXIS2_PLACEMENT_3D('',#72878,#8288,#8289);
#7545=AXIS2_PLACEMENT_3D('',#73419,#8291,#8292);
#7546=AXIS2_PLACEMENT_3D('',#73960,#8294,#8295);
#7547=AXIS2_PLACEMENT_3D('',#74342,#8297,#8298);
#7548=AXIS2_PLACEMENT_3D('',#74794,#8300,#8301);
#7549=AXIS2_PLACEMENT_3D('',#75178,#8303,#8304);
#7550=AXIS2_PLACEMENT_3D('',#75200,#8306,#8307);
#7551=AXIS2_PLACEMENT_3D('',#75218,#8308,#8309);
#7552=AXIS2_PLACEMENT_3D('',#75232,#8311,#8312);
#7553=AXIS2_PLACEMENT_3D('',#75277,#8313,#8314);
#7554=AXIS2_PLACEMENT_3D('',#75529,#8316,#8317);
#7555=AXIS2_PLACEMENT_3D('',#75824,#8319,#8320);
#7556=AXIS2_PLACEMENT_3D('',#76213,#8322,#8323);
#7557=AXIS2_PLACEMENT_3D('',#76471,#8325,#8326);
#7558=AXIS2_PLACEMENT_3D('',#76618,#8328,#8329);
#7559=AXIS2_PLACEMENT_3D('',#77012,#8331,#8332);
#7560=AXIS2_PLACEMENT_3D('',#77169,#8334,#8335);
#7561=AXIS2_PLACEMENT_3D('',#77551,#8337,#8338);
#7562=AXIS2_PLACEMENT_3D('',#77635,#8340,#8341);
#7563=AXIS2_PLACEMENT_3D('',#77882,#8342,#8343);
#7564=AXIS2_PLACEMENT_3D('',#78143,#8344,#8345);
#7565=AXIS2_PLACEMENT_3D('',#78272,#8346,#8347);
#7566=AXIS2_PLACEMENT_3D('',#78274,#8348,#8349);
#7567=AXIS2_PLACEMENT_3D('',#78277,#8351,#8352);
#7568=AXIS2_PLACEMENT_3D('',#78278,#8353,#8354);
#7569=AXIS2_PLACEMENT_3D('',#78280,#8355,#8356);
#7570=AXIS2_PLACEMENT_3D('',#78283,#8358,#8359);
#7571=AXIS2_PLACEMENT_3D('',#79804,#8360,#8361);
#7572=AXIS2_PLACEMENT_3D('',#79814,#8366,#8367);
#7573=AXIS2_PLACEMENT_3D('',#79816,#8368,#8369);
#7574=AXIS2_PLACEMENT_3D('',#79817,#8370,#8371);
#7575=AXIS2_PLACEMENT_3D('',#79820,#8373,#8374);
#7576=AXIS2_PLACEMENT_3D('',#79821,#8375,#8376);
#7577=AXIS2_PLACEMENT_3D('',#79824,#8378,#8379);
#7578=AXIS2_PLACEMENT_3D('',#79825,#8380,#8381);
#7579=AXIS2_PLACEMENT_3D('',#79831,#8385,#8386);
#7580=AXIS2_PLACEMENT_3D('',#79835,#8389,#8390);
#7581=AXIS2_PLACEMENT_3D('',#79839,#8393,#8394);
#7582=AXIS2_PLACEMENT_3D('',#79841,#8396,#8397);
#8272=DIRECTION('axis',(0.,0.,1.));
#8273=DIRECTION('refdir',(1.,0.,0.));
#8274=DIRECTION('center_axis',(0.,0.,-1.));
#8275=DIRECTION('ref_axis',(-0.608813211676711,-0.793313603367475,0.));
#8276=DIRECTION('',(0.,0.,-1.));
#8277=DIRECTION('center_axis',(0.,0.,1.));
#8278=DIRECTION('ref_axis',(1.,-3.58774509990574E-14,0.));
#8279=DIRECTION('center_axis',(0.,0.,-1.));
#8280=DIRECTION('ref_axis',(-0.608813211676711,-0.793313603367475,0.));
#8281=DIRECTION('',(0.,0.,-1.));
#8282=DIRECTION('center_axis',(0.,0.,-1.));
#8283=DIRECTION('ref_axis',(-0.608813211676711,-0.793313603367475,0.));
#8284=DIRECTION('',(0.,0.,-1.));
#8285=DIRECTION('center_axis',(0.,0.,-1.));
#8286=DIRECTION('ref_axis',(-0.608813211676711,-0.793313603367475,0.));
#8287=DIRECTION('',(0.,0.,-1.));
#8288=DIRECTION('center_axis',(0.,0.,-1.));
#8289=DIRECTION('ref_axis',(-0.608813211676711,-0.793313603367475,0.));
#8290=DIRECTION('',(0.,0.,-1.));
#8291=DIRECTION('center_axis',(0.,0.,-1.));
#8292=DIRECTION('ref_axis',(-0.608813211676711,-0.793313603367475,0.));
#8293=DIRECTION('',(0.,0.,-1.));
#8294=DIRECTION('center_axis',(0.,0.,-1.));
#8295=DIRECTION('ref_axis',(-0.608813211676711,-0.793313603367475,0.));
#8296=DIRECTION('',(0.,0.,-1.));
#8297=DIRECTION('center_axis',(0.,0.,-1.));
#8298=DIRECTION('ref_axis',(-0.608813211676711,-0.793313603367475,0.));
#8299=DIRECTION('',(0.,0.,-1.));
#8300=DIRECTION('center_axis',(0.,0.,-1.));
#8301=DIRECTION('ref_axis',(-0.608813211676711,-0.793313603367475,0.));
#8302=DIRECTION('',(0.,0.,-1.));
#8303=DIRECTION('center_axis',(0.,0.,-1.));
#8304=DIRECTION('ref_axis',(-0.608813211676711,-0.793313603367475,0.));
#8305=DIRECTION('',(0.,0.,-1.));
#8306=DIRECTION('center_axis',(0.,0.,-1.));
#8307=DIRECTION('ref_axis',(1.,-3.58774509990574E-14,0.));
#8308=DIRECTION('center_axis',(0.,0.,-1.));
#8309=DIRECTION('ref_axis',(0.937388910103482,-0.348284411386738,0.));
#8310=DIRECTION('',(0.,0.,-1.));
#8311=DIRECTION('center_axis',(0.,0.,-1.));
#8312=DIRECTION('ref_axis',(1.,0.,0.));
#8313=DIRECTION('center_axis',(0.,0.,-1.));
#8314=DIRECTION('ref_axis',(0.937388910103482,-0.348284411386738,0.));
#8315=DIRECTION('',(0.,0.,-1.));
#8316=DIRECTION('center_axis',(0.,0.,-1.));
#8317=DIRECTION('ref_axis',(0.937388910103482,-0.348284411386738,0.));
#8318=DIRECTION('',(0.,0.,-1.));
#8319=DIRECTION('center_axis',(0.,0.,-1.));
#8320=DIRECTION('ref_axis',(0.937388910103482,-0.348284411386738,0.));
#8321=DIRECTION('',(0.,0.,-1.));
#8322=DIRECTION('center_axis',(0.,0.,-1.));
#8323=DIRECTION('ref_axis',(0.937388910103482,-0.348284411386738,0.));
#8324=DIRECTION('',(0.,0.,-1.));
#8325=DIRECTION('center_axis',(0.,0.,-1.));
#8326=DIRECTION('ref_axis',(0.937388910103482,-0.348284411386738,0.));
#8327=DIRECTION('',(0.,0.,-1.));
#8328=DIRECTION('center_axis',(0.,0.,-1.));
#8329=DIRECTION('ref_axis',(0.937388910103482,-0.348284411386738,0.));
#8330=DIRECTION('',(0.,0.,-1.));
#8331=DIRECTION('center_axis',(0.,0.,-1.));
#8332=DIRECTION('ref_axis',(0.937388910103482,-0.348284411386738,0.));
#8333=DIRECTION('',(0.,0.,-1.));
#8334=DIRECTION('center_axis',(0.,0.,-1.));
#8335=DIRECTION('ref_axis',(0.937388910103482,-0.348284411386738,0.));
#8336=DIRECTION('',(0.,0.,-1.));
#8337=DIRECTION('center_axis',(0.,0.,-1.));
#8338=DIRECTION('ref_axis',(0.937388910103482,-0.348284411386738,0.));
#8339=DIRECTION('',(0.,0.,-1.));
#8340=DIRECTION('center_axis',(0.,0.,-1.));
#8341=DIRECTION('ref_axis',(1.,0.,0.));
#8342=DIRECTION('center_axis',(0.,0.,-1.));
#8343=DIRECTION('ref_axis',(0.937388910103482,-0.348284411386738,0.));
#8344=DIRECTION('center_axis',(0.,0.,-1.));
#8345=DIRECTION('ref_axis',(-0.608813211676711,-0.793313603367475,0.));
#8346=DIRECTION('center_axis',(0.,0.,-1.));
#8347=DIRECTION('ref_axis',(1.,0.,0.));
#8348=DIRECTION('center_axis',(0.,0.,-1.));
#8349=DIRECTION('ref_axis',(1.,0.,0.));
#8350=DIRECTION('',(0.,0.,-1.));
#8351=DIRECTION('center_axis',(0.,0.,1.));
#8352=DIRECTION('ref_axis',(1.,0.,0.));
#8353=DIRECTION('center_axis',(0.,0.,-1.));
#8354=DIRECTION('ref_axis',(1.,0.,0.));
#8355=DIRECTION('center_axis',(0.,0.,-1.));
#8356=DIRECTION('ref_axis',(1.,0.,0.));
#8357=DIRECTION('',(0.,0.,-1.));
#8358=DIRECTION('center_axis',(0.,0.,1.));
#8359=DIRECTION('ref_axis',(1.,0.,0.));
#8360=DIRECTION('center_axis',(0.,0.,1.));
#8361=DIRECTION('ref_axis',(1.,0.,0.));
#8362=DIRECTION('',(0.,-1.,0.));
#8363=DIRECTION('',(1.,0.,0.));
#8364=DIRECTION('',(0.,1.,0.));
#8365=DIRECTION('',(1.,0.,0.));
#8366=DIRECTION('center_axis',(0.,0.,-1.));
#8367=DIRECTION('ref_axis',(1.,0.,0.));
#8368=DIRECTION('center_axis',(0.,0.,-1.));
#8369=DIRECTION('ref_axis',(1.,0.,0.));
#8370=DIRECTION('center_axis',(0.,0.,-1.));
#8371=DIRECTION('ref_axis',(1.,0.,0.));
#8372=DIRECTION('',(0.,0.,-1.));
#8373=DIRECTION('center_axis',(0.,0.,1.));
#8374=DIRECTION('ref_axis',(1.,0.,0.));
#8375=DIRECTION('center_axis',(0.,0.,-1.));
#8376=DIRECTION('ref_axis',(1.,0.,0.));
#8377=DIRECTION('',(0.,0.,-1.));
#8378=DIRECTION('center_axis',(0.,0.,1.));
#8379=DIRECTION('ref_axis',(1.,0.,0.));
#8380=DIRECTION('center_axis',(0.,1.,0.));
#8381=DIRECTION('ref_axis',(-1.,0.,0.));
#8382=DIRECTION('',(1.,0.,0.));
#8383=DIRECTION('',(0.,0.,1.));
#8384=DIRECTION('',(0.,0.,-1.));
#8385=DIRECTION('center_axis',(1.,0.,0.));
#8386=DIRECTION('ref_axis',(0.,1.,0.));
#8387=DIRECTION('',(0.,1.,0.));
#8388=DIRECTION('',(0.,0.,1.));
#8389=DIRECTION('center_axis',(0.,-1.,0.));
#8390=DIRECTION('ref_axis',(1.,0.,0.));
#8391=DIRECTION('',(1.,0.,0.));
#8392=DIRECTION('',(0.,0.,1.));
#8393=DIRECTION('center_axis',(-1.,0.,0.));
#8394=DIRECTION('ref_axis',(0.,-1.,0.));
#8395=DIRECTION('',(0.,-1.,0.));
#8396=DIRECTION('center_axis',(0.,0.,1.));
#8397=DIRECTION('ref_axis',(1.,0.,0.));
#71897=CARTESIAN_POINT('',(0.,0.,0.));
#71898=CARTESIAN_POINT('Origin',(0.,0.,24.4167025567876));
#71899=CARTESIAN_POINT('',(4.94636091871675,6.44535235552233,0.874940417221147));
#71900=CARTESIAN_POINT('',(4.94635496516529,6.4453438615057,0.708350185246763));
#71901=CARTESIAN_POINT('',(4.9467595481762,6.44587135576158,24.4167025567876));
#71902=CARTESIAN_POINT('',(2.10208451021607,-7.84862588447237,0.));
#71903=CARTESIAN_POINT('Ctrl Pts',(4.94635496517363,6.44534386149931,0.708350185246352));
#71904=CARTESIAN_POINT('Ctrl Pts',(5.44049095014118,6.06630505566983,0.683958258880921));
#71905=CARTESIAN_POINT('Ctrl Pts',(6.87015483931645,4.68667886721249,0.606635132002986));
#71906=CARTESIAN_POINT('Ctrl Pts',(8.32157346971745,1.57860155059824,0.476380804612548));
#71907=CARTESIAN_POINT('Ctrl Pts',(8.06280828226814,-2.59475929044894,0.317587203075035));
#71908=CARTESIAN_POINT('Ctrl Pts',(5.8384210982867,-6.13665782895719,0.158793601537515));
#71909=CARTESIAN_POINT('Ctrl Pts',(3.40721893572613,-7.4990738864542,0.0529312005125064));
#71910=CARTESIAN_POINT('Ctrl Pts',(2.10208451021607,-7.84862588447237,0.));
#71911=CARTESIAN_POINT('',(-2.10231583414457,-7.84925104679543,-1.60949812505473E-15));
#71912=CARTESIAN_POINT('Origin',(0.,0.,0.));
#71913=CARTESIAN_POINT('Ctrl Pts',(4.94636091871776,6.44535235552155,0.874940417221097));
#71914=CARTESIAN_POINT('Ctrl Pts',(5.54686650886728,5.98419136571353,0.845285016134203));
#71915=CARTESIAN_POINT('Ctrl Pts',(7.04180178671693,4.46845944575802,0.762698414534804));
#71916=CARTESIAN_POINT('Ctrl Pts',(8.38967733351479,1.16400612135573,0.6271806124229));
#71917=CARTESIAN_POINT('Ctrl Pts',(7.92408883944575,-2.99170878695321,0.46838701088538));
#71918=CARTESIAN_POINT('Ctrl Pts',(5.52703242316562,-6.41823535228475,0.309593409347865));
#71919=CARTESIAN_POINT('Ctrl Pts',(1.8455873829112,-8.24902208290505,0.153464405719403));
#71920=CARTESIAN_POINT('Ctrl Pts',(-0.863038767841767,-8.18056566201579,
0.0502666026034473));
#71921=CARTESIAN_POINT('Ctrl Pts',(-2.10231583414457,-7.84925104679543,
-1.60949812505473E-15));
#71922=CARTESIAN_POINT('Origin',(0.,0.,24.4167025567876));
#71923=CARTESIAN_POINT('',(4.9467595481762,6.44587135576158,2.87494842260025));
#71924=CARTESIAN_POINT('',(4.94675954817618,6.44587135576159,2.70835108074798));
#71925=CARTESIAN_POINT('',(4.9467595481762,6.44587135576158,24.4167025567876));
#71926=CARTESIAN_POINT('',(-8.12526511089558,-0.000106822124032805,1.4167025564899));
#71927=CARTESIAN_POINT('Ctrl Pts',(4.94675954817618,6.44587135576159,2.70835108074799));
#71928=CARTESIAN_POINT('Ctrl Pts',(5.00654996272257,6.39998635624443,2.70539779587792));
#71929=CARTESIAN_POINT('Ctrl Pts',(5.0656987513671,6.35327181669309,2.70244451100785));
#71930=CARTESIAN_POINT('Ctrl Pts',(5.12418284497226,6.30574640576292,2.69949122613778));
#71931=CARTESIAN_POINT('Ctrl Pts',(5.28700683250325,6.17343219108189,2.69126906538914));
#71932=CARTESIAN_POINT('Ctrl Pts',(5.44473011680673,6.03478622619136,2.68304690464051));
#71933=CARTESIAN_POINT('Ctrl Pts',(5.5968671918238,5.89022624349748,2.67482474389187));
#71934=CARTESIAN_POINT('Ctrl Pts',(5.74897622359167,5.74569290737622,2.66660409872451));
#71935=CARTESIAN_POINT('Ctrl Pts',(5.89550088736123,5.59524793238774,2.65838345355716));
#71936=CARTESIAN_POINT('Ctrl Pts',(6.03599120669964,5.43934717729477,2.6501628083898));
#71937=CARTESIAN_POINT('Ctrl Pts',(6.17646574291822,5.28346393657796,2.64194308675531));
#71938=CARTESIAN_POINT('Ctrl Pts',(6.31090709061718,5.12212635857307,2.63372336512082));
#71939=CARTESIAN_POINT('Ctrl Pts',(6.43890381653687,4.95582538068956,2.62550364348633));
#71940=CARTESIAN_POINT('Ctrl Pts',(6.56691079828585,4.78951107782118,2.61728326324077));
#71941=CARTESIAN_POINT('Ctrl Pts',(6.68847194429077,4.61823281266861,2.60906288299519));
#71942=CARTESIAN_POINT('Ctrl Pts',(6.80321698323602,4.44251350493264,2.60084250274963));
#71943=CARTESIAN_POINT('Ctrl Pts',(6.91796159749113,4.26679484756256,2.59262215292903));
#71944=CARTESIAN_POINT('Ctrl Pts',(7.02588999601499,4.0866354290706,2.58440180310845));
#71945=CARTESIAN_POINT('Ctrl Pts',(7.12667572325493,3.90258641135193,2.57618145328786));
#71946=CARTESIAN_POINT('Ctrl Pts',(7.22748299970096,3.71849804172979,2.56795934585716));
#71947=CARTESIAN_POINT('Ctrl Pts',(7.32114441204801,3.53051867034308,2.55973723842646));
#71948=CARTESIAN_POINT('Ctrl Pts',(7.4073793590196,3.33922425034175,2.55151513099576));
#71949=CARTESIAN_POINT('Ctrl Pts',(7.44519801229645,3.25533137862455,2.5479092955306));
#71950=CARTESIAN_POINT('Ctrl Pts',(7.48158894702567,3.17080121861856,2.54430346006544));
#71951=CARTESIAN_POINT('Ctrl Pts',(7.5165313868341,3.08568363142396,2.54069762460027));
#71952=CARTESIAN_POINT('Ctrl Pts',(7.59620841783576,2.89159539171117,2.53247546651058));
#71953=CARTESIAN_POINT('Ctrl Pts',(7.66837709955814,2.69438740193867,2.52425330842089));
#71954=CARTESIAN_POINT('Ctrl Pts',(7.73281095174109,2.49465876366551,2.51603115033119));
#71955=CARTESIAN_POINT('Ctrl Pts',(7.79723292682117,2.29496694140597,2.50781050783329));
#71956=CARTESIAN_POINT('Ctrl Pts',(7.8539228274159,2.09275567873303,2.49958986533539));
#71957=CARTESIAN_POINT('Ctrl Pts',(7.90270361351394,1.88864055856421,2.49136922283748));
#71958=CARTESIAN_POINT('Ctrl Pts',(7.9514789194125,1.68454836938245,2.48314950387452));
#71959=CARTESIAN_POINT('Ctrl Pts',(7.99234681613915,1.47855303665947,2.47492978491157));
#71960=CARTESIAN_POINT('Ctrl Pts',(8.02518089209509,1.27128250662546,2.46671006594861));
#71961=CARTESIAN_POINT('Ctrl Pts',(8.05801759897362,1.06399536845787,2.45848968835758));
#71962=CARTESIAN_POINT('Ctrl Pts',(8.08281914996309,0.855433119907242,2.45026931076654));
#71963=CARTESIAN_POINT('Ctrl Pts',(8.09951058010313,0.646232098628225,2.44204893317551));
#71964=CARTESIAN_POINT('Ctrl Pts',(8.11620194849499,0.437031851266314,2.4338285859949));
#71965=CARTESIAN_POINT('Ctrl Pts',(8.12478323524068,0.227193130324511,2.42560823881427));
#71966=CARTESIAN_POINT('Ctrl Pts',(8.12523146303619,0.0173561109345648,
2.41738789163366));
#71967=CARTESIAN_POINT('Ctrl Pts',(8.12567978667038,-0.192525775157294,
2.40916578680386));
#71968=CARTESIAN_POINT('Ctrl Pts',(8.11799157656876,-0.402405663767066,
2.40094368197406));
#71969=CARTESIAN_POINT('Ctrl Pts',(8.10219598212575,-0.611643547930737,
2.39272157714425));
#71970=CARTESIAN_POINT('Ctrl Pts',(8.09526873333835,-0.703406025410291,
2.38911572578376));
#71971=CARTESIAN_POINT('Ctrl Pts',(8.08678285649728,-0.795045059485583,
2.38550987442326));
#71972=CARTESIAN_POINT('Ctrl Pts',(8.0767439624085,-0.886506925070441,2.38190402306276));
#71973=CARTESIAN_POINT('Ctrl Pts',(8.05385299354372,-1.09506084534311,2.37368185929709));
#71974=CARTESIAN_POINT('Ctrl Pts',(8.0228761563586,-1.30276208569347,2.36545969553142));
#71975=CARTESIAN_POINT('Ctrl Pts',(7.98390120047228,-1.50897620378761,2.35723753176575));
#71976=CARTESIAN_POINT('Ctrl Pts',(7.94493342875514,-1.71515231088016,2.34901688357372));
#71977=CARTESIAN_POINT('Ctrl Pts',(7.89797053557262,-1.91984155295615,2.34079623538168));
#71978=CARTESIAN_POINT('Ctrl Pts',(7.84315157048059,-2.12241866863442,2.33257558718965));
#71979=CARTESIAN_POINT('Ctrl Pts',(7.78833876393394,-2.32497302612382,2.32435586253265));
#71980=CARTESIAN_POINT('Ctrl Pts',(7.72567172454593,-2.52541544615141,2.31613613787566));
#71981=CARTESIAN_POINT('Ctrl Pts',(7.65533987497481,-2.72313403289677,2.30791641321866));
#71982=CARTESIAN_POINT('Ctrl Pts',(7.58500239023559,-2.9208684613622,2.29969602997624));
#71983=CARTESIAN_POINT('Ctrl Pts',(7.50699896457821,-3.11587834148089,2.29147564673383));
#71984=CARTESIAN_POINT('Ctrl Pts',(7.4215682120023,-3.30756902227254,2.28325526349142));
#71985=CARTESIAN_POINT('Ctrl Pts',(7.33613777583018,-3.49925899311308,2.27503491069425));
#71986=CARTESIAN_POINT('Ctrl Pts',(7.24328019034877,-3.68762952072127,2.26681455789709));
#71987=CARTESIAN_POINT('Ctrl Pts',(7.14328155724583,-3.87210745672321,2.25859420509993));
#71988=CARTESIAN_POINT('Ctrl Pts',(7.04326154383628,-4.05662483521265,2.25037209474211));
#71989=CARTESIAN_POINT('Ctrl Pts',(6.93609757323777,-4.23724769987652,2.24214998438428));
#71990=CARTESIAN_POINT('Ctrl Pts',(6.82212144050659,-4.41342798893108,2.23392787402646));
#71991=CARTESIAN_POINT('Ctrl Pts',(6.77213705497226,-4.49069209046385,2.23032205652605));
#71992=CARTESIAN_POINT('Ctrl Pts',(6.72084308082629,-4.56710211611093,2.22671623902564));
#71993=CARTESIAN_POINT('Ctrl Pts',(6.66827014779923,-4.64261357410561,2.22311042152523));
#71994=CARTESIAN_POINT('Ctrl Pts',(6.54839087633042,-4.81479834772838,2.21488826707978));
#71995=CARTESIAN_POINT('Ctrl Pts',(6.42181915258924,-4.98236585834492,2.20666611263434));
#71996=CARTESIAN_POINT('Ctrl Pts',(6.28893556637754,-5.14480096840019,2.19844395818889));
#71997=CARTESIAN_POINT('Ctrl Pts',(6.15607647469026,-5.30720613667798,2.19022331933892));
#71998=CARTESIAN_POINT('Ctrl Pts',(6.01690802944503,-5.46448056427156,2.18200268048895));
#71999=CARTESIAN_POINT('Ctrl Pts',(5.87185147584527,-5.61614171901971,2.17378204163899));
#72000=CARTESIAN_POINT('Ctrl Pts',(5.72681121825511,-5.76778583578114,2.16556232631578));
#72001=CARTESIAN_POINT('Ctrl Pts',(5.57588437683982,-5.91381772545637,2.15734261099258));
#72002=CARTESIAN_POINT('Ctrl Pts',(5.41953003628161,-6.05379069247868,2.14912289566938));
#72003=CARTESIAN_POINT('Ctrl Pts',(5.26316316664825,-6.19377487589456,2.14090252167926));
#72004=CARTESIAN_POINT('Ctrl Pts',(5.10136814694562,-6.32769896764435,2.13268214768914));
#72005=CARTESIAN_POINT('Ctrl Pts',(4.9346390076379,-6.45515494986746,2.12446177369903));
#72006=CARTESIAN_POINT('Ctrl Pts',(4.76791048454023,-6.58261046102921,2.11624143009039));
#72007=CARTESIAN_POINT('Ctrl Pts',(4.59624811441685,-6.70359773335699,2.10802108648175));
#72008=CARTESIAN_POINT('Ctrl Pts',(4.42017734043375,-6.8177503504907,2.09980074287311));
#72009=CARTESIAN_POINT('Ctrl Pts',(4.24406891810606,-6.93192737631511,2.09157864154896));
#72010=CARTESIAN_POINT('Ctrl Pts',(4.06355045643346,-7.03926666671835,2.08335654022482));
#72011=CARTESIAN_POINT('Ctrl Pts',(3.87917552096256,-7.13944569557503,2.07513443890068));
#72012=CARTESIAN_POINT('Ctrl Pts',(3.79831631354934,-7.1833800668717,2.07152856592969));
#72013=CARTESIAN_POINT('Ctrl Pts',(3.71671571368778,-7.2259378643607,2.06792269295871));
#72014=CARTESIAN_POINT('Ctrl Pts',(3.63442190659676,-7.26709467169305,2.06431681998772));
#72015=CARTESIAN_POINT('Ctrl Pts',(3.44677435505551,-7.36094103022438,2.05609465530618));
#72016=CARTESIAN_POINT('Ctrl Pts',(3.2554590105286,-7.44753096748448,2.04787249062462));
#72017=CARTESIAN_POINT('Ctrl Pts',(3.06105653712331,-7.52659421245989,2.03965032594308));
#72018=CARTESIAN_POINT('Ctrl Pts',(2.86668989789977,-7.60564288371799,2.03142967685204));
#72019=CARTESIAN_POINT('Ctrl Pts',(2.66923753880226,-7.67716752060457,2.02320902776101));
#72020=CARTESIAN_POINT('Ctrl Pts',(2.46930022512807,-7.74094593448905,2.01498837866997));
#72021=CARTESIAN_POINT('Ctrl Pts',(2.26938537354817,-7.80471718314398,2.00676865313337));
#72022=CARTESIAN_POINT('Ctrl Pts',(2.06698640581499,-7.86074385653922,1.99854892759678));
#72023=CARTESIAN_POINT('Ctrl Pts',(1.8627201697933,-7.90885333860385,1.99032920206018));
#72024=CARTESIAN_POINT('Ctrl Pts',(1.65843756831291,-7.95696667511725,1.98210881797335));
#72025=CARTESIAN_POINT('Ctrl Pts',(1.4522876862897,-7.99716148256033,1.97388843388651));
#72026=CARTESIAN_POINT('Ctrl Pts',(1.24489955385584,-8.0293158278467,1.96566804979968));
#72027=CARTESIAN_POINT('Ctrl Pts',(1.03751219006002,-8.06147005396013,1.95744769617988));
#72028=CARTESIAN_POINT('Ctrl Pts',(0.828886877101282,-8.08558383494591,
1.94922734256007));
#72029=CARTESIAN_POINT('Ctrl Pts',(0.619660326089502,-8.10158679782983,
1.94100698894027));
#72030=CARTESIAN_POINT('Ctrl Pts',(0.410389042151422,-8.11759318216938,
1.93278487779747));
#72031=CARTESIAN_POINT('Ctrl Pts',(0.200516557694702,-8.12548526149068,
1.92456276665469));
#72032=CARTESIAN_POINT('Ctrl Pts',(-0.00931671950940989,-8.12524465854645,
1.9163406555119));
#72033=CARTESIAN_POINT('Ctrl Pts',(-0.101339243902614,-8.12513914196395,
1.912734843158));
#72034=CARTESIAN_POINT('Ctrl Pts',(-0.193354211646623,-8.12347016864793,
1.90912903080411));
#72035=CARTESIAN_POINT('Ctrl Pts',(-0.285307631331966,-8.12023935102924,
1.90552321845021));
#72036=CARTESIAN_POINT('Ctrl Pts',(-0.494984716518033,-8.11287226861541,
1.89730105306821));
#72037=CARTESIAN_POINT('Ctrl Pts',(-0.70441090320622,-8.09737835170293,
1.88907888768622));
#72038=CARTESIAN_POINT('Ctrl Pts',(-0.91294698938132,-8.07379807507468,
1.88085672230422));
#72039=CARTESIAN_POINT('Ctrl Pts',(-1.12144463783091,-8.05022214480305,
1.87263607244571));
#72040=CARTESIAN_POINT('Ctrl Pts',(-1.32905222009258,-8.01856286277639,
1.8644154225872));
#72041=CARTESIAN_POINT('Ctrl Pts',(-1.53513588680306,-7.97891254316961,
1.8561947727287));
#72042=CARTESIAN_POINT('Ctrl Pts',(-1.74119640250264,-7.93926667779735,
1.84797504636091));
#72043=CARTESIAN_POINT('Ctrl Pts',(-1.94573305471411,-7.89163162277346,
1.83975531999312));
#72044=CARTESIAN_POINT('Ctrl Pts',(-2.14812158852616,-7.83615091760029,
1.83153559362534));
#72045=CARTESIAN_POINT('Ctrl Pts',(-2.35052633952146,-7.78066576681577,
1.8233152086194));
#72046=CARTESIAN_POINT('Ctrl Pts',(-2.5507823428187,-7.71733378514711,1.81509482361347));
#72047=CARTESIAN_POINT('Ctrl Pts',(-2.74827889416591,-7.64634884650067,
1.80687443860754));
#72048=CARTESIAN_POINT('Ctrl Pts',(-2.94577471470873,-7.57536417052265,
1.79865408401983));
#72049=CARTESIAN_POINT('Ctrl Pts',(-3.14051082688264,-7.49672669655549,
1.79043372943212));
#72050=CARTESIAN_POINT('Ctrl Pts',(-3.33189444944503,-7.41067924958687,
1.78221337484441));
#72051=CARTESIAN_POINT('Ctrl Pts',(-3.52331899161975,-7.32461340486757,
1.77399126266783));
#72052=CARTESIAN_POINT('Ctrl Pts',(-3.71138934292691,-7.23113454303285,
1.76576915049127));
#72053=CARTESIAN_POINT('Ctrl Pts',(-3.89553435227035,-7.13053291646435,
1.75754703831469));
#72054=CARTESIAN_POINT('Ctrl Pts',(-3.97629114251125,-7.08641407510312,
1.7539412311807));
#72055=CARTESIAN_POINT('Ctrl Pts',(-4.05629329600876,-7.04092594081101,
1.7503354240467));
#72056=CARTESIAN_POINT('Ctrl Pts',(-4.13549417314262,-6.9940957604542,1.7467296169127));
#72057=CARTESIAN_POINT('Ctrl Pts',(-4.31609156993985,-6.88731148015273,
1.73850749355601));
#72058=CARTESIAN_POINT('Ctrl Pts',(-4.49258058326739,-6.77351091743634,
1.73028537019933));
#72059=CARTESIAN_POINT('Ctrl Pts',(-4.66441928172336,-6.65303542203011,
1.72206324684263));
#72060=CARTESIAN_POINT('Ctrl Pts',(-4.83622630117851,-6.53258213665777,
1.71384263926006));
#72061=CARTESIAN_POINT('Ctrl Pts',(-5.00338447526566,-6.40545654394141,
1.70562203167748));
#72062=CARTESIAN_POINT('Ctrl Pts',(-5.16538137421267,-6.27204295436796,
1.69740142409492));
#72063=CARTESIAN_POINT('Ctrl Pts',(-5.32736007243909,-6.13864435411519,
1.68918174011634));
#72064=CARTESIAN_POINT('Ctrl Pts',(-5.48417842547541,-5.99895935498211,
1.68096205613776));
#72065=CARTESIAN_POINT('Ctrl Pts',(-5.63535693628535,-5.85341265956541,
1.67274237215917));
#72066=CARTESIAN_POINT('Ctrl Pts',(-5.78654756365206,-5.70785429896699,
1.66452202939472));
#72067=CARTESIAN_POINT('Ctrl Pts',(-5.93209723108903,-5.5564335061223,1.65630168663026));
#72068=CARTESIAN_POINT('Ctrl Pts',(-6.07156242213258,-5.39961270061543,
1.6480813438658));
#72069=CARTESIAN_POINT('Ctrl Pts',(-6.21102709986354,-5.24279247229988,
1.63986103135696));
#72070=CARTESIAN_POINT('Ctrl Pts',(-6.34440715185304,-5.08057249340363,
1.63164071884812));
#72071=CARTESIAN_POINT('Ctrl Pts',(-6.47129821992731,-4.91344959384602,
1.62342040633928));
#72072=CARTESIAN_POINT('Ctrl Pts',(-6.59821642662373,-4.74629095114831,
1.61519833572439));
#72073=CARTESIAN_POINT('Ctrl Pts',(-6.71864269829153,-4.57422752799915,
1.60697626510949));
#72074=CARTESIAN_POINT('Ctrl Pts',(-6.83221436141168,-4.39778745305181,
1.59875419449459));
#72075=CARTESIAN_POINT('Ctrl Pts',(-6.88202495260671,-4.32040385046845,
1.59514813478812));
#72076=CARTESIAN_POINT('Ctrl Pts',(-6.93051758438691,-4.24217875673097,
1.59154207508164));
#72077=CARTESIAN_POINT('Ctrl Pts',(-6.97766433109251,-4.16315842181141,
1.58793601537516));
#72078=CARTESIAN_POINT('Ctrl Pts',(-7.0851647931161,-3.98298220379674,1.57971374954309));
#72079=CARTESIAN_POINT('Ctrl Pts',(-7.18570052831571,-3.79861025402686,
1.57149148371102));
#72080=CARTESIAN_POINT('Ctrl Pts',(-7.27895895856883,-3.61060161773223,
1.56326921787894));
#72081=CARTESIAN_POINT('Ctrl Pts',(-7.37220020351639,-3.42262762694744,
1.55504846721446));
#72082=CARTESIAN_POINT('Ctrl Pts',(-7.45816668895786,-3.23101855143005,
1.54682771654997));
#72083=CARTESIAN_POINT('Ctrl Pts',(-7.53659229682653,-3.03635704651397,
1.53860696588548));
#72084=CARTESIAN_POINT('Ctrl Pts',(-7.61500909493637,-2.84171740844671,
1.53038713867996));
#72085=CARTESIAN_POINT('Ctrl Pts',(-7.68588659637947,-2.64402629917056,
1.52216731147444));
#72086=CARTESIAN_POINT('Ctrl Pts',(-7.74900692705355,-2.4438860871522,1.51394748426891));
#72087=CARTESIAN_POINT('Ctrl Pts',(-7.81213231003214,-2.24372985542539,
1.50572699912847));
#72088=CARTESIAN_POINT('Ctrl Pts',(-7.86749919024205,-2.04112440991499,
1.49750651398802));
#72089=CARTESIAN_POINT('Ctrl Pts',(-7.91493933402158,-1.8366880250217,1.48928602884758));
#72090=CARTESIAN_POINT('Ctrl Pts',(-7.9623792988666,-1.63225241122055,1.48106557471312));
#72091=CARTESIAN_POINT('Ctrl Pts',(-8.00189252297233,-1.42598615994298,
1.47284512057865));
#72092=CARTESIAN_POINT('Ctrl Pts',(-8.03336162146412,-1.21851902787254,
1.46462466644419));
#72093=CARTESIAN_POINT('Ctrl Pts',(-8.06483744242478,-1.01100757640927,
1.45640245624585));
#72094=CARTESIAN_POINT('Ctrl Pts',(-8.08826566048024,-0.802295023498583,
1.44818024604752));
#72095=CARTESIAN_POINT('Ctrl Pts',(-8.10358046933688,-0.593018667060264,
1.43995803584918));
#72096=CARTESIAN_POINT('Ctrl Pts',(-8.11029558120164,-0.501256885552666,
1.436352828512));
#72097=CARTESIAN_POINT('Ctrl Pts',(-8.11545150101203,-0.409386774614503,
1.43274762117482));
#72098=CARTESIAN_POINT('Ctrl Pts',(-8.11904583497314,-0.317462268789904,
1.42914241383765));
#72099=CARTESIAN_POINT('Ctrl Pts',(-8.12317994770551,-0.211733008777547,
1.42499579482097));
#72100=CARTESIAN_POINT('Ctrl Pts',(-8.12524860804669,-0.105922731453665,
1.42084917580429));
#72101=CARTESIAN_POINT('Ctrl Pts',(-8.12524999929771,-0.000106829522945291,
1.41670255678761));
#72102=CARTESIAN_POINT('Ctrl Pts',(-8.12583419228576,-0.000106543491459244,
1.4167025452787));
#72103=CARTESIAN_POINT('Ctrl Pts',(-8.12502534027835,1.24489697938662,1.36791796761918));
#72104=CARTESIAN_POINT('Ctrl Pts',(-7.51929797608287,3.84148931606845,1.26620218944715));
#72105=CARTESIAN_POINT('Ctrl Pts',(-4.86711214124423,6.93200738973815,1.11155521076262));
#72106=CARTESIAN_POINT('Ctrl Pts',(-0.95745427596839,8.41576571390258,0.9527616092251));
#72107=CARTESIAN_POINT('Ctrl Pts',(2.54915990794148,7.93533015430886,0.818359934053017));
#72108=CARTESIAN_POINT('Ctrl Pts',(4.36820127080559,6.88883045742807,0.736889459393433));
#72109=CARTESIAN_POINT('Ctrl Pts',(4.94635496517363,6.44534386149931,0.708350185246352));
#72110=CARTESIAN_POINT('',(-8.12531588310525,3.02062580826617E-5,1.58329744321239));
#72111=CARTESIAN_POINT('Ctrl Pts',(-8.12593926228046,3.02085755239396E-5,
1.58329744321239));
#72112=CARTESIAN_POINT('Ctrl Pts',(-8.12594527009992,0.0285713546895934,
1.58217903602426));
#72113=CARTESIAN_POINT('Ctrl Pts',(-8.11883025624699,1.40788508355762,1.52812942832363));
#72114=CARTESIAN_POINT('Ctrl Pts',(-7.39463807035817,4.13048620871564,1.42114862011048));
#72115=CARTESIAN_POINT('Ctrl Pts',(-4.51728121963489,7.16489725681085,1.26235501857297));
#72116=CARTESIAN_POINT('Ctrl Pts',(-0.538848536700319,8.45288342237417,
1.10356141703545));
#72117=CARTESIAN_POINT('Ctrl Pts',(2.8034090240862,7.82474427555336,0.974423216584827));
#72118=CARTESIAN_POINT('Ctrl Pts',(4.47503875958309,6.80730634394467,0.898216216646709));
#72119=CARTESIAN_POINT('Ctrl Pts',(4.94636091871776,6.44535235552155,0.874940417221097));
#72120=CARTESIAN_POINT('Ctrl Pts',(4.94675954817621,6.44587135576157,2.87494842260024));
#72121=CARTESIAN_POINT('Ctrl Pts',(5.11318684010766,6.3181499430928,2.86672929304954));
#72122=CARTESIAN_POINT('Ctrl Pts',(5.2746458763742,6.18399423460548,2.85851016349884));
#72123=CARTESIAN_POINT('Ctrl Pts',(5.43064894709995,6.04381829441142,2.85029103394814));
#72124=CARTESIAN_POINT('Ctrl Pts',(5.58670953802513,5.9035906696704,2.842068873906));
#72125=CARTESIAN_POINT('Ctrl Pts',(5.73736164193147,5.75729209116024,2.83384671386386));
#72126=CARTESIAN_POINT('Ctrl Pts',(5.88214107051609,5.60536385875599,2.82562455382172));
#72127=CARTESIAN_POINT('Ctrl Pts',(6.02689381201688,5.45346363116923,2.81740390936419));
#72128=CARTESIAN_POINT('Ctrl Pts',(6.1657758352205,5.29593603437041,2.80918326490666));
#72129=CARTESIAN_POINT('Ctrl Pts',(6.29836032883316,5.13325868534605,2.80096262044913));
#72130=CARTESIAN_POINT('Ctrl Pts',(6.43092992747311,4.97059961202352,2.79274289952551));
#72131=CARTESIAN_POINT('Ctrl Pts',(6.55720322257782,4.80279217018242,2.78452317860188));
#72132=CARTESIAN_POINT('Ctrl Pts',(6.67679363853073,4.63034710048561,2.77630345767825));
#72133=CARTESIAN_POINT('Ctrl Pts',(6.79639363680517,4.45788821342652,2.7680830781399));
#72134=CARTESIAN_POINT('Ctrl Pts',(6.90930951555532,4.28079119700873,2.75986269860155));
#72135=CARTESIAN_POINT('Ctrl Pts',(7.01519739680621,4.09959669313255,2.7516423190632));
#72136=CARTESIAN_POINT('Ctrl Pts',(7.12108488619231,3.9184028598123,2.74342196994644));
#72137=CARTESIAN_POINT('Ctrl Pts',(7.21994428349637,3.73311182553568,2.73520162082968));
#72138=CARTESIAN_POINT('Ctrl Pts',(7.31147687342435,3.54429026631298,2.72698127171291));
#72139=CARTESIAN_POINT('Ctrl Pts',(7.40302903423637,3.35542833453178,2.71875916497627));
#72140=CARTESIAN_POINT('Ctrl Pts',(7.4872511292024,3.16303463535269,2.71053705823964));
#72141=CARTESIAN_POINT('Ctrl Pts',(7.56389147054215,2.96769833109091,2.70231495150299));
#72142=CARTESIAN_POINT('Ctrl Pts',(7.59750241650546,2.88203276838012,2.69870911180553));
#72143=CARTESIAN_POINT('Ctrl Pts',(7.62965578754156,2.79580151722597,2.69510327210807));
#72144=CARTESIAN_POINT('Ctrl Pts',(7.66033330596529,2.70905540807473,2.69149743241061));
#72145=CARTESIAN_POINT('Ctrl Pts',(7.73028524070325,2.51125394048837,2.68327527246571));
#72146=CARTESIAN_POINT('Ctrl Pts',(7.79258332089186,2.31070898626016,2.67505311252082));
#72147=CARTESIAN_POINT('Ctrl Pts',(7.84703106126773,2.10803014352249,2.66683095257592));
#72148=CARTESIAN_POINT('Ctrl Pts',(7.90146876533037,1.90538866043161,2.65861030821591));
#72149=CARTESIAN_POINT('Ctrl Pts',(7.94805894115351,1.70061435877334,2.65038966385591));
#72150=CARTESIAN_POINT('Ctrl Pts',(7.98665530036555,1.49433084544318,2.6421690194959));
#72151=CARTESIAN_POINT('Ctrl Pts',(8.02524732353679,1.28807050667525,2.63394929866988));
#72152=CARTESIAN_POINT('Ctrl Pts',(8.05584726873433,1.08030158472424,2.62572957784385));
#72153=CARTESIAN_POINT('Ctrl Pts',(8.0783600269179,0.871657523339884,2.61750985701782));
#72154=CARTESIAN_POINT('Ctrl Pts',(8.10087458896488,0.662996744084499,2.6092894775762));
#72155=CARTESIAN_POINT('Ctrl Pts',(8.11530063485901,0.453460978442835,2.60106909813458));
#72156=CARTESIAN_POINT('Ctrl Pts',(8.12159485509865,0.243689499435362,2.59284871869296));
#72157=CARTESIAN_POINT('Ctrl Pts',(8.1278890520454,0.0339187967250488,2.58462836967234));
#72158=CARTESIAN_POINT('Ctrl Pts',(8.12605147735175,-0.176087322514969,
2.57640802065172));
#72159=CARTESIAN_POINT('Ctrl Pts',(8.11609093552446,-0.38568833116607,2.56818767163109));
#72160=CARTESIAN_POINT('Ctrl Pts',(8.10612826399912,-0.595334155337057,
2.55996556498908));
#72161=CARTESIAN_POINT('Ctrl Pts',(8.08803916956429,-0.804574401001969,
2.55174345834707));
#72162=CARTESIAN_POINT('Ctrl Pts',(8.06188451092087,-1.0127712945548,2.54352135170506));
#72163=CARTESIAN_POINT('Ctrl Pts',(8.05041427273469,-1.10407693884677,2.53991551142774));
#72164=CARTESIAN_POINT('Ctrl Pts',(8.03739345750648,-1.19518198281216,2.53630967115042));
#72165=CARTESIAN_POINT('Ctrl Pts',(8.02283033388594,-1.28603304630154,2.5327038308731));
#72166=CARTESIAN_POINT('Ctrl Pts',(7.98962300227551,-1.49319474258745,2.52448167078277));
#72167=CARTESIAN_POINT('Ctrl Pts',(7.94838205632125,-1.69910374035563,2.51625951069245));
#72168=CARTESIAN_POINT('Ctrl Pts',(7.89922660659719,-1.90313073122343,2.50803735060213));
#72169=CARTESIAN_POINT('Ctrl Pts',(7.85008021766045,-2.10712011394843,2.49981670609643));
#72170=CARTESIAN_POINT('Ctrl Pts',(7.793022305761,-2.30922789536695,2.49159606159073));
#72171=CARTESIAN_POINT('Ctrl Pts',(7.72822276287901,-2.50883648128345,2.48337541708503));
#72172=CARTESIAN_POINT('Ctrl Pts',(7.66343049978985,-2.70842264251782,2.47515569611346));
#72173=CARTESIAN_POINT('Ctrl Pts',(7.59089843314881,-2.90550988817235,2.46693597514187));
#72174=CARTESIAN_POINT('Ctrl Pts',(7.51084610308596,-3.09949647172866,2.4587162541703));
#72175=CARTESIAN_POINT('Ctrl Pts',(7.43078735874187,-3.29349859867395,2.45049587458451));
#72176=CARTESIAN_POINT('Ctrl Pts',(7.3432072570489,-3.48439929322881,2.44227549499874));
#72177=CARTESIAN_POINT('Ctrl Pts',(7.24837361356307,-3.67161647244134,2.43405511541295));
#72178=CARTESIAN_POINT('Ctrl Pts',(7.15354032103805,-3.85883295879963,2.42583476624919));
#72179=CARTESIAN_POINT('Ctrl Pts',(7.05145367616815,-4.04236569499885,2.41761441708542));
#72180=CARTESIAN_POINT('Ctrl Pts',(6.94242785718441,-4.22165642968372,2.40939406792166));
#72181=CARTESIAN_POINT('Ctrl Pts',(6.83337872704452,-4.40098549908922,2.40117196113897));
#72182=CARTESIAN_POINT('Ctrl Pts',(6.71738761205256,-4.57607050274914,2.39294985435627));
#72183=CARTESIAN_POINT('Ctrl Pts',(6.59481308323288,-4.74638051147613,2.38472774757358));
#72184=CARTESIAN_POINT('Ctrl Pts',(6.54105750954748,-4.82107068007513,2.38112190816092));
#72185=CARTESIAN_POINT('Ctrl Pts',(6.48603630710692,-4.89484285566418,2.37751606874826));
#72186=CARTESIAN_POINT('Ctrl Pts',(6.42978227541665,-4.96765411972672,2.3739102293356));
#72187=CARTESIAN_POINT('Ctrl Pts',(6.30150988326345,-5.13368088681117,2.36568806937151));
#72188=CARTESIAN_POINT('Ctrl Pts',(6.16678229109025,-5.29476411247359,2.35746590940743));
#72189=CARTESIAN_POINT('Ctrl Pts',(6.02600517238921,-5.45040817048031,2.34924374944334));
#72190=CARTESIAN_POINT('Ctrl Pts',(5.88525400302796,-5.60602353873556,2.34102310506378));
#72191=CARTESIAN_POINT('Ctrl Pts',(5.7384557306157,-5.75620152160216,2.33280246068421));
#72192=CARTESIAN_POINT('Ctrl Pts',(5.58605501672273,-5.90048107467915,2.32458181630465));
#72193=CARTESIAN_POINT('Ctrl Pts',(5.4336714240135,-6.04474441892959,2.31636209545858));
#72194=CARTESIAN_POINT('Ctrl Pts',(5.27568686061463,-6.18311045349229,2.30814237461251));
#72195=CARTESIAN_POINT('Ctrl Pts',(5.11258200345081,-6.31515580334253,2.29992265376643));
#72196=CARTESIAN_POINT('Ctrl Pts',(4.94946407729784,-6.44721173349845,2.29170227430452));
#72197=CARTESIAN_POINT('Ctrl Pts',(4.78122526530201,-6.57294577915914,2.28348189484261));
#72198=CARTESIAN_POINT('Ctrl Pts',(4.60837922868544,-6.69197492875762,2.2752615153807));
#72199=CARTESIAN_POINT('Ctrl Pts',(4.43553383171244,-6.81100363787027,2.26704116633957));
#72200=CARTESIAN_POINT('Ctrl Pts',(4.25808148881973,-6.92332733535738,2.25882081729844));
#72201=CARTESIAN_POINT('Ctrl Pts',(4.07656517178318,-7.02860611805103,2.25060046825732));
#72202=CARTESIAN_POINT('Ctrl Pts',(3.89501004410986,-7.13390741076836,2.2423783615947));
#72203=CARTESIAN_POINT('Ctrl Pts',(3.70938946169537,-7.23216063129356,2.23415625493207));
#72204=CARTESIAN_POINT('Ctrl Pts',(3.52027230707397,-7.32307110757147,2.22593414826945));
#72205=CARTESIAN_POINT('Ctrl Pts',(3.43733416743192,-7.36294028703093,2.22232830811232));
#72206=CARTESIAN_POINT('Ctrl Pts',(3.35372384018368,-7.40139783865352,2.21872246795519));
#72207=CARTESIAN_POINT('Ctrl Pts',(3.2694906609304,-7.43842176678554,2.21511662779806));
#72208=CARTESIAN_POINT('Ctrl Pts',(3.07741928968188,-7.52284499179453,2.20689446796006));
#72209=CARTESIAN_POINT('Ctrl Pts',(2.88204457163584,-7.59983880869683,2.19867230812206));
#72210=CARTESIAN_POINT('Ctrl Pts',(2.6839598612744,-7.66916208105996,2.19045014828406));
#72211=CARTESIAN_POINT('Ctrl Pts',(2.48591166375443,-7.7384725751039,2.18222950403209));
#72212=CARTESIAN_POINT('Ctrl Pts',(2.28515474935039,-7.80011524912847,2.17400885978011));
#72213=CARTESIAN_POINT('Ctrl Pts',(2.0823001640475,-7.85389798694303,2.16578821552814));
#72214=CARTESIAN_POINT('Ctrl Pts',(1.8794683681093,-7.90767468262437,2.15756849481092));
#72215=CARTESIAN_POINT('Ctrl Pts',(1.67453965692389,-7.95359312935804,2.1493487740937));
#72216=CARTESIAN_POINT('Ctrl Pts',(1.46813868038228,-7.99151152021102,2.14112905337648));
#72217=CARTESIAN_POINT('Ctrl Pts',(1.26172116570797,-8.0294329493218,2.13290867404401));
#72218=CARTESIAN_POINT('Ctrl Pts',(1.05383143976939,-8.05935298572509,2.12468829471154));
#72219=CARTESIAN_POINT('Ctrl Pts',(0.845103805785858,-8.08118104734365,
2.11646791537907));
#72220=CARTESIAN_POINT('Ctrl Pts',(0.636376944235713,-8.10300902818362,
2.10824756646755));
#72221=CARTESIAN_POINT('Ctrl Pts',(0.426812474664166,-8.11674506609866,
2.10002721755604));
#72222=CARTESIAN_POINT('Ctrl Pts',(0.217049814348368,-8.12235045664685,
2.09180686864453));
#72223=CARTESIAN_POINT('Ctrl Pts',(0.00724230392923697,-8.12795704570361,
2.08358476211087));
#72224=CARTESIAN_POINT('Ctrl Pts',(-0.202763186794446,-8.12542950643695,
2.0753626555772));
#72225=CARTESIAN_POINT('Ctrl Pts',(-0.412326127505104,-8.11478124949013,
2.06714054904354));
#72226=CARTESIAN_POINT('Ctrl Pts',(-0.504230875448006,-8.11011140964436,
2.06353470811588));
#72227=CARTESIAN_POINT('Ctrl Pts',(-0.596050525226838,-8.10388038764368,
2.05992886718822));
#72228=CARTESIAN_POINT('Ctrl Pts',(-0.687731230561746,-8.09609247211332,
2.05632302626055));
#72229=CARTESIAN_POINT('Ctrl Pts',(-0.896784683851678,-8.07833420302493,
2.04810086549959));
#72230=CARTESIAN_POINT('Ctrl Pts',(-1.1051844479233,-8.05247155703697,2.03987870473862));
#72231=CARTESIAN_POINT('Ctrl Pts',(-1.31229411584146,-8.01857666397397,
2.03165654397766));
#72232=CARTESIAN_POINT('Ctrl Pts',(-1.51936560747801,-7.98468801871676,
2.02343589879792));
#72233=CARTESIAN_POINT('Ctrl Pts',(-1.72514718645945,-7.94277012905113,
2.01521525361819));
#72234=CARTESIAN_POINT('Ctrl Pts',(-1.92901036318679,-7.89294663488978,
2.00699460843845));
#72235=CARTESIAN_POINT('Ctrl Pts',(-2.13285063729275,-7.84312873805426,
1.99877488679148));
#72236=CARTESIAN_POINT('Ctrl Pts',(-2.33477265282164,-7.78540707987436,
1.99055516514452));
#72237=CARTESIAN_POINT('Ctrl Pts',(-2.53416004363824,-7.71995598664445,
1.98233544349755));
#72238=CARTESIAN_POINT('Ctrl Pts',(-2.7335634105079,-7.65449964910027,1.97411506323968));
#72239=CARTESIAN_POINT('Ctrl Pts',(-2.93043146559177,-7.58131272849055,
1.96589468298181));
#72240=CARTESIAN_POINT('Ctrl Pts',(-3.12416387337227,-7.50061915143114,
1.95767430272394));
#72241=CARTESIAN_POINT('Ctrl Pts',(-3.3178955641178,-7.41992587303171,1.94945395289103));
#72242=CARTESIAN_POINT('Ctrl Pts',(-3.5084913593472,-7.33172610970674,1.94123360305811));
#72243=CARTESIAN_POINT('Ctrl Pts',(-3.69537125251977,-7.23629178989836,
1.9330132532252));
#72244=CARTESIAN_POINT('Ctrl Pts',(-3.88229110286499,-7.14083706508264,
1.92479114578246));
#72245=CARTESIAN_POINT('Ctrl Pts',(-4.06549320098115,-7.038144827766,1.91656903833971));
#72246=CARTESIAN_POINT('Ctrl Pts',(-4.2444214963054,-6.92853330252519,1.90834693089697));
#72247=CARTESIAN_POINT('Ctrl Pts',(-4.32289115682492,-6.88046276589438,
1.90474109550566));
#72248=CARTESIAN_POINT('Ctrl Pts',(-4.40053917807562,-6.83106203178722,
1.90113526011435));
#72249=CARTESIAN_POINT('Ctrl Pts',(-4.47732032824069,-6.78036062763793,
1.89752942472304));
#72250=CARTESIAN_POINT('Ctrl Pts',(-4.65239952191805,-6.66474942700232,
1.88930726666098));
#72251=CARTESIAN_POINT('Ctrl Pts',(-4.82302732827707,-6.54233430842207,
1.88108510859891));
#72252=CARTESIAN_POINT('Ctrl Pts',(-4.98867941096454,-6.4134830862113,1.87286295053685));
#72253=CARTESIAN_POINT('Ctrl Pts',(-5.15430095897274,-6.28465561517034,
1.86464230806672));
#72254=CARTESIAN_POINT('Ctrl Pts',(-5.31494838101878,-6.14939458944456,
1.85642166559659));
#72255=CARTESIAN_POINT('Ctrl Pts',(-5.47012893708334,-6.00810926782989,
1.84820102312646));
#72256=CARTESIAN_POINT('Ctrl Pts',(-5.62529205963782,-5.86683981868753,
1.83998130419119));
#72257=CARTESIAN_POINT('Ctrl Pts',(-5.77498932419644,-5.71954762343952,
1.83176158525592));
#72258=CARTESIAN_POINT('Ctrl Pts',(-5.918762886503,-5.56668064970991,1.82354186632065));
#72259=CARTESIAN_POINT('Ctrl Pts',(-6.06254796907189,-5.4138014270827,1.8153214887572));
#72260=CARTESIAN_POINT('Ctrl Pts',(-6.20040819678272,-5.25534674656431,
1.80710111119376));
#72261=CARTESIAN_POINT('Ctrl Pts',(-6.33192353251545,-5.09180046161249,
1.79888073363031));
#72262=CARTESIAN_POINT('Ctrl Pts',(-6.46343838172507,-4.92825478167791,
1.79066038647704));
#72263=CARTESIAN_POINT('Ctrl Pts',(-6.58860820303355,-4.75961776666391,
1.78244003932377));
#72264=CARTESIAN_POINT('Ctrl Pts',(-6.70705377619678,-4.5864056957169,1.77421969217049));
#72265=CARTESIAN_POINT('Ctrl Pts',(-6.82552467503089,-4.41315658909366,
1.76599758736769));
#72266=CARTESIAN_POINT('Ctrl Pts',(-6.93726828672637,-4.23533071591357,
1.75777548256488));
#72267=CARTESIAN_POINT('Ctrl Pts',(-7.04194857682741,-4.05347354793618,
1.74955337776207));
#72268=CARTESIAN_POINT('Ctrl Pts',(-7.08785672234551,-3.97371903710175,
1.74594752623656));
#72269=CARTESIAN_POINT('Ctrl Pts',(-7.13240694770843,-3.89318953402025,
1.74234167471104));
#72270=CARTESIAN_POINT('Ctrl Pts',(-7.17557366011081,-3.8119326083791,1.73873582318552));
#72271=CARTESIAN_POINT('Ctrl Pts',(-7.27390924468367,-3.62682591762555,
1.73052154190463));
#72272=CARTESIAN_POINT('Ctrl Pts',(-7.36509510738364,-3.43788036080296,
1.72230726062374));
#72273=CARTESIAN_POINT('Ctrl Pts',(-7.44884708413954,-3.24566860286225,
1.71409297934284));
#72274=CARTESIAN_POINT('Ctrl Pts',(-7.53258335119622,-3.05349289886344,
1.70588023884813));
#72275=CARTESIAN_POINT('Ctrl Pts',(-7.60888839697619,-2.8580524879719,1.69766749835342));
#72276=CARTESIAN_POINT('Ctrl Pts',(-7.67752562207033,-2.65994133111119,
1.68945475785871));
#72277=CARTESIAN_POINT('Ctrl Pts',(-7.74615513048944,-2.46185244728693,
1.6812429406975));
#72278=CARTESIAN_POINT('Ctrl Pts',(-7.80711844230906,-2.26109369679558,
1.67303112353629));
#72279=CARTESIAN_POINT('Ctrl Pts',(-7.86022811674692,-2.05827634568374,
1.66481930637508));
#72280=CARTESIAN_POINT('Ctrl Pts',(-7.91334192051017,-1.85544322533877,
1.65660685073763));
#72281=CARTESIAN_POINT('Ctrl Pts',(-7.95860078932263,-1.65055147055819,
1.64839439510018));
#72282=CARTESIAN_POINT('Ctrl Pts',(-7.99586765266581,-1.44422575920546,
1.64018193946274));
#72283=CARTESIAN_POINT('Ctrl Pts',(-8.03313464924543,-1.23789931019728,
1.63196945446413));
#72284=CARTESIAN_POINT('Ctrl Pts',(-8.0624095334704,-1.03013918645309,1.62375696946551));
#72285=CARTESIAN_POINT('Ctrl Pts',(-8.08360659039843,-0.82157900056356,
1.6155444844669));
#72286=CARTESIAN_POINT('Ctrl Pts',(-8.10480806444663,-0.612975354140554,
1.60733028812067));
#72287=CARTESIAN_POINT('Ctrl Pts',(-8.11792831905951,-0.403571607369352,
1.59911609177443));
#72288=CARTESIAN_POINT('Ctrl Pts',(-8.12293352926269,-0.194006292887625,
1.59090189542819));
#72289=CARTESIAN_POINT('Ctrl Pts',(-8.12447808619866,-0.129336569362995,
1.58836707802292));
#72290=CARTESIAN_POINT('Ctrl Pts',(-8.12525024040116,-0.064651475246315,
1.58583226061766));
#72291=CARTESIAN_POINT('Ctrl Pts',(-8.12524999994385,3.02060131589238E-5,
1.58329744321239));
#72292=CARTESIAN_POINT('Origin',(0.,0.,24.4167025567876));
#72293=CARTESIAN_POINT('',(4.94671019697112,6.44580737750965,4.87493507917627));
#72294=CARTESIAN_POINT('',(4.94648442104396,6.445513583535,4.7083419611594));
#72295=CARTESIAN_POINT('',(4.9467595481762,6.44587135576158,24.4167025567876));
#72296=CARTESIAN_POINT('',(-8.12518278065587,-2.09407945338198E-5,3.41670255698467));
#72297=CARTESIAN_POINT('Ctrl Pts',(4.94648442104396,6.445513583535,4.7083419611594));
#72298=CARTESIAN_POINT('Ctrl Pts',(5.64364652292867,5.90964851341047,4.6738994556356));
#72299=CARTESIAN_POINT('Ctrl Pts',(7.19392102387665,4.26498724618048,4.5865257495993));
#72300=CARTESIAN_POINT('Ctrl Pts',(8.43364688506178,0.784339091177833,4.44622084305048));
#72301=CARTESIAN_POINT('Ctrl Pts',(7.78105715559112,-3.34615258666749,4.28742724151297));
#72302=CARTESIAN_POINT('Ctrl Pts',(5.23185395479474,-6.66102783264922,4.12863363997545));
#72303=CARTESIAN_POINT('Ctrl Pts',(1.40739926919892,-8.35229398964753,3.96984003843793));
#72304=CARTESIAN_POINT('Ctrl Pts',(-2.76010551353616,-8.00770910714061,
3.81104643690042));
#72305=CARTESIAN_POINT('Ctrl Pts',(-6.25484139177157,-5.71126490000266,
3.6522528353629));
#72306=CARTESIAN_POINT('Ctrl Pts',(-7.88570092334897,-2.65791459092136,
3.52080487600157));
#72307=CARTESIAN_POINT('Ctrl Pts',(-8.12461652328501,-0.653270324207159,
3.44228811715276));
#72308=CARTESIAN_POINT('Ctrl Pts',(-8.12455793610677,-2.09859534307796E-5,
3.41670255881645));
#72309=CARTESIAN_POINT('Ctrl Pts',(-8.12524999997303,-2.09359364451616E-5,
3.41670255678761));
#72310=CARTESIAN_POINT('Ctrl Pts',(-8.12525054662003,0.212133106632909,
3.40839391109587));
#72311=CARTESIAN_POINT('Ctrl Pts',(-8.11693759016218,0.424271844703091,
3.40008526540412));
#72312=CARTESIAN_POINT('Ctrl Pts',(-8.10034075105971,0.635741519189564,
3.39177661971238));
#72313=CARTESIAN_POINT('Ctrl Pts',(-8.08374270635953,0.847226554875311,
3.38346737047896));
#72314=CARTESIAN_POINT('Ctrl Pts',(-8.05885960296614,1.05804214951943,3.37515812124554));
#72315=CARTESIAN_POINT('Ctrl Pts',(-8.02577298472956,1.26753917497061,3.36684887201212));
#72316=CARTESIAN_POINT('Ctrl Pts',(-7.9926785791969,1.47708550782921,3.35853766710636));
#72317=CARTESIAN_POINT('Ctrl Pts',(-7.95137684593506,1.6853123734601,3.3502264622006));
#72318=CARTESIAN_POINT('Ctrl Pts',(-7.90200075295423,1.89157914526747,3.34191525729484));
#72319=CARTESIAN_POINT('Ctrl Pts',(-7.88764430434135,1.95155266952234,3.33949871562584));
#72320=CARTESIAN_POINT('Ctrl Pts',(-7.87260558032577,2.01136056062553,3.33708217395684));
#72321=CARTESIAN_POINT('Ctrl Pts',(-7.85688865322471,2.07098726537098,3.33466563228784));
#72322=CARTESIAN_POINT('Ctrl Pts',(-7.80341260928096,2.27386409127254,3.32644347234192));
#72323=CARTESIAN_POINT('Ctrl Pts',(-7.74206565800979,2.47470203848903,3.31822131239599));
#72324=CARTESIAN_POINT('Ctrl Pts',(-7.67302839265335,2.67288661338926,3.30999915245006));
#72325=CARTESIAN_POINT('Ctrl Pts',(-7.6040038528869,2.87103465706786,3.30177850808903));
#72326=CARTESIAN_POINT('Ctrl Pts',(-7.52729192531106,3.06653002601864,3.29355786372799));
#72327=CARTESIAN_POINT('Ctrl Pts',(-7.44312258174497,3.25877489182945,3.28533721936695));
#72328=CARTESIAN_POINT('Ctrl Pts',(-7.35896269403651,3.45099816022721,3.27711749853983));
#72329=CARTESIAN_POINT('Ctrl Pts',(-7.26734718125301,3.63997138426629,3.2688977777127));
#72330=CARTESIAN_POINT('Ctrl Pts',(-7.16855385840787,3.82511740232971,3.26067805688557));
#72331=CARTESIAN_POINT('Ctrl Pts',(-7.06975261962332,4.01027825545101,3.25245767744295));
#72332=CARTESIAN_POINT('Ctrl Pts',(-6.96377255814811,4.19161102817368,3.24423729800033));
#72333=CARTESIAN_POINT('Ctrl Pts',(-6.85093758982922,4.36856288758271,3.23601691855772));
#72334=CARTESIAN_POINT('Ctrl Pts',(-6.73810303907606,4.54551409215014,3.22779656953607));
#72335=CARTESIAN_POINT('Ctrl Pts',(-6.61841379315987,4.71808416841445,3.21957622051443));
#72336=CARTESIAN_POINT('Ctrl Pts',(-6.49223755427729,4.8857485712357,3.21135587149278));
#72337=CARTESIAN_POINT('Ctrl Pts',(-6.36603433721458,5.05344882296558,3.20313376484974));
#72338=CARTESIAN_POINT('Ctrl Pts',(-6.23334153372333,5.2162410698821,3.19491165820669));
#72339=CARTESIAN_POINT('Ctrl Pts',(-6.09456832782582,5.3736323339025,3.18668955156365));
#72340=CARTESIAN_POINT('Ctrl Pts',(-6.03370874084892,5.44265695043495,3.18308371129255));
#72341=CARTESIAN_POINT('Ctrl Pts',(-5.97168022833068,5.51064323045342,3.17947787102145));
#72342=CARTESIAN_POINT('Ctrl Pts',(-5.90851966259576,5.57755169937665,3.17587203075034));
#72343=CARTESIAN_POINT('Ctrl Pts',(-5.76449878431245,5.73011867446293,3.16764987066119));
#72344=CARTESIAN_POINT('Ctrl Pts',(-5.61454171433746,5.87712958608984,3.15942771057204));
#72345=CARTESIAN_POINT('Ctrl Pts',(-5.45910102793138,6.01813123231278,3.15120555048289));
#72346=CARTESIAN_POINT('Ctrl Pts',(-5.3036889937906,6.15910688780788,3.14298490597835));
#72347=CARTESIAN_POINT('Ctrl Pts',(-5.14279557911143,6.29407529048464,3.13476426147381));
#72348=CARTESIAN_POINT('Ctrl Pts',(-4.97690874665384,6.42262149670838,3.12654361696927));
#72349=CARTESIAN_POINT('Ctrl Pts',(-4.81104055046561,6.55115326163084,3.11832389599883));
#72350=CARTESIAN_POINT('Ctrl Pts',(-4.64018028965452,6.67326408979431,3.11010417502838));
#72351=CARTESIAN_POINT('Ctrl Pts',(-4.46484805175013,6.78858007519121,3.10188445405793));
#72352=CARTESIAN_POINT('Ctrl Pts',(-4.28950176515715,6.90390530040838,3.0936640744733));
#72353=CARTESIAN_POINT('Ctrl Pts',(-4.10968303060545,7.01243443053628,3.08544369488865));
#72354=CARTESIAN_POINT('Ctrl Pts',(-3.92594077841907,7.11383697921496,3.07722331530401));
#72355=CARTESIAN_POINT('Ctrl Pts',(-3.7421992062265,7.21523915262283,3.06900296614138));
#72356=CARTESIAN_POINT('Ctrl Pts',(-3.55453440513977,7.30951465706955,3.06078261697875));
#72357=CARTESIAN_POINT('Ctrl Pts',(-3.36352022173331,7.39637879509231,3.05256226781611));
#72358=CARTESIAN_POINT('Ctrl Pts',(-3.17246519697824,7.48326150581202,3.04434016103454));
#72359=CARTESIAN_POINT('Ctrl Pts',(-2.97805962791343,7.56272956208721,3.03611805425296));
#72360=CARTESIAN_POINT('Ctrl Pts',(-2.78089868479704,7.63454583242475,3.02789594747139));
#72361=CARTESIAN_POINT('Ctrl Pts',(-2.69443292613379,7.66604115903938,3.02429010805187));
#72362=CARTESIAN_POINT('Ctrl Pts',(-2.60743747384918,7.69606544792564,3.02068426863235));
#72363=CARTESIAN_POINT('Ctrl Pts',(-2.5199635922462,7.72460167621953,3.01707842921283));
#72364=CARTESIAN_POINT('Ctrl Pts',(-2.32050261699057,7.78967097257762,3.00885626924859));
#72365=CARTESIAN_POINT('Ctrl Pts',(-2.11848709807292,7.84702129777551,3.00063410928435));
#72366=CARTESIAN_POINT('Ctrl Pts',(-1.91453127864162,7.89647120843246,2.99241194932011));
#72367=CARTESIAN_POINT('Ctrl Pts',(-1.71061305423132,7.94591200402502,2.98419130494036));
#72368=CARTESIAN_POINT('Ctrl Pts',(-1.504755529824,7.98745522209652,2.97597066056061));
#72369=CARTESIAN_POINT('Ctrl Pts',(-1.2975857193745,8.02096994529809,2.96775001618086));
#72370=CARTESIAN_POINT('Ctrl Pts',(-1.09043918304662,8.05448090334806,2.95953029533469));
#72371=CARTESIAN_POINT('Ctrl Pts',(-0.881980946243665,8.07996512008632,
2.95131057448853));
#72372=CARTESIAN_POINT('Ctrl Pts',(-0.672846598932096,8.09734308380258,
2.94309085364236));
#72373=CARTESIAN_POINT('Ctrl Pts',(-0.463695494457813,8.11472243995089,
2.93487047418033));
#72374=CARTESIAN_POINT('Ctrl Pts',(-0.253868465142897,8.12399421810081,
2.92665009471829));
#72375=CARTESIAN_POINT('Ctrl Pts',(-0.0440056553494257,8.12513083370337,
2.91842971525625));
#72376=CARTESIAN_POINT('Ctrl Pts',(0.165856377813637,8.12626744509971,2.91020936621502));
#72377=CARTESIAN_POINT('Ctrl Pts',(0.375753896036386,8.11926895524163,2.9019890171738));
#72378=CARTESIAN_POINT('Ctrl Pts',(0.585046782080702,8.10415990866894,2.89376866813257));
#72379=CARTESIAN_POINT('Ctrl Pts',(0.794384417767329,8.08904763157828,2.88554656146983));
#72380=CARTESIAN_POINT('Ctrl Pts',(1.00311686856462,8.06582135454113,2.87732445480709));
#72381=CARTESIAN_POINT('Ctrl Pts',(1.21060804928841,8.03455759289198,2.86910234814435));
#72382=CARTESIAN_POINT('Ctrl Pts',(1.30160419689751,8.02084673607426,2.865496507988));
#72383=CARTESIAN_POINT('Ctrl Pts',(1.39236169515423,8.00559070101045,2.86189066783166));
#72384=CARTESIAN_POINT('Ctrl Pts',(1.48282738326404,7.98879906581348,2.85828482767532));
#72385=CARTESIAN_POINT('Ctrl Pts',(1.68910954411817,7.95051035254463,2.85006269932273));
#72386=CARTESIAN_POINT('Ctrl Pts',(1.89394194825558,7.90422130195749,2.84184057097013));
#72387=CARTESIAN_POINT('Ctrl Pts',(2.09669841206705,7.85006645394391,2.83361844261754));
#72388=CARTESIAN_POINT('Ctrl Pts',(2.29941724410512,7.79592165711652,2.82539784029901));
#72389=CARTESIAN_POINT('Ctrl Pts',(2.5000606198312,7.73391405278821,2.81717723798048));
#72390=CARTESIAN_POINT('Ctrl Pts',(2.69801531649065,7.66422865750245,2.80895663566195));
#72391=CARTESIAN_POINT('Ctrl Pts',(2.89989977431968,7.59315988023536,2.80057283941912));
#72392=CARTESIAN_POINT('Ctrl Pts',(3.09898738478772,7.51410537956481,2.79218904317629));
#72393=CARTESIAN_POINT('Ctrl Pts',(3.29464576591258,7.42731424134285,2.78380524693346));
#72394=CARTESIAN_POINT('Ctrl Pts',(3.4864840455747,7.34221764312561,2.77558513880921));
#72395=CARTESIAN_POINT('Ctrl Pts',(3.67502548782356,7.24968384603085,2.76736503068495));
#72396=CARTESIAN_POINT('Ctrl Pts',(3.85969528407515,7.14999579556436,2.7591449225607));
#72397=CARTESIAN_POINT('Ctrl Pts',(4.04988111205948,7.04733009276431,2.75067928225858));
#72398=CARTESIAN_POINT('Ctrl Pts',(4.23596012924437,6.93707627618972,2.74221364195646));
#72399=CARTESIAN_POINT('Ctrl Pts',(4.41733225402655,6.81959407296627,2.73374800165434));
#72400=CARTESIAN_POINT('Ctrl Pts',(4.59870437880873,6.70211186974282,2.72528236135222));
#72401=CARTESIAN_POINT('Ctrl Pts',(4.77536932835898,6.57740147163754,2.71681672105011));
#72402=CARTESIAN_POINT('Ctrl Pts',(4.94675954817618,6.44587135576159,2.70835108074799));
#72403=CARTESIAN_POINT('',(-8.12524999887371,-0.000135288016022189,3.58329744321239));
#72404=CARTESIAN_POINT('Ctrl Pts',(-8.12524999887371,-0.000135288016022189,
3.58329744321239));
#72405=CARTESIAN_POINT('Ctrl Pts',(-8.12525350335822,0.210340211731544,
3.5750539685695));
#72406=CARTESIAN_POINT('Ctrl Pts',(-8.11707446516784,0.420817569687947,
3.56681049392662));
#72407=CARTESIAN_POINT('Ctrl Pts',(-8.1007385130676,0.630652919919719,3.55856701928373));
#72408=CARTESIAN_POINT('Ctrl Pts',(-8.08440281262829,0.840485037566233,
3.55032367163439));
#72409=CARTESIAN_POINT('Ctrl Pts',(-8.05991047461304,1.04967487660205,3.54208032398506));
#72410=CARTESIAN_POINT('Ctrl Pts',(-8.02733908616164,1.25758290314462,3.53383697633572));
#72411=CARTESIAN_POINT('Ctrl Pts',(-7.99475885361346,1.46554738287492,3.52559139037331));
#72412=CARTESIAN_POINT('Ctrl Pts',(-7.95409523049929,1.67222906598806,3.5173458044109));
#72413=CARTESIAN_POINT('Ctrl Pts',(-7.90547731210573,1.87699654509046,3.50910021844849));
#72414=CARTESIAN_POINT('Ctrl Pts',(-7.85902523741095,2.07264198916994,3.5012219589984));
#72415=CARTESIAN_POINT('Ctrl Pts',(-7.80531218040087,2.26653982392757,3.4933436995483));
#72416=CARTESIAN_POINT('Ctrl Pts',(-7.74449383032738,2.45815029534834,3.48546544009821));
#72417=CARTESIAN_POINT('Ctrl Pts',(-7.68102064709461,2.65812491726941,3.47724328009178));
#72418=CARTESIAN_POINT('Ctrl Pts',(-7.60978737587496,2.85567276256273,3.46902112008536));
#72419=CARTESIAN_POINT('Ctrl Pts',(-7.53100486733088,3.05018905163904,3.46079896007893));
#72420=CARTESIAN_POINT('Ctrl Pts',(-7.45223688070886,3.24466948567034,3.45257831565722));
#72421=CARTESIAN_POINT('Ctrl Pts',(-7.3659225448347,3.43611920536153,3.44435767123552));
#72422=CARTESIAN_POINT('Ctrl Pts',(-7.27232120155027,3.62395252507292,3.43613702681382));
#72423=CARTESIAN_POINT('Ctrl Pts',(-7.17873037374545,3.81176474297771,3.42791730592607));
#72424=CARTESIAN_POINT('Ctrl Pts',(-7.07785430448506,3.99596110795115,3.41969758503833));
#72425=CARTESIAN_POINT('Ctrl Pts',(-6.969999094814,4.17597894879656,3.41147786415058));
#72426=CARTESIAN_POINT('Ctrl Pts',(-6.86213524311471,4.35601121378771,3.40325748464782));
#72427=CARTESIAN_POINT('Ctrl Pts',(-6.74729128299553,4.53186403107694,3.39503710514507));
#72428=CARTESIAN_POINT('Ctrl Pts',(-6.62581815285298,4.70300131488647,3.38681672564231));
#72429=CARTESIAN_POINT('Ctrl Pts',(-6.50434547224924,4.87413796536377,3.37859637656093));
#72430=CARTESIAN_POINT('Ctrl Pts',(-6.37624384370664,5.04055887813666,3.37037602747954));
#72431=CARTESIAN_POINT('Ctrl Pts',(-6.24190653496301,5.2017583922445,3.36215567839816));
#72432=CARTESIAN_POINT('Ctrl Pts',(-6.10754050310864,5.36299237296134,3.35393357169636));
#72433=CARTESIAN_POINT('Ctrl Pts',(-5.96693631642396,5.51900249787455,3.34571146499456));
#72434=CARTESIAN_POINT('Ctrl Pts',(-5.82052710764396,5.66931669177881,3.33748935829275));
#72435=CARTESIAN_POINT('Ctrl Pts',(-5.75631872560042,5.73523762167929,3.33388351838206));
#72436=CARTESIAN_POINT('Ctrl Pts',(-5.69099435995881,5.80006351310103,3.33027767847137));
#72437=CARTESIAN_POINT('Ctrl Pts',(-5.62459279563755,5.86375676898029,3.32667183856068));
#72438=CARTESIAN_POINT('Ctrl Pts',(-5.47318166809742,6.00899231859359,3.31844967855303));
#72439=CARTESIAN_POINT('Ctrl Pts',(-5.31611724404946,6.14838420077997,3.31022751854539));
#72440=CARTESIAN_POINT('Ctrl Pts',(-5.15387402109143,6.28150221978938,3.30200535853774));
#72441=CARTESIAN_POINT('Ctrl Pts',(-4.99166070430765,6.414595701252,3.29378471411482));
#72442=CARTESIAN_POINT('Ctrl Pts',(-4.82427072192752,6.5414174405494,3.2855640696919));
#72443=CARTESIAN_POINT('Ctrl Pts',(-4.65221201782622,6.66157720841644,3.27734342526898));
#72444=CARTESIAN_POINT('Ctrl Pts',(-4.48017264336145,6.78172347714287,3.26912370438009));
#72445=CARTESIAN_POINT('Ctrl Pts',(-4.3034658361829,6.89520909970062,3.26090398349119));
#72446=CARTESIAN_POINT('Ctrl Pts',(-4.1226295898715,7.00168642736991,3.2526842626023));
#72447=CARTESIAN_POINT('Ctrl Pts',(-3.94177885383763,7.10817228666357,3.24446388309836));
#72448=CARTESIAN_POINT('Ctrl Pts',(-3.75679827050111,7.20764857693053,3.23624350359442));
#72449=CARTESIAN_POINT('Ctrl Pts',(-3.56825248706198,7.29981244629449,3.22802312409047));
#72450=CARTESIAN_POINT('Ctrl Pts',(-3.37970740137907,7.39197597458526,3.2198027750079));
#72451=CARTESIAN_POINT('Ctrl Pts',(-3.18759740831881,7.47682700888961,3.21158242592532));
#72452=CARTESIAN_POINT('Ctrl Pts',(-2.99250976947125,7.55410966574613,3.20336207684274));
#72453=CARTESIAN_POINT('Ctrl Pts',(-2.79738041828228,7.63140884666633,3.1951399701398));
#72454=CARTESIAN_POINT('Ctrl Pts',(-2.59927242383551,7.70113630852653,3.18691786343685));
#72455=CARTESIAN_POINT('Ctrl Pts',(-2.39879198582123,7.76308473296922,3.17869575673391));
#72456=CARTESIAN_POINT('Ctrl Pts',(-2.31087043610211,7.79025247827947,3.17508991683033));
#72457=CARTESIAN_POINT('Ctrl Pts',(-2.22249281008404,7.81592472265312,3.17148407692676));
#72458=CARTESIAN_POINT('Ctrl Pts',(-2.13371115334702,7.84008700695231,3.16787823702318));
#72459=CARTESIAN_POINT('Ctrl Pts',(-1.93126816993193,7.89518267760579,3.15965607701146));
#72460=CARTESIAN_POINT('Ctrl Pts',(-1.72665665855564,7.94244216953387,3.15143391699972));
#72461=CARTESIAN_POINT('Ctrl Pts',(-1.52049910613384,7.9817147299779,3.143211756988));
#72462=CARTESIAN_POINT('Ctrl Pts',(-1.31437955458275,8.02098005133962,3.13499111256102));
#72463=CARTESIAN_POINT('Ctrl Pts',(-1.10671482055134,8.05226132437254,3.12677046813403));
#72464=CARTESIAN_POINT('Ctrl Pts',(-0.898137639883169,8.0754588936063,3.11854982370704));
#72465=CARTESIAN_POINT('Ctrl Pts',(-0.689583891453495,8.09865385674972,
3.11033010281397));
#72466=CARTESIAN_POINT('Ctrl Pts',(-0.480118194254602,8.11376689653932,
3.10211038192091));
#72467=CARTESIAN_POINT('Ctrl Pts',(-0.270379299796881,8.1207501252496,3.09389066102784));
#72468=CARTESIAN_POINT('Ctrl Pts',(-0.0606235997583052,8.12773391349947,
3.08567028151976));
#72469=CARTESIAN_POINT('Ctrl Pts',(0.149405046379006,8.12658657653562,3.07744990201167));
#72470=CARTESIAN_POINT('Ctrl Pts',(0.359065913971908,8.11731231578061,3.06922952250359));
#72471=CARTESIAN_POINT('Ctrl Pts',(0.568726005667304,8.1080380893471,3.06100917341689));
#72472=CARTESIAN_POINT('Ctrl Pts',(0.778018026803319,8.09063701499423,3.05278882433019));
#72473=CARTESIAN_POINT('Ctrl Pts',(0.986303865499881,8.06516535772206,3.04456847524349));
#72474=CARTESIAN_POINT('Ctrl Pts',(1.19463423848764,8.03968825426973,3.03634636853648));
#72475=CARTESIAN_POINT('Ctrl Pts',(1.40195770621676,8.00613715632205,3.02812426182946));
#72476=CARTESIAN_POINT('Ctrl Pts',(1.607642761719,7.96462003570745,3.01990215512245));
#72477=CARTESIAN_POINT('Ctrl Pts',(1.69784681793703,7.94641252581916,3.01629631524352));
#72478=CARTESIAN_POINT('Ctrl Pts',(1.78773587569151,7.92667357721418,3.01269047536459));
#72479=CARTESIAN_POINT('Ctrl Pts',(1.87725731472338,7.90541539305921,3.00908463548566));
#72480=CARTESIAN_POINT('Ctrl Pts',(2.08138547454277,7.85694215514455,3.00086254402858));
#72481=CARTESIAN_POINT('Ctrl Pts',(2.28366885122072,7.80055040854686,2.9926404525715));
#72482=CARTESIAN_POINT('Ctrl Pts',(2.48348871359225,7.7364055847635,2.98441836111442));
#72483=CARTESIAN_POINT('Ctrl Pts',(2.68327103617755,7.67227281174899,2.97619781432639));
#72484=CARTESIAN_POINT('Ctrl Pts',(2.88059048735292,7.6003899589272,2.96797726753835));
#72485=CARTESIAN_POINT('Ctrl Pts',(3.07484378835328,7.52097222702792,2.95975672075032));
#72486=CARTESIAN_POINT('Ctrl Pts',(3.26909078469402,7.44155707270011,2.95153644076727));
#72487=CARTESIAN_POINT('Ctrl Pts',(3.46027155529169,7.35460763648865,2.94331616078422));
#72488=CARTESIAN_POINT('Ctrl Pts',(3.647802165979,7.26038751860939,2.93509588080117));
#72489=CARTESIAN_POINT('Ctrl Pts',(3.83531994853028,7.16617384590983,2.92687616313096));
#72490=CARTESIAN_POINT('Ctrl Pts',(4.0191878067775,7.06469061856965,2.91865644546074));
#72491=CARTESIAN_POINT('Ctrl Pts',(4.19884524925915,6.95624799265192,2.91043672779053));
#72492=CARTESIAN_POINT('Ctrl Pts',(4.37852390560449,6.8477925618815,2.90221603954004));
#72493=CARTESIAN_POINT('Ctrl Pts',(4.55399089994502,6.73237624282856,2.89399535128957));
#72494=CARTESIAN_POINT('Ctrl Pts',(4.72471274193336,6.6103537778785,2.88577466303908));
#72495=CARTESIAN_POINT('Ctrl Pts',(4.79965682014225,6.55678792449998,2.88216591622614));
#72496=CARTESIAN_POINT('Ctrl Pts',(4.87368685165283,6.50194958619583,2.87855716941319));
#72497=CARTESIAN_POINT('Ctrl Pts',(4.94675954817621,6.44587135576157,2.87494842260024));
#72498=CARTESIAN_POINT('Ctrl Pts',(4.94671019697112,6.44580737750965,4.87493507917627));
#72499=CARTESIAN_POINT('Ctrl Pts',(5.75015646111357,5.82789648496184,4.83522813691696));
#72500=CARTESIAN_POINT('Ctrl Pts',(7.356633927154,4.0356546125411,4.74258999414515));
#72501=CARTESIAN_POINT('Ctrl Pts',(8.46217010059878,0.365053444517306,4.59702065086083));
#72502=CARTESIAN_POINT('Ctrl Pts',(7.60550572314025,-3.72798464644211,4.43822704932331));
#72503=CARTESIAN_POINT('Ctrl Pts',(4.89501810258881,-6.91233568369901,4.27943344778579));
#72504=CARTESIAN_POINT('Ctrl Pts',(0.991381904642859,-8.41182196364104,
4.12063984624828));
#72505=CARTESIAN_POINT('Ctrl Pts',(-3.15390118497908,-7.86094740754393,
3.96184624471076));
#72506=CARTESIAN_POINT('Ctrl Pts',(-6.53042864729724,-5.39398632844221,
3.80305264317324));
#72507=CARTESIAN_POINT('Ctrl Pts',(-7.9486544727063,-2.38889033598931,3.67686971310851));
#72508=CARTESIAN_POINT('Ctrl Pts',(-8.12500981392525,-0.518932006235639,
3.6036179835563));
#72509=CARTESIAN_POINT('Ctrl Pts',(-8.12470237155434,-0.000135567501295938,
3.58329745451658));
#72510=CARTESIAN_POINT('Origin',(0.,0.,24.4167025567876));
#72511=CARTESIAN_POINT('',(4.94675954817622,6.44587135576156,6.87494727151379));
#72512=CARTESIAN_POINT('',(4.9467595481762,6.44587135576158,6.70835375129049));
#72513=CARTESIAN_POINT('',(4.9467595481762,6.44587135576158,24.4167025567876));
#72514=CARTESIAN_POINT('',(-8.1252499987303,0.000143642949229983,5.41670255678761));
#72515=CARTESIAN_POINT('Ctrl Pts',(4.9467595481762,6.44587135576158,6.70835375129049));
#72516=CARTESIAN_POINT('Ctrl Pts',(5.11326717757315,6.31808828965565,6.70013160170819));
#72517=CARTESIAN_POINT('Ctrl Pts',(5.27480674507703,6.18386087726778,6.69190945212589));
#72518=CARTESIAN_POINT('Ctrl Pts',(5.43088886988298,6.04360270413941,6.68368730254359));
#72519=CARTESIAN_POINT('Ctrl Pts',(5.52172970930857,5.96197151031037,6.6789019565543));
#72520=CARTESIAN_POINT('Ctrl Pts',(5.61072256014284,5.87829825786018,6.67411661056502));
#72521=CARTESIAN_POINT('Ctrl Pts',(5.69777643160371,5.79267048069897,6.66933126457574));
#72522=CARTESIAN_POINT('Ctrl Pts',(5.84735200294864,5.64554521818103,6.66110910456816));
#72523=CARTESIAN_POINT('Ctrl Pts',(5.99125071310778,5.49259917758122,6.65288694456059));
#72524=CARTESIAN_POINT('Ctrl Pts',(6.12902875487278,5.334294150536,6.64466478455301));
#72525=CARTESIAN_POINT('Ctrl Pts',(6.26678140011208,5.17601830374068,6.63644414013018));
#72526=CARTESIAN_POINT('Ctrl Pts',(6.39841543505899,5.01238566456822,6.62822349570735));
#72527=CARTESIAN_POINT('Ctrl Pts',(6.52352602984438,4.84389261859125,6.62000285128451));
#72528=CARTESIAN_POINT('Ctrl Pts',(6.64862256929821,4.67541850167165,6.61178313039564));
#72529=CARTESIAN_POINT('Ctrl Pts',(6.76719695582161,4.50208530493441,6.60356340950677));
#72530=CARTESIAN_POINT('Ctrl Pts',(6.87888604857588,4.32442068874065,6.59534368861789));
#72531=CARTESIAN_POINT('Ctrl Pts',(6.99058409055312,4.1467418369557,6.58712330911399));
#72532=CARTESIAN_POINT('Ctrl Pts',(7.09539557702665,3.96473112067881,6.57890292961008));
#72533=CARTESIAN_POINT('Ctrl Pts',(7.19300137027119,3.77894414483421,6.57068255010618));
#72534=CARTESIAN_POINT('Ctrl Pts',(7.29060680230357,3.59315785653605,6.56246220102364));
#72535=CARTESIAN_POINT('Ctrl Pts',(7.38100645954513,3.40359559914725,6.55424185194111));
#72536=CARTESIAN_POINT('Ctrl Pts',(7.46392749545489,3.21083694775872,6.54602150285857));
#72537=CARTESIAN_POINT('Ctrl Pts',(7.54686626098896,3.01803708199755,6.53779939615566));
#72538=CARTESIAN_POINT('Ctrl Pts',(7.62232309398686,2.82203972804977,6.52957728945276));
#72539=CARTESIAN_POINT('Ctrl Pts',(7.69007314197288,2.62344480285128,6.52135518274985));
#72540=CARTESIAN_POINT('Ctrl Pts',(7.71978521399354,2.53635015279798,6.51774934284597));
#72541=CARTESIAN_POINT('Ctrl Pts',(7.74801567483915,2.44875614619009,6.51414350294209));
#72542=CARTESIAN_POINT('Ctrl Pts',(7.7747485585597,2.3607143862979,6.5105376630382));
#72543=CARTESIAN_POINT('Ctrl Pts',(7.83570579827994,2.15995854120309,6.50231550303063));
#72544=CARTESIAN_POINT('Ctrl Pts',(7.88889320817592,1.9568072932397,6.49409334302306));
#72545=CARTESIAN_POINT('Ctrl Pts',(7.93414200400985,1.75187848400128,6.4858711830155));
#72546=CARTESIAN_POINT('Ctrl Pts',(7.97938245916653,1.54698744913946,6.47765053859263));
#72547=CARTESIAN_POINT('Ctrl Pts',(8.01668715724014,1.34031979501592,6.46942989416977));
#72548=CARTESIAN_POINT('Ctrl Pts',(8.04593809175954,1.13250509317743,6.4612092497469));
#72549=CARTESIAN_POINT('Ctrl Pts',(8.07518574013385,0.924713737918286,6.45298952885797));
#72550=CARTESIAN_POINT('Ctrl Pts',(8.09638139017429,0.715775884357431,6.44476980796903));
#72551=CARTESIAN_POINT('Ctrl Pts',(8.10945860640715,0.506328622012376,6.43655008708009));
#72552=CARTESIAN_POINT('Ctrl Pts',(8.12253687046756,0.296864577455713,6.42832970757622));
#72553=CARTESIAN_POINT('Ctrl Pts',(8.12749537984046,0.0868913369679979,
6.42010932807234));
#72554=CARTESIAN_POINT('Ctrl Pts',(8.12431970883006,-0.122950523445302,
6.41188894856847));
#72555=CARTESIAN_POINT('Ctrl Pts',(8.12114404957194,-0.332791607291501,
6.40366859948596));
#72556=CARTESIAN_POINT('Ctrl Pts',(8.10983427728161,-0.542501016966194,
6.39544825040345));
#72557=CARTESIAN_POINT('Ctrl Pts',(8.09042808378968,-0.751439274677085,
6.38722790132095));
#72558=CARTESIAN_POINT('Ctrl Pts',(8.07101774099448,-0.960422206177113,
6.37900579461805));
#72559=CARTESIAN_POINT('Ctrl Pts',(8.04350754585145,-1.16863336237135,6.37078368791515));
#72560=CARTESIAN_POINT('Ctrl Pts',(8.00798706716778,-1.37543836451278,6.36256158121226));
#72561=CARTESIAN_POINT('Ctrl Pts',(7.99240940999671,-1.46613357876682,6.3589557413084));
#72562=CARTESIAN_POINT('Ctrl Pts',(7.9752918045222,-1.55655844534596,6.35534990140455));
#72563=CARTESIAN_POINT('Ctrl Pts',(7.95664491912615,-1.64666001149114,6.35174406150069));
#72564=CARTESIAN_POINT('Ctrl Pts',(7.91412565053497,-1.85211269755876,6.34352190149313));
#72565=CARTESIAN_POINT('Ctrl Pts',(7.86363746031812,-2.05595153774641,6.33529974148558));
#72566=CARTESIAN_POINT('Ctrl Pts',(7.80532772794959,-2.25755323786646,6.32707758147802));
#72567=CARTESIAN_POINT('Ctrl Pts',(7.74702874377128,-2.45911777689289,6.31885693705519));
#72568=CARTESIAN_POINT('Ctrl Pts',(7.68091117691605,-2.65844571550676,6.31063629263237));
#72569=CARTESIAN_POINT('Ctrl Pts',(7.60717260809678,-2.85492775269743,6.30241564820954));
#72570=CARTESIAN_POINT('Ctrl Pts',(7.53344232330819,-3.05138771645695,6.29419592732064));
#72571=CARTESIAN_POINT('Ctrl Pts',(7.45209284949711,-3.2450021408717,6.28597620643174));
#72572=CARTESIAN_POINT('Ctrl Pts',(7.36337065003751,-3.43517979626484,6.27775648554285));
#72573=CARTESIAN_POINT('Ctrl Pts',(7.27464134160532,-3.62537268987063,6.26953610603896));
#72574=CARTESIAN_POINT('Ctrl Pts',(7.17853824946032,-3.81212799559555,6.26131572653507));
#72575=CARTESIAN_POINT('Ctrl Pts',(7.07535517616391,-3.99487630517273,6.25309534703119));
#72576=CARTESIAN_POINT('Ctrl Pts',(6.9721724847201,-4.17762393844794,6.2448749979487));
#72577=CARTESIAN_POINT('Ctrl Pts',(6.86191001197225,-4.35636434954377,6.2366546488662));
#72578=CARTESIAN_POINT('Ctrl Pts',(6.74490680083194,-4.53055402909964,6.22843429978371));
#72579=CARTESIAN_POINT('Ctrl Pts',(6.62787857284226,-4.70478095273569,6.22021219308079));
#72580=CARTESIAN_POINT('Ctrl Pts',(6.50410689170542,-4.87445495589887,6.21199008637787));
#72581=CARTESIAN_POINT('Ctrl Pts',(6.37397391533588,-5.03906182628451,6.20376797967495));
#72582=CARTESIAN_POINT('Ctrl Pts',(6.31690354444877,-5.11125087018064,6.20016213977103));
#72583=CARTESIAN_POINT('Ctrl Pts',(6.25861024672682,-5.18246575875067,6.1965562998671));
#72584=CARTESIAN_POINT('Ctrl Pts',(6.19912872449208,-5.25266509685104,6.19295045996318));
#72585=CARTESIAN_POINT('Ctrl Pts',(6.06349691433436,-5.41273603889675,6.18472829995561));
#72586=CARTESIAN_POINT('Ctrl Pts',(5.92163949572164,-5.56757725726279,6.17650613994804));
#72587=CARTESIAN_POINT('Ctrl Pts',(5.77398408845677,-5.71671193158691,6.16828397994048));
#72588=CARTESIAN_POINT('Ctrl Pts',(5.62635589840466,-5.86581911602604,6.16006333551762));
#72589=CARTESIAN_POINT('Ctrl Pts',(5.47293206030617,-6.00922164620704,6.15184269109476));
#72590=CARTESIAN_POINT('Ctrl Pts',(5.31417758224729,-6.1464790072724,6.14362204667191));
#72591=CARTESIAN_POINT('Ctrl Pts',(5.1554409391846,-6.28372094839786,6.13540232578308));
#72592=CARTESIAN_POINT('Ctrl Pts',(4.99137507492434,-6.41481890572221,6.12718260489425));
#72593=CARTESIAN_POINT('Ctrl Pts',(4.82247927684922,-6.53937162018338,6.11896288400542));
#72594=CARTESIAN_POINT('Ctrl Pts',(4.65356994579412,-6.66393431458135,6.11074250450152));
#72595=CARTESIAN_POINT('Ctrl Pts',(4.47983014357609,-6.78195054084556,6.10252212499762));
#72596=CARTESIAN_POINT('Ctrl Pts',(4.30179028736472,-6.89306085030696,6.09430174549372));
#72597=CARTESIAN_POINT('Ctrl Pts',(4.12375109003059,-7.00417074857923,6.08608139641121));
#72598=CARTESIAN_POINT('Ctrl Pts',(3.94141212233445,-7.10837462717717,6.07786104732871));
#72599=CARTESIAN_POINT('Ctrl Pts',(3.75533113739616,-7.2053574242367,6.0696406982462));
#72600=CARTESIAN_POINT('Ctrl Pts',(3.56921036585876,-7.30236095751314,6.06141859154331));
#72601=CARTESIAN_POINT('Ctrl Pts',(3.37934624043094,-7.39214018827443,6.05319648484041));
#72602=CARTESIAN_POINT('Ctrl Pts',(3.18632035808629,-7.47442640863798,6.04497437813751));
#72603=CARTESIAN_POINT('Ctrl Pts',(3.10166803548755,-7.51051338094985,6.04136853823356));
#72604=CARTESIAN_POINT('Ctrl Pts',(3.01640789291937,-7.54515983824007,6.0377626983296));
#72605=CARTESIAN_POINT('Ctrl Pts',(2.93059020803865,-7.57834603294466,6.03415685842564));
#72606=CARTESIAN_POINT('Ctrl Pts',(2.73490577518451,-7.65401833403713,6.02593469841807));
#72607=CARTESIAN_POINT('Ctrl Pts',(2.53625652373678,-7.72211976588572,6.0177125384105));
#72608=CARTESIAN_POINT('Ctrl Pts',(2.33524608255602,-7.78243620573961,6.00949037840293));
#72609=CARTESIAN_POINT('Ctrl Pts',(2.13427269348219,-7.84274152750846,6.00126973398007));
#72610=CARTESIAN_POINT('Ctrl Pts',(1.93093926589526,-7.89526463656503,5.99304908955722));
#72611=CARTESIAN_POINT('Ctrl Pts',(1.72586489068135,-7.93984117861393,5.98482844513436));
#72612=CARTESIAN_POINT('Ctrl Pts',(1.52081355419142,-7.98441271278875,5.9766087242455));
#72613=CARTESIAN_POINT('Ctrl Pts',(1.31402194883852,-8.02103939958893,5.96838900335665));
#72614=CARTESIAN_POINT('Ctrl Pts',(1.10612048594723,-8.04960775647285,5.96016928246779));
#72615=CARTESIAN_POINT('Ctrl Pts',(0.898202364700916,-8.07817840243076,
5.9519489029639));
#72616=CARTESIAN_POINT('Ctrl Pts',(0.68917450026178,-8.09868938544733,5.94372852346));
#72617=CARTESIAN_POINT('Ctrl Pts',(0.479674636532062,-8.11107883117701,
5.93550814395611));
#72618=CARTESIAN_POINT('Ctrl Pts',(0.270175548104904,-8.1234682310567,5.92728779487363));
#72619=CARTESIAN_POINT('Ctrl Pts',(0.0602047586679581,-8.12773613901279,
5.91906744579115));
#72620=CARTESIAN_POINT('Ctrl Pts',(-0.149597219396503,-8.12387273622924,
5.91084709670866));
#72621=CARTESIAN_POINT('Ctrl Pts',(-0.359444055926759,-8.12000850739857,
5.90262499000573));
#72622=CARTESIAN_POINT('Ctrl Pts',(-0.569121713821754,-8.10800949991264,
5.89440288330279));
#72623=CARTESIAN_POINT('Ctrl Pts',(-0.777990919875223,-8.08791800719392,
5.88618077659986));
#72624=CARTESIAN_POINT('Ctrl Pts',(-0.869591399545033,-8.07910679751351,
5.88257493669595));
#72625=CARTESIAN_POINT('Ctrl Pts',(-0.961036437701934,-8.06873983509607,
5.87896909679204));
#72626=CARTESIAN_POINT('Ctrl Pts',(-1.05227243640895,-8.05682383337714,
5.87536325688813));
#72627=CARTESIAN_POINT('Ctrl Pts',(-1.26031189456843,-8.02965255694936,
5.86714109688057));
#72628=CARTESIAN_POINT('Ctrl Pts',(-1.46733271424759,-7.99441464640026,
5.85891893687301));
#72629=CARTESIAN_POINT('Ctrl Pts',(-1.67270239057271,-7.95121086848238,
5.85069677686544));
#72630=CARTESIAN_POINT('Ctrl Pts',(-1.87803421125648,-7.9080150542851,5.84247613244259));
#72631=CARTESIAN_POINT('Ctrl Pts',(-2.0817152073591,-7.85685636405683,5.83425548801973));
#72632=CARTESIAN_POINT('Ctrl Pts',(-2.28312310706937,-7.79788666501802,
5.82603484359687));
#72633=CARTESIAN_POINT('Ctrl Pts',(-2.4845083799611,-7.73892359082701,5.81781512270794));
#72634=CARTESIAN_POINT('Ctrl Pts',(-2.68362078314228,-7.67215134262059,
5.80959540181902));
#72635=CARTESIAN_POINT('Ctrl Pts',(-2.87985244255038,-7.59777187546695,
5.80137568093009));
#72636=CARTESIAN_POINT('Ctrl Pts',(-3.07609982525436,-7.52338644856975,
5.79315530142622));
#72637=CARTESIAN_POINT('Ctrl Pts',(-3.26946572601762,-7.44139268686743,
5.78493492192234));
#72638=CARTESIAN_POINT('Ctrl Pts',(-3.45936052270696,-7.35204137205692,
5.77671454241847));
#72639=CARTESIAN_POINT('Ctrl Pts',(-3.64925461664817,-7.26269038791092,
5.76849419333595));
#72640=CARTESIAN_POINT('Ctrl Pts',(-3.83567736629031,-7.16598203319751,
5.76027384425343));
#72641=CARTESIAN_POINT('Ctrl Pts',(-4.01806162330063,-7.06221412546085,
5.75205349517091));
#72642=CARTESIAN_POINT('Ctrl Pts',(-4.20048487649988,-6.95842403076024,
5.74383138846802));
#72643=CARTESIAN_POINT('Ctrl Pts',(-4.37886765541288,-6.84757151347801,
5.73560928176513));
#72644=CARTESIAN_POINT('Ctrl Pts',(-4.55266883186641,-6.72999955942437,
5.72738717506223));
#72645=CARTESIAN_POINT('Ctrl Pts',(-4.62889007783673,-6.6784378783587,5.72378133515836));
#72646=CARTESIAN_POINT('Ctrl Pts',(-4.70423050929684,-6.62558441772932,
5.72017549525449));
#72647=CARTESIAN_POINT('Ctrl Pts',(-4.77864627239449,-6.57147071558797,
5.71656965535063));
#72648=CARTESIAN_POINT('Ctrl Pts',(-4.9483316515537,-6.44807879318686,5.70834749534304));
#72649=CARTESIAN_POINT('Ctrl Pts',(-5.11326322577337,-6.31809069393865,
5.70012533533545));
#72650=CARTESIAN_POINT('Ctrl Pts',(-5.27293378566799,-6.18189751245207,
5.69190317532786));
#72651=CARTESIAN_POINT('Ctrl Pts',(-5.43257491360501,-6.04572943535508,
5.68368253090502));
#72652=CARTESIAN_POINT('Ctrl Pts',(-5.58695673828264,-5.90335875028178,
5.67546188648218));
#72653=CARTESIAN_POINT('Ctrl Pts',(-5.73560548418229,-5.75521652870837,
5.66724124205934));
#72654=CARTESIAN_POINT('Ctrl Pts',(-5.88423753039618,-5.60709094991612,
5.65902152117055));
#72655=CARTESIAN_POINT('Ctrl Pts',(-6.02713757470671,-5.45319533735453,
5.65080180028176));
#72656=CARTESIAN_POINT('Ctrl Pts',(-6.16386844811541,-5.29399785765231,
5.64258207939297));
#72657=CARTESIAN_POINT('Ctrl Pts',(-6.30061027725098,-5.13478762205919,
5.63436169988909));
#72658=CARTESIAN_POINT('Ctrl Pts',(-6.43118175342137,-4.97027489262195,
5.6261413203852));
#72659=CARTESIAN_POINT('Ctrl Pts',(-6.55518509520167,-4.80096197966052,
5.61792094088132));
#72660=CARTESIAN_POINT('Ctrl Pts',(-6.6791879780798,-4.63164969327948,5.6097005917988));
#72661=CARTESIAN_POINT('Ctrl Pts',(-6.79662260295266,-4.45753749859879,
5.60148024271627));
#72662=CARTESIAN_POINT('Ctrl Pts',(-6.90713342654288,-4.27915825723167,
5.59325989363375));
#72663=CARTESIAN_POINT('Ctrl Pts',(-7.01766787882271,-4.10074087600106,
5.58503778693083));
#72664=CARTESIAN_POINT('Ctrl Pts',(-7.12127541679716,-3.91805487633051,
5.57681568022792));
#72665=CARTESIAN_POINT('Ctrl Pts',(-7.21764495598233,-3.7316603344735,5.56859357352501));
#72666=CARTESIAN_POINT('Ctrl Pts',(-7.25990822772958,-3.64991621448168,
5.56498773362105));
#72667=CARTESIAN_POINT('Ctrl Pts',(-7.3007800083315,-3.56745915617885,5.56138189371708));
#72668=CARTESIAN_POINT('Ctrl Pts',(-7.34023687728877,-3.48433783491067,
5.55777605381312));
#72669=CARTESIAN_POINT('Ctrl Pts',(-7.42988527438341,-3.29548115639035,
5.54958336706141));
#72670=CARTESIAN_POINT('Ctrl Pts',(-7.5122579616518,-3.10312729128265,5.5413906803097));
#72671=CARTESIAN_POINT('Ctrl Pts',(-7.58709759951355,-2.90785790195389,
5.533197993558));
#72672=CARTESIAN_POINT('Ctrl Pts',(-7.66192252875972,-2.71262688991375,
5.52500691695679));
#72673=CARTESIAN_POINT('Ctrl Pts',(-7.72921725615911,-2.51448177661229,
5.51681584035558));
#72674=CARTESIAN_POINT('Ctrl Pts',(-7.78877289866171,-2.31402339996225,
5.50862476375437));
#72675=CARTESIAN_POINT('Ctrl Pts',(-7.84832856774633,-2.11356493383977,
5.50043368349716));
#72676=CARTESIAN_POINT('Ctrl Pts',(-7.90014505578914,-1.9107934881051,5.49224260323995));
#72677=CARTESIAN_POINT('Ctrl Pts',(-7.94406331021462,-1.70632519931046,
5.48405152298274));
#72678=CARTESIAN_POINT('Ctrl Pts',(-7.98797906389208,-1.5018685531386,5.47586090913359));
#72679=CARTESIAN_POINT('Ctrl Pts',(-8.02399742093537,-1.29571554997155,
5.46767029528444));
#72680=CARTESIAN_POINT('Ctrl Pts',(-8.05201031857506,-1.08849317501803,
5.45947968143529));
#72681=CARTESIAN_POINT('Ctrl Pts',(-8.0800290291043,-0.881227799843871,
5.4512873679714));
#72682=CARTESIAN_POINT('Ctrl Pts',(-8.10003891956644,-0.67289290616256,
5.4430950545075));
#72683=CARTESIAN_POINT('Ctrl Pts',(-8.11198360200186,-0.464122401261746,
5.43490274104361));
#72684=CARTESIAN_POINT('Ctrl Pts',(-8.12082910586603,-0.309519688480521,
5.42883601295827));
#72685=CARTESIAN_POINT('Ctrl Pts',(-8.12525273576271,-0.15467824512713,
5.42276928487294));
#72686=CARTESIAN_POINT('Ctrl Pts',(-8.1252499987303,0.000143642949229983,
5.41670255678761));
#72687=CARTESIAN_POINT('Ctrl Pts',(-8.12573213003729,0.000143651472636081,
5.41670255678761));
#72688=CARTESIAN_POINT('Ctrl Pts',(-8.12585620087823,0.150890634550742,
5.4107958552836));
#72689=CARTESIAN_POINT('Ctrl Pts',(-8.08492819103664,1.65244585104497,5.35195795326709));
#72690=CARTESIAN_POINT('Ctrl Pts',(-7.20076958702257,4.45987723445766,5.24018885073806));
#72691=CARTESIAN_POINT('Ctrl Pts',(-4.18945003805173,7.3613922576165,5.08139524920055));
#72692=CARTESIAN_POINT('Ctrl Pts',(-0.156962385468667,8.46858609222108,
4.92260164766304));
#72693=CARTESIAN_POINT('Ctrl Pts',(3.03083502612948,7.71915799554154,4.79825055164931));
#72694=CARTESIAN_POINT('Ctrl Pts',(4.57224865441187,6.73316530009744,4.7268306561481));
#72695=CARTESIAN_POINT('Ctrl Pts',(4.94648442104396,6.445513583535,4.7083419611594));
#72696=CARTESIAN_POINT('',(-8.12524999734671,0.000207647102394412,5.58329744321239));
#72697=CARTESIAN_POINT('Ctrl Pts',(-8.12533441219635,0.000207649259680899,
5.58329744321239));
#72698=CARTESIAN_POINT('Ctrl Pts',(-8.12562907062817,0.28536548919225,5.57212571550358));
#72699=CARTESIAN_POINT('Ctrl Pts',(-8.04117065934008,1.92141613527934,5.50802278728225));
#72700=CARTESIAN_POINT('Ctrl Pts',(-6.97069019979266,4.81155535844047,5.39098865854841));
#72701=CARTESIAN_POINT('Ctrl Pts',(-3.81915827587035,7.56013339119582,5.2321950570109));
#72702=CARTESIAN_POINT('Ctrl Pts',(0.263284048831229,8.46594757475224,5.07340145547338));
#72703=CARTESIAN_POINT('Ctrl Pts',(3.27676851279123,7.59770512482637,4.95431479619517));
#72704=CARTESIAN_POINT('Ctrl Pts',(4.67912522857444,6.65160043926574,4.88815933742947));
#72705=CARTESIAN_POINT('Ctrl Pts',(4.94671019697112,6.44580737750965,4.87493507917627));
#72706=CARTESIAN_POINT('Ctrl Pts',(4.94675954817621,6.44587135576157,6.8749472715138));
#72707=CARTESIAN_POINT('Ctrl Pts',(5.11324656279799,6.31810411006692,6.86672685106715));
#72708=CARTESIAN_POINT('Ctrl Pts',(5.27477223251341,6.18388990291018,6.85850643062051));
#72709=CARTESIAN_POINT('Ctrl Pts',(5.43084628687882,6.04364096971308,6.85028601017386));
#72710=CARTESIAN_POINT('Ctrl Pts',(5.58695183458293,5.90336373644284,6.84206393097306));
#72711=CARTESIAN_POINT('Ctrl Pts',(5.73760335044615,5.75704954245965,6.83384185177226));
#72712=CARTESIAN_POINT('Ctrl Pts',(5.88234568684138,5.60514913120057,6.82561977257147));
#72713=CARTESIAN_POINT('Ctrl Pts',(5.91455356959241,5.57134844262867,6.823790205843));
#72714=CARTESIAN_POINT('Ctrl Pts',(5.94646900781122,5.53727129789113,6.82196063911454));
#72715=CARTESIAN_POINT('Ctrl Pts',(5.97808724146106,5.50292290478255,6.82013107238607));
#72716=CARTESIAN_POINT('Ctrl Pts',(6.12018108924529,5.34855959037181,6.81190891237851));
#72717=CARTESIAN_POINT('Ctrl Pts',(6.2563163451145,5.18866424262867,6.80368675237095));
#72718=CARTESIAN_POINT('Ctrl Pts',(6.38607265362911,5.02372009820118,6.79546459236338));
#72719=CARTESIAN_POINT('Ctrl Pts',(6.51580504425887,4.85880635780642,6.78724394794052));
#72720=CARTESIAN_POINT('Ctrl Pts',(6.63916065193111,4.68884591001028,6.77902330351766));
#72721=CARTESIAN_POINT('Ctrl Pts',(6.75575976647367,4.51435460948691,6.7708026590948));
#72722=CARTESIAN_POINT('Ctrl Pts',(6.87234578189167,4.33988291188495,6.76258293820593));
#72723=CARTESIAN_POINT('Ctrl Pts',(6.98217665564701,4.16088162306084,6.75436321731706));
#72724=CARTESIAN_POINT('Ctrl Pts',(7.08491586655426,3.97789576614919,6.74614349642818));
#72725=CARTESIAN_POINT('Ctrl Pts',(7.18766330956431,3.79489524727575,6.73792311692429));
#72726=CARTESIAN_POINT('Ctrl Pts',(7.28331780747041,3.60790977841086,6.7297027374204));
#72727=CARTESIAN_POINT('Ctrl Pts',(7.37158817412478,3.41751011024161,6.72148235791651));
#72728=CARTESIAN_POINT('Ctrl Pts',(7.45985821411461,3.2271111466896,6.713262008834));
#72729=CARTESIAN_POINT('Ctrl Pts',(7.54074405579936,3.03329827799834,6.70504165975149));
#72730=CARTESIAN_POINT('Ctrl Pts',(7.61400193618793,2.83666389941184,6.69682131066898));
#72731=CARTESIAN_POINT('Ctrl Pts',(7.68727548008957,2.63998747776947,6.68859920396607));
#72732=CARTESIAN_POINT('Ctrl Pts',(7.75291770129322,2.44048861763195,6.68037709726316));
#72733=CARTESIAN_POINT('Ctrl Pts',(7.81073378077975,2.23877765047939,6.67215499056025));
#72734=CARTESIAN_POINT('Ctrl Pts',(7.83608926861664,2.15031644695909,6.66854915065635));
#72735=CARTESIAN_POINT('Ctrl Pts',(7.85994020024479,2.06142999144596,6.66494331075246));
#72736=CARTESIAN_POINT('Ctrl Pts',(7.88227318895816,1.97217061562417,6.66133747084856));
#72737=CARTESIAN_POINT('Ctrl Pts',(7.93319763694886,1.76863832086244,6.65311531084099));
#72738=CARTESIAN_POINT('Ctrl Pts',(7.97624300383516,1.56309896572517,6.64489315083341));
#72739=CARTESIAN_POINT('Ctrl Pts',(8.01127135890826,1.35617800322678,6.63667099082583));
#72740=CARTESIAN_POINT('Ctrl Pts',(8.04629325723027,1.14929518231821,6.628450346403));
#72741=CARTESIAN_POINT('Ctrl Pts',(8.07330104392661,0.941031553192318,6.62022970198017));
#72742=CARTESIAN_POINT('Ctrl Pts',(8.09220808537406,0.732021765732926,6.61200905755734));
#72743=CARTESIAN_POINT('Ctrl Pts',(8.11111300274323,0.523035459109987,6.60378933666833));
#72744=CARTESIAN_POINT('Ctrl Pts',(8.12191896516244,0.313303455333208,6.59556961577933));
#72745=CARTESIAN_POINT('Ctrl Pts',(8.12459121942834,0.103465355012618,6.58734989489032));
#72746=CARTESIAN_POINT('Ctrl Pts',(8.12726368781179,-0.106389558834649,
6.57912951538642));
#72747=CARTESIAN_POINT('Ctrl Pts',(8.12180113934578,-0.316350291117155,
6.57090913588252));
#72748=CARTESIAN_POINT('Ctrl Pts',(8.10822093952032,-0.52577633878319,6.56268875637863));
#72749=CARTESIAN_POINT('Ctrl Pts',(8.09464078995146,-0.735201611420664,
6.55446840729611));
#72750=CARTESIAN_POINT('Ctrl Pts',(8.07294307087896,-0.944091909047287,
6.54624805821359));
#72751=CARTESIAN_POINT('Ctrl Pts',(8.04319714669472,-1.15181041057196,6.53802770913107));
#72752=CARTESIAN_POINT('Ctrl Pts',(8.01344486243466,-1.35957332508609,6.52980560242814));
#72753=CARTESIAN_POINT('Ctrl Pts',(7.9756409770586,-1.56616365073405,6.52158349572522));
#72754=CARTESIAN_POINT('Ctrl Pts',(7.92990641515993,-1.77095223236128,6.5133613890223));
#72755=CARTESIAN_POINT('Ctrl Pts',(7.90984932830451,-1.8607631368102,6.50975554911854));
#72756=CARTESIAN_POINT('Ctrl Pts',(7.88826759828174,-1.95022764285475,6.50614970921479));
#72757=CARTESIAN_POINT('Ctrl Pts',(7.86517450686964,-2.03929339208167,6.50254386931103));
#72758=CARTESIAN_POINT('Ctrl Pts',(7.81251684659427,-2.24238417283806,6.49432170930347));
#72759=CARTESIAN_POINT('Ctrl Pts',(7.75198012259201,-2.44346782500171,6.48609954929591));
#72760=CARTESIAN_POINT('Ctrl Pts',(7.68374244915463,-2.64192913182,6.47787738928836));
#72761=CARTESIAN_POINT('Ctrl Pts',(7.6155173539177,-2.84035385641074,6.46965674486554));
#72762=CARTESIAN_POINT('Ctrl Pts',(7.53959423830998,-3.03615692144081,6.46143610044273));
#72763=CARTESIAN_POINT('Ctrl Pts',(7.45620066198893,-3.22873957615907,6.45321545601991));
#72764=CARTESIAN_POINT('Ctrl Pts',(7.37281645437288,-3.42130059551691,6.44499573513097));
#72765=CARTESIAN_POINT('Ctrl Pts',(7.2819635787938,-3.61064165611998,6.43677601424204));
#72766=CARTESIAN_POINT('Ctrl Pts',(7.18391752103794,-3.79618448095243,6.4285562933531));
#72767=CARTESIAN_POINT('Ctrl Pts',(7.08586360722461,-3.98174217262531,6.4203359138492));
#72768=CARTESIAN_POINT('Ctrl Pts',(6.98061549508917,-4.16350075819488,6.41211553434531));
#72769=CARTESIAN_POINT('Ctrl Pts',(6.86849486896408,-4.34090610328237,6.40389515484141));
#72770=CARTESIAN_POINT('Ctrl Pts',(6.75637465776682,-4.51831079184111,6.3956748057589));
#72771=CARTESIAN_POINT('Ctrl Pts',(6.63738214339274,-4.69136202407706,6.38745445667638));
#72772=CARTESIAN_POINT('Ctrl Pts',(6.51188291021747,-4.85953377662072,6.37923410759387));
#72773=CARTESIAN_POINT('Ctrl Pts',(6.38635684363019,-5.0277414865309,6.37101200089094));
#72774=CARTESIAN_POINT('Ctrl Pts',(6.25432145540267,-5.19106739585481,6.36278989418801));
#72775=CARTESIAN_POINT('Ctrl Pts',(6.11618393866971,-5.34901688077899,6.35456778748508));
#72776=CARTESIAN_POINT('Ctrl Pts',(6.05560314252433,-5.41828629993294,6.35096194758123));
#72777=CARTESIAN_POINT('Ctrl Pts',(5.99384924426072,-5.48652210404114,6.34735610767737));
#72778=CARTESIAN_POINT('Ctrl Pts',(5.93095895674036,-5.55368467019521,6.34375026777352));
#72779=CARTESIAN_POINT('Ctrl Pts',(5.78755436288664,-5.70683106054015,6.33552810776595));
#72780=CARTESIAN_POINT('Ctrl Pts',(5.63819122501462,-5.85444536596324,6.32730594775838));
#72781=CARTESIAN_POINT('Ctrl Pts',(5.48332028749775,-5.9960725635382,6.31908378775082));
#72782=CARTESIAN_POINT('Ctrl Pts',(5.32847789722709,-6.13767365507582,6.31086314332797));
#72783=CARTESIAN_POINT('Ctrl Pts',(5.16812995130048,-6.27328964232015,6.30264249890511));
#72784=CARTESIAN_POINT('Ctrl Pts',(5.00276273555141,-6.40250361767005,6.29442185448227));
#72785=CARTESIAN_POINT('Ctrl Pts',(4.83741409769366,-6.53170307670136,6.28620213359337));
#72786=CARTESIAN_POINT('Ctrl Pts',(4.66704754823662,-6.65450177806621,6.27798241270448));
#72787=CARTESIAN_POINT('Ctrl Pts',(4.49218166297588,-6.77052372193786,6.26976269181559));
#72788=CARTESIAN_POINT('Ctrl Pts',(4.31730176637635,-6.88655496220691,6.2615423123117));
#72789=CARTESIAN_POINT('Ctrl Pts',(4.1379220580616,-6.99580819456734,6.25332193280781));
#72790=CARTESIAN_POINT('Ctrl Pts',(3.95459013144472,-7.09795072220003,6.24510155330392));
#72791=CARTESIAN_POINT('Ctrl Pts',(3.77125888328944,-7.20009287183102,6.23688120422142));
#72792=CARTESIAN_POINT('Ctrl Pts',(3.58397570521678,-7.29512422805787,6.22866085513891));
#72793=CARTESIAN_POINT('Ctrl Pts',(3.3933132912971,-7.38275778213036,6.22044050605641));
#72794=CARTESIAN_POINT('Ctrl Pts',(3.20261011120727,-7.47041007342695,6.2122183993535));
#72795=CARTESIAN_POINT('Ctrl Pts',(3.00852652003218,-7.55066127925759,6.20399629265059));
#72796=CARTESIAN_POINT('Ctrl Pts',(2.81165672712676,-7.62327187048336,6.19577418594768));
#72797=CARTESIAN_POINT('Ctrl Pts',(2.7253186411861,-7.65511555443778,6.19216834604379));
#72798=CARTESIAN_POINT('Ctrl Pts',(2.63844493492152,-7.68549034782062,6.18856250613991));
#72799=CARTESIAN_POINT('Ctrl Pts',(2.55108680360857,-7.71437902121449,6.18495666623602));
#72800=CARTESIAN_POINT('Ctrl Pts',(2.35188979188242,-7.78025196659809,6.17673450622844));
#72801=CARTESIAN_POINT('Ctrl Pts',(2.1501071362402,-7.83841630277248,6.16851234622086));
#72802=CARTESIAN_POINT('Ctrl Pts',(1.9463523433089,-7.88868811135261,6.16029018621328));
#72803=CARTESIAN_POINT('Ctrl Pts',(1.74263510834874,-7.93895065336723,6.15206954179041));
#72804=CARTESIAN_POINT('Ctrl Pts',(1.53694674804625,-7.98132350075102,6.14384889736755));
#72805=CARTESIAN_POINT('Ctrl Pts',(1.32991374343956,-8.0156732092514,6.13562825294468));
#72806=CARTESIAN_POINT('Ctrl Pts',(1.12290399759584,-8.05001905879348,6.12740853205581));
#72807=CARTESIAN_POINT('Ctrl Pts',(0.914550200080307,-8.07634352063609,
6.11918881116696));
#72808=CARTESIAN_POINT('Ctrl Pts',(0.70548761512801,-8.09456452117104,6.11096909027809));
#72809=CARTESIAN_POINT('Ctrl Pts',(0.496408278784366,-8.11278698168561,
6.1027487107742));
#72810=CARTESIAN_POINT('Ctrl Pts',(0.286620335328576,-8.12290465517997,
6.0945283312703));
#72811=CARTESIAN_POINT('Ctrl Pts',(0.0767638127118421,-8.12488737642301,
6.0863079517664));
#72812=CARTESIAN_POINT('Ctrl Pts',(-0.133091933283915,-8.12687009032854,
6.07808760268386));
#72813=CARTESIAN_POINT('Ctrl Pts',(-0.343015962777012,-8.12071791208522,
6.06986725360131));
#72814=CARTESIAN_POINT('Ctrl Pts',(-0.552368064768117,-8.10645280523635,
6.06164690451877));
#72815=CARTESIAN_POINT('Ctrl Pts',(-0.761764929032563,-8.09218464831727,
6.05342479781588));
#72816=CARTESIAN_POINT('Ctrl Pts',(-0.97058932697103,-8.06980011736266,
6.045202691113));
#72817=CARTESIAN_POINT('Ctrl Pts',(-1.17820487007173,-8.03937316254441,
6.03698058441012));
#72818=CARTESIAN_POINT('Ctrl Pts',(-1.26925555051546,-8.02602929195236,
6.03337474450623));
#72819=CARTESIAN_POINT('Ctrl Pts',(-1.36007381335723,-8.01113929371327,
6.02976890460236));
#72820=CARTESIAN_POINT('Ctrl Pts',(-1.45060645962936,-7.99471253152867,
6.02616306469848));
#72821=CARTESIAN_POINT('Ctrl Pts',(-1.65704210940815,-7.95725566414464,
6.01794090469093));
#72822=CARTESIAN_POINT('Ctrl Pts',(-1.86206025867977,-7.91179261772738,
6.00971874468338));
#72823=CARTESIAN_POINT('Ctrl Pts',(-2.06503417928948,-7.85845540808537,
6.00149658467583));
#72824=CARTESIAN_POINT('Ctrl Pts',(-2.26797068586497,-7.80512803005217,
5.99327594025302));
#72825=CARTESIAN_POINT('Ctrl Pts',(-2.46886343053342,-7.74392946063848,
5.98505529583021));
#72826=CARTESIAN_POINT('Ctrl Pts',(-2.66709844025841,-7.67504224564732,
5.9768346514074));
#72827=CARTESIAN_POINT('Ctrl Pts',(-2.86531117961673,-7.60616276967027,
5.96861493051856));
#72828=CARTESIAN_POINT('Ctrl Pts',(-3.0608665014427,-7.52959646940878,5.96039520962973));
#72829=CARTESIAN_POINT('Ctrl Pts',(-3.25316729715076,-7.4455752027126,5.95217548874089));
#72830=CARTESIAN_POINT('Ctrl Pts',(-3.4454835011922,-7.36154720371101,5.94395510923699));
#72831=CARTESIAN_POINT('Ctrl Pts',(-3.63454438650858,-7.27006316040427,
5.93573472973309));
#72832=CARTESIAN_POINT('Ctrl Pts',(-3.81977349584356,-7.1714027918498,5.92751435022919));
#72833=CARTESIAN_POINT('Ctrl Pts',(-4.0050019196957,-7.07274278841067,5.9192940011467));
#72834=CARTESIAN_POINT('Ctrl Pts',(-4.18639833669129,-6.9669066539555,5.9110736520642));
#72835=CARTESIAN_POINT('Ctrl Pts',(-4.3634110687525,-6.85421997076168,5.9028533029817));
#72836=CARTESIAN_POINT('Ctrl Pts',(-4.54046164849956,-6.74150919365022,
5.8946311962788));
#72837=CARTESIAN_POINT('Ctrl Pts',(-4.71312642176304,-6.62194510006658,
5.8864090895759));
#72838=CARTESIAN_POINT('Ctrl Pts',(-4.88088193900288,-6.49589709432158,
5.878186982873));
#72839=CARTESIAN_POINT('Ctrl Pts',(-4.95445183538576,-6.44061820469394,
5.87458114296899));
#72840=CARTESIAN_POINT('Ctrl Pts',(-5.02707792745737,-6.38409281514049,
5.87097530306498));
#72841=CARTESIAN_POINT('Ctrl Pts',(-5.09871797967501,-6.32635460010255,
5.86736946316097));
#72842=CARTESIAN_POINT('Ctrl Pts',(-5.26207408753466,-6.19469793889987,
5.85914730315339));
#72843=CARTESIAN_POINT('Ctrl Pts',(-5.42035506271293,-6.05668901521307,
5.85092514314583));
#72844=CARTESIAN_POINT('Ctrl Pts',(-5.57307371896767,-5.91274360051675,
5.84270298313825));
#72845=CARTESIAN_POINT('Ctrl Pts',(-5.72576422470408,-5.76882471917357,
5.83448233871543));
#72846=CARTESIAN_POINT('Ctrl Pts',(-5.87289424320319,-5.61897173316621,
5.8262616942926));
#72847=CARTESIAN_POINT('Ctrl Pts',(-6.01401196384205,-5.46363868326454,
5.81804104986978));
#72848=CARTESIAN_POINT('Ctrl Pts',(-6.15511383085854,-5.30832308398143,
5.8098213289808));
#72849=CARTESIAN_POINT('Ctrl Pts',(-6.29020455010105,-5.14752886827035,
5.80160160809184));
#72850=CARTESIAN_POINT('Ctrl Pts',(-6.41887071237704,-4.98174531066054,
5.79338188720287));
#72851=CARTESIAN_POINT('Ctrl Pts',(-6.54754718418195,-4.81594846944647,
5.785161507699));
#72852=CARTESIAN_POINT('Ctrl Pts',(-6.66979788732694,-4.64516171903379,
5.77694112819514));
#72853=CARTESIAN_POINT('Ctrl Pts',(-6.78525044528358,-4.46990648193885,
5.76872074869128));
#72854=CARTESIAN_POINT('Ctrl Pts',(-6.9007025759817,-4.29465189341588,5.76050039960881));
#72855=CARTESIAN_POINT('Ctrl Pts',(-7.00935645168,-4.11492909922792,5.75228005052633));
#72856=CARTESIAN_POINT('Ctrl Pts',(-7.11088339739159,-3.93128794051016,
5.74405970144386));
#72857=CARTESIAN_POINT('Ctrl Pts',(-7.21243205092006,-3.74760751686015,
5.73583759474098));
#72858=CARTESIAN_POINT('Ctrl Pts',(-7.3068505873098,-3.56000731327155,5.72761548803809));
#72859=CARTESIAN_POINT('Ctrl Pts',(-7.39385608552553,-3.36906214680541,
5.7193933813352));
#72860=CARTESIAN_POINT('Ctrl Pts',(-7.43201271723356,-3.28532233101569,
5.71578754143129));
#72861=CARTESIAN_POINT('Ctrl Pts',(-7.46874420789188,-3.20093947430102,
5.71218170152737));
#72862=CARTESIAN_POINT('Ctrl Pts',(-7.50402958019199,-3.11596335378059,
5.70857586162345));
#72863=CARTESIAN_POINT('Ctrl Pts',(-7.58418660423391,-2.92292492194509,
5.70038455239166));
#72864=CARTESIAN_POINT('Ctrl Pts',(-7.65690599965396,-2.72675532862698,
5.69219324315985));
#72865=CARTESIAN_POINT('Ctrl Pts',(-7.72195962781729,-2.52804807487117,
5.68400193392806));
#72866=CARTESIAN_POINT('Ctrl Pts',(-7.78860742395512,-2.3244714118421,5.67560989303508));
#72867=CARTESIAN_POINT('Ctrl Pts',(-7.84720881983712,-2.11823142459329,
5.66721785214211));
#72868=CARTESIAN_POINT('Ctrl Pts',(-7.89757210617641,-1.9099849188526,5.65882581124914));
#72869=CARTESIAN_POINT('Ctrl Pts',(-7.9467185781731,-1.70676980310642,5.65063652828688));
#72870=CARTESIAN_POINT('Ctrl Pts',(-7.98802034313663,-1.50164430971879,
5.64244724532462));
#72871=CARTESIAN_POINT('Ctrl Pts',(-8.02135041567727,-1.29523166708281,
5.63425796236236));
#72872=CARTESIAN_POINT('Ctrl Pts',(-8.05591831390485,-1.0811531884108,5.62576454250403));
#72873=CARTESIAN_POINT('Ctrl Pts',(-8.0819110099373,-0.865690460132721,
5.61727112264571));
#72874=CARTESIAN_POINT('Ctrl Pts',(-8.09924532175734,-0.649548135623411,
5.60877770278738));
#72875=CARTESIAN_POINT('Ctrl Pts',(-8.11657963357738,-0.433405811114101,
5.60028428292905));
#72876=CARTESIAN_POINT('Ctrl Pts',(-8.12525553763274,-0.216584249013234,
5.59179086307072));
#72877=CARTESIAN_POINT('Ctrl Pts',(-8.12524999734671,0.000207647102394412,
5.58329744321239));
#72878=CARTESIAN_POINT('Origin',(0.,0.,24.4167025567876));
#72879=CARTESIAN_POINT('',(4.9467595481762,6.44587135576158,8.87494054454767));
#72880=CARTESIAN_POINT('',(4.94675954817621,6.44587135576157,8.70834331018201));
#72881=CARTESIAN_POINT('',(4.9467595481762,6.44587135576158,24.4167025567876));
#72882=CARTESIAN_POINT('',(-8.12524999753662,-0.000200077936422182,7.41670255682301));
#72883=CARTESIAN_POINT('Ctrl Pts',(4.94675954817621,6.44587135576157,8.708343310182));
#72884=CARTESIAN_POINT('Ctrl Pts',(5.11321786853059,6.31812613092856,8.70012269712016));
#72885=CARTESIAN_POINT('Ctrl Pts',(5.27474386885071,6.18391519945133,8.69190208405833));
#72886=CARTESIAN_POINT('Ctrl Pts',(5.43084219160774,6.04364464974184,8.68368147099649));
#72887=CARTESIAN_POINT('Ctrl Pts',(5.58692326850953,5.90338959722383,8.67546176615391));
#72888=CARTESIAN_POINT('Ctrl Pts',(5.73757764558412,5.75707646023444,8.66724206131133));
#72889=CARTESIAN_POINT('Ctrl Pts',(5.88234461276443,5.60515025839462,8.65902235646874));
#72890=CARTESIAN_POINT('Ctrl Pts',(6.0271233166663,5.45321173941117,8.65080198522837));
#72891=CARTESIAN_POINT('Ctrl Pts',(6.16601345141907,5.2956594581423,8.642581613988));
#72892=CARTESIAN_POINT('Ctrl Pts',(6.29859188485475,5.13297455970141,8.63436124274763));
#72893=CARTESIAN_POINT('Ctrl Pts',(6.43117007521497,4.97028995953456,8.62614088657887));
#72894=CARTESIAN_POINT('Ctrl Pts',(6.55743640308595,4.80247299154491,8.61792053041011));
#72895=CARTESIAN_POINT('Ctrl Pts',(6.67700834462886,4.63003748670101,8.60970017424135));
#72896=CARTESIAN_POINT('Ctrl Pts',(6.79660566708931,4.45756537986442,8.6014780731801));
#72897=CARTESIAN_POINT('Ctrl Pts',(6.90950559627171,4.28047302027635,8.59325597211886));
#72898=CARTESIAN_POINT('Ctrl Pts',(7.01536860951096,4.09930370126297,8.58503387105761));
#72899=CARTESIAN_POINT('Ctrl Pts',(7.05905657855677,4.02453802665272,8.58164074171372));
#72900=CARTESIAN_POINT('Ctrl Pts',(7.10154662717555,3.94907833495743,8.57824761236983));
#72901=CARTESIAN_POINT('Ctrl Pts',(7.14281713462611,3.87296410308586,8.57485448302593));
#72902=CARTESIAN_POINT('Ctrl Pts',(7.24282296448423,3.68852568949356,8.56663232301836));
#72903=CARTESIAN_POINT('Ctrl Pts',(7.33569775733754,3.50018131614254,8.55841016301079));
#72904=CARTESIAN_POINT('Ctrl Pts',(7.42115217109695,3.30850238263825,8.55018800300323));
#72905=CARTESIAN_POINT('Ctrl Pts',(7.50659083310692,3.11685878117127,8.54196735858038));
#72906=CARTESIAN_POINT('Ctrl Pts',(7.58461172583095,2.9218821157531,8.53374671415755));
#72907=CARTESIAN_POINT('Ctrl Pts',(7.65497289788578,2.72416546764954,8.52552606973471));
#72908=CARTESIAN_POINT('Ctrl Pts',(7.72532616533749,2.52647103167784,8.51730634884582));
#72909=CARTESIAN_POINT('Ctrl Pts',(7.78802133116929,2.32603750551014,8.50908662795694));
#72910=CARTESIAN_POINT('Ctrl Pts',(7.84286545707911,2.12347568496917,8.50086690706805));
#72911=CARTESIAN_POINT('Ctrl Pts',(7.89771397744039,1.92089763391905,8.49264652756416));
#72912=CARTESIAN_POINT('Ctrl Pts',(7.94471012115541,1.71619123193746,8.48442614806026));
#72913=CARTESIAN_POINT('Ctrl Pts',(7.98371120191593,1.50998112799536,8.47620576855636));
#72914=CARTESIAN_POINT('Ctrl Pts',(8.02271213834406,1.30377178718071,8.46798541947385));
#72915=CARTESIAN_POINT('Ctrl Pts',(8.05371801877767,1.09605904603583,8.45976507039135));
#72916=CARTESIAN_POINT('Ctrl Pts',(8.0766374345402,0.887476936874398,8.45154472130884));
#72917=CARTESIAN_POINT('Ctrl Pts',(8.09956175077984,0.678850230072898,8.44332261460593));
#72918=CARTESIAN_POINT('Ctrl Pts',(8.11439611591062,0.46935407733536,8.43510050790302));
#72919=CARTESIAN_POINT('Ctrl Pts',(8.12110096613918,0.259627926605015,8.42687840120012));
#72920=CARTESIAN_POINT('Ctrl Pts',(8.12404140675585,0.167651630198292,8.42327256129622));
#72921=CARTESIAN_POINT('Ctrl Pts',(8.12541897333413,0.0756311367006419,
8.41966672139232));
#72922=CARTESIAN_POINT('Ctrl Pts',(8.12523349038375,-0.0163795374249914,
8.41606088148843));
#72923=CARTESIAN_POINT('Ctrl Pts',(8.12481054578905,-0.226185437084521,
8.40783872148086));
#72924=CARTESIAN_POINT('Ctrl Pts',(8.11625692606618,-0.436009567513309,
8.39961656147329));
#72925=CARTESIAN_POINT('Ctrl Pts',(8.09959192648282,-0.645211738078572,
8.39139440146571));
#72926=CARTESIAN_POINT('Ctrl Pts',(8.08292999874661,-0.854375346561104,
8.38317375704287));
#72927=CARTESIAN_POINT('Ctrl Pts',(8.05815969871724,-1.06291692993365,8.37495311262003));
#72928=CARTESIAN_POINT('Ctrl Pts',(8.02535230981967,-1.27019993141711,8.36673246819718));
#72929=CARTESIAN_POINT('Ctrl Pts',(7.99254860661099,-1.47745964605331,8.3585127473083));
#72930=CARTESIAN_POINT('Ctrl Pts',(7.95170966325661,-1.68346076968223,8.35029302641941));
#72931=CARTESIAN_POINT('Ctrl Pts',(7.90295827801188,-1.88757463918743,8.34207330553052));
#72932=CARTESIAN_POINT('Ctrl Pts',(7.85420298650384,-2.09170486356159,8.33385292602663));
#72933=CARTESIAN_POINT('Ctrl Pts',(7.79753405223371,-2.2939472439496,8.32563254652274));
#72934=CARTESIAN_POINT('Ctrl Pts',(7.7331250287989,-2.49368499443374,8.31741216701884));
#72935=CARTESIAN_POINT('Ctrl Pts',(7.66871624372434,-2.69342200574288,8.30919181793633));
#72936=CARTESIAN_POINT('Ctrl Pts',(7.59656751990552,-2.89065412560853,8.30097146885382));
#72937=CARTESIAN_POINT('Ctrl Pts',(7.51690192843684,-3.08478086106007,8.29275111977131));
#72938=CARTESIAN_POINT('Ctrl Pts',(7.43721930340095,-3.27894910339977,8.28452901306841));
#72939=CARTESIAN_POINT('Ctrl Pts',(7.35001671190377,-3.47001036173554,8.2763069063655));
#72940=CARTESIAN_POINT('Ctrl Pts',(7.25556534238605,-3.65738419158643,8.26808479966259));
#72941=CARTESIAN_POINT('Ctrl Pts',(7.21414329211456,-3.73955778249652,8.26447895975869));
#72942=CARTESIAN_POINT('Ctrl Pts',(7.17132769597844,-3.82102245975466,8.26087311985478));
#72943=CARTESIAN_POINT('Ctrl Pts',(7.1271442429179,-3.90173070612801,8.25726727995088));
#72944=CARTESIAN_POINT('Ctrl Pts',(7.02639561557108,-4.08576442179398,8.24904511994331));
#72945=CARTESIAN_POINT('Ctrl Pts',(6.91849850696173,-4.26592419553473,8.24082295993573));
#72946=CARTESIAN_POINT('Ctrl Pts',(6.80377614654044,-4.44165709057637,8.23260079992816));
#72947=CARTESIAN_POINT('Ctrl Pts',(6.68907493280776,-4.61735759290226,8.22438015550532));
#72948=CARTESIAN_POINT('Ctrl Pts',(6.56755113950271,-4.78863259814186,8.21615951108247));
#72949=CARTESIAN_POINT('Ctrl Pts',(6.43957190969968,-4.9549572331461,8.20793886665963));
#72950=CARTESIAN_POINT('Ctrl Pts',(6.31160705749997,-5.12126318269934,8.19971914577075));
#72951=CARTESIAN_POINT('Ctrl Pts',(6.17718839657641,-5.28261963849276,8.19149942488187));
#72952=CARTESIAN_POINT('Ctrl Pts',(6.03672452997019,-5.43853330519877,8.18327970399298));
#72953=CARTESIAN_POINT('Ctrl Pts',(5.89624940852793,-5.59445946467459,8.17505932448909));
#72954=CARTESIAN_POINT('Ctrl Pts',(5.74972830909333,-5.74494174255745,8.1668389449852));
#72955=CARTESIAN_POINT('Ctrl Pts',(5.59760872190857,-5.88952155602754,8.1586185654813));
#72956=CARTESIAN_POINT('Ctrl Pts',(5.44548969767696,-6.03410083444713,8.15039821639879));
#72957=CARTESIAN_POINT('Ctrl Pts',(5.28777244291146,-6.17277749075465,8.14217786731628));
#72958=CARTESIAN_POINT('Ctrl Pts',(5.12494013544889,-6.30513094000157,8.13395751823377));
#72959=CARTESIAN_POINT('Ctrl Pts',(4.96207301226475,-6.4375126881832,8.12573541153087));
#72960=CARTESIAN_POINT('Ctrl Pts',(4.7940888805261,-6.56356834210117,8.11751330482795));
#72961=CARTESIAN_POINT('Ctrl Pts',(4.62150357939489,-6.68291794264603,8.10929119812504));
#72962=CARTESIAN_POINT('Ctrl Pts',(4.54581556072405,-6.73525921814972,8.10568535822116));
#72963=CARTESIAN_POINT('Ctrl Pts',(4.46924299772639,-6.78631126521106,8.10207951831727));
#72964=CARTESIAN_POINT('Ctrl Pts',(4.39183118215686,-6.83604464803549,8.09847367841338));
#72965=CARTESIAN_POINT('Ctrl Pts',(4.21531410123973,-6.94944841586751,8.09025151840582));
#72966=CARTESIAN_POINT('Ctrl Pts',(4.03437315758485,-7.05603033285991,8.08202935839825));
#72967=CARTESIAN_POINT('Ctrl Pts',(3.84955672844517,-7.15545949307118,8.07380719839069));
#72968=CARTESIAN_POINT('Ctrl Pts',(3.66477436638238,-7.25487032557825,8.06558655396785));
#72969=CARTESIAN_POINT('Ctrl Pts',(3.4761182043948,-7.34713089301159,8.05736590954501));
#72970=CARTESIAN_POINT('Ctrl Pts',(3.28416175498827,-7.43195594238639,8.04914526512217));
#72971=CARTESIAN_POINT('Ctrl Pts',(3.09222687059411,-7.51677146223903,8.04092554423329));
#72972=CARTESIAN_POINT('Ctrl Pts',(2.89699270884084,-7.59415301246364,8.03270582334441));
#72973=CARTESIAN_POINT('Ctrl Pts',(2.69905408157299,-7.66386290503974,8.02448610245552));
#72974=CARTESIAN_POINT('Ctrl Pts',(2.50109959423505,-7.73357838320465,8.01626572295164));
#72975=CARTESIAN_POINT('Ctrl Pts',(2.30044048588349,-7.79562087486791,8.00804534344775));
#72976=CARTESIAN_POINT('Ctrl Pts',(2.09768910876352,-7.84980177873779,7.99982496394386));
#72977=CARTESIAN_POINT('Ctrl Pts',(1.89493848197112,-7.90398248209891,7.99160461486136));
#72978=CARTESIAN_POINT('Ctrl Pts',(1.69009588772657,-7.95030158224647,7.98338426577886));
#72979=CARTESIAN_POINT('Ctrl Pts',(1.48378683720432,-7.98862091879688,7.97516391669636));
#72980=CARTESIAN_POINT('Ctrl Pts',(1.27743367505221,-8.02694844853313,7.96694180999345));
#72981=CARTESIAN_POINT('Ctrl Pts',(1.06961372045437,-8.05727274360453,7.95871970329055));
#72982=CARTESIAN_POINT('Ctrl Pts',(0.860961728771738,-8.07950694436798,
7.95049759658764));
#72983=CARTESIAN_POINT('Ctrl Pts',(0.769456509388262,-8.08925784778504,
7.94689175668371));
#72984=CARTESIAN_POINT('Ctrl Pts',(0.677791352711616,-8.0974534542192,7.94328591677978));
#72985=CARTESIAN_POINT('Ctrl Pts',(0.586020113558015,-8.10408958421644,
7.93968007687586));
#72986=CARTESIAN_POINT('Ctrl Pts',(0.376760181747902,-8.11922151578361,
7.93145791686828));
#72987=CARTESIAN_POINT('Ctrl Pts',(0.166879311345257,-8.12624649689666,
7.92323575686071));
#72988=CARTESIAN_POINT('Ctrl Pts',(-0.0429826381961779,-8.12513630995282,
7.91501359685313));
#72989=CARTESIAN_POINT('Ctrl Pts',(-0.252805904038364,-8.12402632764892,
7.90679295243028));
#72990=CARTESIAN_POINT('Ctrl Pts',(-0.462609960989967,-8.11478417174254,
7.89857230800743));
#72991=CARTESIAN_POINT('Ctrl Pts',(-0.671754719371072,-8.09743373912394,
7.89035166358458));
#72992=CARTESIAN_POINT('Ctrl Pts',(-0.88087598174945,-8.0800852557094,7.88213194269567));
#72993=CARTESIAN_POINT('Ctrl Pts',(-1.08933779941136,-8.05463033854202,
7.87391222180677));
#72994=CARTESIAN_POINT('Ctrl Pts',(-1.29650413562753,-8.02114484277654,
7.86569250091787));
#72995=CARTESIAN_POINT('Ctrl Pts',(-1.50368707129472,-7.98765666394558,
7.85747212141397));
#72996=CARTESIAN_POINT('Ctrl Pts',(-1.70957402630208,-7.9461366652205,7.84925174191007));
#72997=CARTESIAN_POINT('Ctrl Pts',(-1.91353704574931,-7.89671219793687,
7.84103136240618));
#72998=CARTESIAN_POINT('Ctrl Pts',(-2.11749931038528,-7.84728791355966,
7.83281101332366));
#72999=CARTESIAN_POINT('Ctrl Pts',(-2.31953736748993,-7.78995929124146,
7.82459066424115));
#73000=CARTESIAN_POINT('Ctrl Pts',(-2.51903583935572,-7.72490427141602,
7.81637031515863));
#73001=CARTESIAN_POINT('Ctrl Pts',(-2.71857696665826,-7.6598353419588,7.80814820845572));
#73002=CARTESIAN_POINT('Ctrl Pts',(-2.91557714326042,-7.58703680612623,
7.79992610175281));
#73003=CARTESIAN_POINT('Ctrl Pts',(-3.10943741765436,-7.50673607556513,
7.7917039950499));
#73004=CARTESIAN_POINT('Ctrl Pts',(-3.19445566643648,-7.47151984826135,
7.78809815514605));
#73005=CARTESIAN_POINT('Ctrl Pts',(-3.2788702611578,-7.43486135523398,7.78449231524221));
#73006=CARTESIAN_POINT('Ctrl Pts',(-3.3626319109193,-7.39678269210115,7.78088647533836));
#73007=CARTESIAN_POINT('Ctrl Pts',(-3.55362810187657,-7.30995441644249,
7.77266431533079));
#73008=CARTESIAN_POINT('Ctrl Pts',(-3.74129095503225,-7.21571013987357,
7.76444215532323));
#73009=CARTESIAN_POINT('Ctrl Pts',(-3.9250450928939,-7.11433121110126,7.75621999531566));
#73010=CARTESIAN_POINT('Ctrl Pts',(-4.10876535949,-7.01297096943259,7.74799935089282));
#73011=CARTESIAN_POINT('Ctrl Pts',(-4.2885780904998,-6.90447884287115,7.73977870646998));
#73012=CARTESIAN_POINT('Ctrl Pts',(-4.46393263934849,-6.78918205337426,
7.73155806204714));
#73013=CARTESIAN_POINT('Ctrl Pts',(-4.63926748829637,-6.67389821669402,
7.72333834115826));
#73014=CARTESIAN_POINT('Ctrl Pts',(-4.81014490847376,-6.55181140534979,
7.71511862026937));
#73015=CARTESIAN_POINT('Ctrl Pts',(-4.97604267064916,-6.42329252816488,
7.70689889938048));
#73016=CARTESIAN_POINT('Ctrl Pts',(-5.141953725582,-6.29476335325058,7.69867851987659));
#73017=CARTESIAN_POINT('Ctrl Pts',(-5.3028840902678,-6.15980126131947,7.6904581403727));
#73018=CARTESIAN_POINT('Ctrl Pts',(-5.45834326960779,-6.0188185147608,7.6822377608688));
#73019=CARTESIAN_POINT('Ctrl Pts',(-5.61380187363556,-5.87783628994099,
7.6740174117863));
#73020=CARTESIAN_POINT('Ctrl Pts',(-5.76378911598376,-5.73083365531125,
7.6657970627038));
#73021=CARTESIAN_POINT('Ctrl Pts',(-5.90784974920863,-5.57826127958126,
7.6575767136213));
#73022=CARTESIAN_POINT('Ctrl Pts',(-6.05194118452063,-5.42565628183991,
7.64935460691839));
#73023=CARTESIAN_POINT('Ctrl Pts',(-6.1901032764461,-5.26747937848341,7.64113250021548));
#73024=CARTESIAN_POINT('Ctrl Pts',(-6.32191887028163,-5.104216821421,7.63291039351257));
#73025=CARTESIAN_POINT('Ctrl Pts',(-6.37972716022301,-5.03261733185672,
7.62930455360866));
#73026=CARTESIAN_POINT('Ctrl Pts',(-6.43631534393656,-4.96004015653743,
7.62569871370474));
#73027=CARTESIAN_POINT('Ctrl Pts',(-6.4916507089754,-4.88652828040104,7.62209287380082));
#73028=CARTESIAN_POINT('Ctrl Pts',(-6.61782830907694,-4.71890397534152,
7.61387071379325));
#73029=CARTESIAN_POINT('Ctrl Pts',(-6.73753078784233,-4.54636225082834,
7.60564855378568));
#73030=CARTESIAN_POINT('Ctrl Pts',(-6.85038749658374,-4.36942544382544,
7.59742639377811));
#73031=CARTESIAN_POINT('Ctrl Pts',(-6.96322340253104,-4.19252125145402,
7.58920574935524));
#73032=CARTESIAN_POINT('Ctrl Pts',(-7.06921589834827,-4.0112238422345,7.58098510493238));
#73033=CARTESIAN_POINT('Ctrl Pts',(-7.16803799930891,-3.82608400364701,
7.57276446050952));
#73034=CARTESIAN_POINT('Ctrl Pts',(-7.26684899827252,-3.64096496427262,
7.56454473962066));
#73035=CARTESIAN_POINT('Ctrl Pts',(-7.35849107166973,-3.45200461760183,
7.55632501873179));
#73036=CARTESIAN_POINT('Ctrl Pts',(-7.44268308985259,-3.25977851801656,
7.54810529784292));
#73037=CARTESIAN_POINT('Ctrl Pts',(-7.52688185402229,-3.0675370160836,7.53988491833902));
#73038=CARTESIAN_POINT('Ctrl Pts',(-7.60362924930881,-2.87202950765201,
7.53166453883512));
#73039=CARTESIAN_POINT('Ctrl Pts',(-7.67269179738429,-2.67385267822515,
7.52344415933122));
#73040=CARTESIAN_POINT('Ctrl Pts',(-7.74175408987807,-2.47567658219683,
7.51522381024871));
#73041=CARTESIAN_POINT('Ctrl Pts',(-7.80313149744535,-2.2748314645172,7.5070034611662));
#73042=CARTESIAN_POINT('Ctrl Pts',(-7.85663986834665,-2.07193087278654,
7.49878311208368));
#73043=CARTESIAN_POINT('Ctrl Pts',(-7.91015968005217,-1.86898689819991,
7.49056100538076));
#73044=CARTESIAN_POINT('Ctrl Pts',(-7.95580701849676,-1.66398685699576,
7.48233889867785));
#73045=CARTESIAN_POINT('Ctrl Pts',(-7.99344820621045,-1.45755731864338,
7.47411679197493));
#73046=CARTESIAN_POINT('Ctrl Pts',(-8.00995590935653,-1.36702676563262,
7.47051095207106));
#73047=CARTESIAN_POINT('Ctrl Pts',(-8.02492445198856,-1.27622141532451,
7.46690511216719));
#73048=CARTESIAN_POINT('Ctrl Pts',(-8.03834567369,-1.18519466450424,7.46329927226332));
#73049=CARTESIAN_POINT('Ctrl Pts',(-8.07024341346567,-0.968854626698262,
7.45472940094421));
#73050=CARTESIAN_POINT('Ctrl Pts',(-8.09340493463014,-0.751214168910868,
7.44615952962511));
#73051=CARTESIAN_POINT('Ctrl Pts',(-8.1077516028081,-0.532964829667744,
7.43758965830601));
#73052=CARTESIAN_POINT('Ctrl Pts',(-8.11940717704868,-0.355653878793876,
7.430627291145));
#73053=CARTESIAN_POINT('Ctrl Pts',(-8.12524562079903,-0.177941250951312,
7.423664923984));
#73054=CARTESIAN_POINT('Ctrl Pts',(-8.12524999753662,-0.000200077936449244,
7.41670255682299));
#73055=CARTESIAN_POINT('Ctrl Pts',(-8.12524999753664,-0.000200077032885864,
7.41670255678761));
#73056=CARTESIAN_POINT('Ctrl Pts',(-8.12525515579502,0.209279933090809,
7.40849693555404));
#73057=CARTESIAN_POINT('Ctrl Pts',(-8.11715495148673,0.418776541723859,
7.40029131432047));
#73058=CARTESIAN_POINT('Ctrl Pts',(-8.10097160197948,0.627651707893815,
7.3920856930869));
#73059=CARTESIAN_POINT('Ctrl Pts',(-8.08478712724863,0.836541397093457,
7.38387950131887));
#73060=CARTESIAN_POINT('Ctrl Pts',(-8.06051840414201,1.04480926092786,7.37567330955084));
#73061=CARTESIAN_POINT('Ctrl Pts',(-8.02823964397931,1.25182098613935,7.36746711778281));
#73062=CARTESIAN_POINT('Ctrl Pts',(-7.99596128150152,1.45883016089853,7.35926102711775));
#73063=CARTESIAN_POINT('Ctrl Pts',(-7.95567312746925,1.6645829346883,7.35105493645269));
#73064=CARTESIAN_POINT('Ctrl Pts',(-7.90750085760631,1.86845330406072,7.34284884578763));
#73065=CARTESIAN_POINT('Ctrl Pts',(-7.85931743671705,2.07237086580882,7.33464085555808));
#73066=CARTESIAN_POINT('Ctrl Pts',(-7.80324632174305,2.27440486314619,7.32643286532853));
#73067=CARTESIAN_POINT('Ctrl Pts',(-7.73946386678466,2.47394151451377,7.31822487509899));
#73068=CARTESIAN_POINT('Ctrl Pts',(-7.7039275779358,2.58511302842863,7.31365180697459));
#73069=CARTESIAN_POINT('Ctrl Pts',(-7.6659984760938,2.69550958120614,7.3090787388502));
#73070=CARTESIAN_POINT('Ctrl Pts',(-7.62571372598687,2.80502722478685,7.30450567072581));
#73071=CARTESIAN_POINT('Ctrl Pts',(-7.55328365229577,3.00193476359422,7.29628351071824));
#73072=CARTESIAN_POINT('Ctrl Pts',(-7.4732108712274,3.19606791339749,7.28806135071066));
#73073=CARTESIAN_POINT('Ctrl Pts',(-7.38573330237192,3.38683202251519,7.27983919070309));
#73074=CARTESIAN_POINT('Ctrl Pts',(-7.29827185819268,3.57756096822429,7.27161854628026));
#73075=CARTESIAN_POINT('Ctrl Pts',(-7.2034084733784,3.76492184455805,7.26339790185742));
#73076=CARTESIAN_POINT('Ctrl Pts',(-7.10142864793773,3.94834126194145,7.25517725743459));
#73077=CARTESIAN_POINT('Ctrl Pts',(-6.99946027924215,4.13174007339124,7.24695753654567));
#73078=CARTESIAN_POINT('Ctrl Pts',(-6.89037720939769,4.31119805205013,7.23873781565676));
#73079=CARTESIAN_POINT('Ctrl Pts',(-6.7745106117521,4.48616690881627,7.23051809476784));
#73080=CARTESIAN_POINT('Ctrl Pts',(-6.65863473015665,4.66114978517155,7.22229771526395));
#73081=CARTESIAN_POINT('Ctrl Pts',(-6.5359743954019,4.83164257333042,7.21407733576005));
#73082=CARTESIAN_POINT('Ctrl Pts',(-6.40690437318145,4.99712556530336,7.20585695625616));
#73083=CARTESIAN_POINT('Ctrl Pts',(-6.27783482861379,5.16260794486907,7.19763660717364));
#73084=CARTESIAN_POINT('Ctrl Pts',(-6.14235582765208,5.323080334251,7.18941625809111));
#73085=CARTESIAN_POINT('Ctrl Pts',(-6.00088304967101,5.47805532891656,7.18119590900859));
#73086=CARTESIAN_POINT('Ctrl Pts',(-5.85938002292125,5.633063459305,7.17297380230569));
#73087=CARTESIAN_POINT('Ctrl Pts',(-5.71188085789198,5.78257162870153,7.16475169560278));
#73088=CARTESIAN_POINT('Ctrl Pts',(-5.55883954320356,5.92612778257577,7.15652958889988));
#73089=CARTESIAN_POINT('Ctrl Pts',(-5.49172262300483,5.98908494511211,7.15292374899601));
#73090=CARTESIAN_POINT('Ctrl Pts',(-5.42354025621363,6.05089783836143,7.14931790909214));
#73091=CARTESIAN_POINT('Ctrl Pts',(-5.35433288438774,6.11153065325406,7.14571206918827));
#73092=CARTESIAN_POINT('Ctrl Pts',(-5.19652385791237,6.24978768047856,7.1374899091807));
#73093=CARTESIAN_POINT('Ctrl Pts',(-5.03333091776804,6.38195195101942,7.12926774917313));
#73094=CARTESIAN_POINT('Ctrl Pts',(-4.8652474860031,6.50761511326849,7.12104558916556));
#73095=CARTESIAN_POINT('Ctrl Pts',(-4.6971950369337,6.63325511211915,7.1128249447427));
#73096=CARTESIAN_POINT('Ctrl Pts',(-4.52425413169958,6.75239621777111,7.10460430031985));
#73097=CARTESIAN_POINT('Ctrl Pts',(-4.34694980155426,6.86467151328214,7.096383655897));
#73098=CARTESIAN_POINT('Ctrl Pts',(-4.16966539035582,6.97693419542019,7.08816393500816));
#73099=CARTESIAN_POINT('Ctrl Pts',(-3.98801878215426,7.08233244948104,7.07994421411932));
#73100=CARTESIAN_POINT('Ctrl Pts',(-3.80256310636589,7.18054325135675,7.07172449323048));
#73101=CARTESIAN_POINT('Ctrl Pts',(-3.61709257071779,7.27876192249143,7.06350411372658));
#73102=CARTESIAN_POINT('Ctrl Pts',(-3.42781261720923,7.3697918501861,7.05528373422269));
#73103=CARTESIAN_POINT('Ctrl Pts',(-3.23530098080577,7.45335596400019,7.0470633547188));
#73104=CARTESIAN_POINT('Ctrl Pts',(-3.04279005683416,7.53691976856681,7.03884300563624));
#73105=CARTESIAN_POINT('Ctrl Pts',(-2.84704774569189,7.61301769944957,7.03062265655368));
#73106=CARTESIAN_POINT('Ctrl Pts',(-2.6486722548104,7.68142062701279,7.02240230747112));
#73107=CARTESIAN_POINT('Ctrl Pts',(-2.45025434860111,7.74983818003494,7.0141802007682));
#73108=CARTESIAN_POINT('Ctrl Pts',(-2.2492024169488,7.81055734652839,7.00595809406528));
#73109=CARTESIAN_POINT('Ctrl Pts',(-2.04613139517198,7.86339836687622,6.99773598736236));
#73110=CARTESIAN_POINT('Ctrl Pts',(-1.95707373390586,7.88657202134409,6.99413014745849));
#73111=CARTESIAN_POINT('Ctrl Pts',(-1.86762792765624,7.90823112237467,6.99052430755463));
#73112=CARTESIAN_POINT('Ctrl Pts',(-1.77784662131366,7.92836357349886,6.98691846765076));
#73113=CARTESIAN_POINT('Ctrl Pts',(-1.57312420264919,7.97427028009167,6.97869630764319));
#73114=CARTESIAN_POINT('Ctrl Pts',(-1.36658897968878,8.01225095672081,6.97047414763563));
#73115=CARTESIAN_POINT('Ctrl Pts',(-1.15886960653281,8.04218308654774,6.96225198762806));
#73116=CARTESIAN_POINT('Ctrl Pts',(-0.951188522136813,8.07210969900709,
6.95403134320523));
#73117=CARTESIAN_POINT('Ctrl Pts',(-0.742324015167708,8.09399068361679,
6.9458106987824));
#73118=CARTESIAN_POINT('Ctrl Pts',(-0.532912673052062,8.10775503116618,
6.93759005435956));
#73119=CARTESIAN_POINT('Ctrl Pts',(-0.323524856888564,8.12151783238394,
6.9293703334707));
#73120=CARTESIAN_POINT('Ctrl Pts',(-0.113590622617442,8.12716579763455,
6.92115061258183));
#73121=CARTESIAN_POINT('Ctrl Pts',(0.0962497682060561,8.12467990413286,
6.91293089169297));
#73122=CARTESIAN_POINT('Ctrl Pts',(0.306106972743071,8.12219381144596,6.90471051218908));
#73123=CARTESIAN_POINT('Ctrl Pts',(0.51587002364315,8.11157255854095,6.89649013268521));
#73124=CARTESIAN_POINT('Ctrl Pts',(0.724899038140248,8.09284924776208,6.88826975318133));
#73125=CARTESIAN_POINT('Ctrl Pts',(0.933927279078422,8.07412600627305,6.88004940409881));
#73126=CARTESIAN_POINT('Ctrl Pts',(1.14222119531879,8.04730079587844,6.87182905501629));
#73127=CARTESIAN_POINT('Ctrl Pts',(1.34914586295771,8.01245861162253,6.86360870593378));
#73128=CARTESIAN_POINT('Ctrl Pts',(1.55611477385339,7.97760897764243,6.85538659923087));
#73129=CARTESIAN_POINT('Ctrl Pts',(1.7617135601569,7.934738994307,6.84716449252797));
#73130=CARTESIAN_POINT('Ctrl Pts',(1.96531622881724,7.88398501287563,6.83894238582506));
#73131=CARTESIAN_POINT('Ctrl Pts',(2.05460704608971,7.86172663821062,6.83533654592113));
#73132=CARTESIAN_POINT('Ctrl Pts',(2.14351409735526,7.83795259461911,6.83173070601718));
#73133=CARTESIAN_POINT('Ctrl Pts',(2.23198536645265,7.81267744671705,6.82812486611325));
#73134=CARTESIAN_POINT('Ctrl Pts',(2.43371860631164,7.75504475390934,6.81990278708515));
#73135=CARTESIAN_POINT('Ctrl Pts',(2.63325171788618,7.68958486235625,6.81168070805706));
#73136=CARTESIAN_POINT('Ctrl Pts',(2.82997406587421,7.61649094721312,6.80345862902897));
#73137=CARTESIAN_POINT('Ctrl Pts',(3.02667271421202,7.54340583788306,6.79523754053601));
#73138=CARTESIAN_POINT('Ctrl Pts',(3.22056099735752,7.46268864090862,6.78701645204305));
#73139=CARTESIAN_POINT('Ctrl Pts',(3.41104584256796,7.37458160320976,6.77879536355009));
#73140=CARTESIAN_POINT('Ctrl Pts',(3.60150474063423,7.28648656712714,6.77057539490353));
#73141=CARTESIAN_POINT('Ctrl Pts',(3.78856085885258,7.19100382461239,6.76235542625698));
#73142=CARTESIAN_POINT('Ctrl Pts',(3.97164281543318,7.08842301990492,6.75413545761042));
#73143=CARTESIAN_POINT('Ctrl Pts',(4.15473889057928,6.9858343045664,6.74591485507198));
#73144=CARTESIAN_POINT('Ctrl Pts',(4.33385993290286,6.87614657530239,6.73769425253354));
#73145=CARTESIAN_POINT('Ctrl Pts',(4.50845983964032,6.75969506981272,6.7294736499951));
#73146=CARTESIAN_POINT('Ctrl Pts',(4.65798384865252,6.65996823557962,6.72243368376022));
#73147=CARTESIAN_POINT('Ctrl Pts',(4.80419244001679,6.55528173096446,6.71539371752536));
#73148=CARTESIAN_POINT('Ctrl Pts',(4.9467595481762,6.44587135576158,6.70835375129049));
#73149=CARTESIAN_POINT('',(-8.1252499974825,-0.000202263843970515,7.5832974431918));
#73150=CARTESIAN_POINT('Ctrl Pts',(-8.1252499974825,-0.000202263844008403,
7.5832974431918));
#73151=CARTESIAN_POINT('Ctrl Pts',(-8.1252552002741,0.208801884231222,7.57510884366752));
#73152=CARTESIAN_POINT('Ctrl Pts',(-8.11719180360737,0.417835476072454,
7.56692024414324));
#73153=CARTESIAN_POINT('Ctrl Pts',(-8.10107906878029,0.626263110736931,
7.55873164461896));
#73154=CARTESIAN_POINT('Ctrl Pts',(-8.08496842127045,0.83466374473374,7.55054410588326));
#73155=CARTESIAN_POINT('Ctrl Pts',(-8.06081054017175,1.04245827946469,7.54235656714756));
#73156=CARTESIAN_POINT('Ctrl Pts',(-8.02867667051253,1.24901500506112,7.53416902841186));
#73157=CARTESIAN_POINT('Ctrl Pts',(-7.99654068670408,1.45558532042276,7.5259809510022));
#73158=CARTESIAN_POINT('Ctrl Pts',(-7.95642770943993,1.6609173673095,7.51779287359254));
#73159=CARTESIAN_POINT('Ctrl Pts',(-7.90846052257459,1.86438722517056,7.50960479618288));
#73160=CARTESIAN_POINT('Ctrl Pts',(-7.86049297173956,2.06785862693837,7.501416656643));
#73161=CARTESIAN_POINT('Ctrl Pts',(-7.80467116400753,2.26946752036822,7.49322851710311));
#73162=CARTESIAN_POINT('Ctrl Pts',(-7.74116853449045,2.46860229342738,7.48504037756323));
#73163=CARTESIAN_POINT('Ctrl Pts',(-7.67765237376068,2.66777949835102,7.47685049328523));
#73164=CARTESIAN_POINT('Ctrl Pts',(-7.60645221399996,2.86448124447907,7.46866060900724));
#73165=CARTESIAN_POINT('Ctrl Pts',(-7.52779101068967,3.05811217287395,7.46047072472924));
#73166=CARTESIAN_POINT('Ctrl Pts',(-7.51125416811851,3.09881895137494,7.45874897599821));
#73167=CARTESIAN_POINT('Ctrl Pts',(-7.49438774727284,3.13939007887198,7.45702722726718));
#73168=CARTESIAN_POINT('Ctrl Pts',(-7.47719409066218,3.1798201353326,7.45530547853615));
#73169=CARTESIAN_POINT('Ctrl Pts',(-7.39508629338615,3.37289267102977,7.44708331852857));
#73170=CARTESIAN_POINT('Ctrl Pts',(-7.30548280958889,3.56281514419167,7.438861158521));
#73171=CARTESIAN_POINT('Ctrl Pts',(-7.20865076152545,3.74900543622686,7.43063899851343));
#73172=CARTESIAN_POINT('Ctrl Pts',(-7.11183656244216,3.93516140794255,7.42241835409057));
#73173=CARTESIAN_POINT('Ctrl Pts',(-7.00779659456183,4.11758630986869,7.41419770966771));
#73174=CARTESIAN_POINT('Ctrl Pts',(-6.89684444736205,4.29572161940124,7.40597706524484));
#73175=CARTESIAN_POINT('Ctrl Pts',(-6.78590476488787,4.47383691663291,7.39775734435595));
#73176=CARTESIAN_POINT('Ctrl Pts',(-6.66805460937235,4.6476633331402,7.38953762346704));
#73177=CARTESIAN_POINT('Ctrl Pts',(-6.54365194239556,4.81666968135482,7.38131790257815));
#73178=CARTESIAN_POINT('Ctrl Pts',(-6.41923930750566,4.98568957140608,7.37309752307425));
#73179=CARTESIAN_POINT('Ctrl Pts',(-6.28827328486527,5.14988838215142,7.36487714357034));
#73180=CARTESIAN_POINT('Ctrl Pts',(-6.15115395708075,5.30876563419311,7.35665676406644));
#73181=CARTESIAN_POINT('Ctrl Pts',(-6.01403513673758,5.4676422982733,7.34843641498392));
#73182=CARTESIAN_POINT('Ctrl Pts',(-5.87076325166009,5.62119722135228,7.34021606590141));
#73183=CARTESIAN_POINT('Ctrl Pts',(-5.72177764548016,5.76896421710028,7.33199571681889));
#73184=CARTESIAN_POINT('Ctrl Pts',(-5.57276018418834,5.91676280740499,7.32377361011599));
#73185=CARTESIAN_POINT('Ctrl Pts',(-5.41802677073111,6.05877079014034,7.31555150341308));
#73186=CARTESIAN_POINT('Ctrl Pts',(-5.25805325742347,6.19455918565627,7.30732939671017));
#73187=CARTESIAN_POINT('Ctrl Pts',(-5.18789619200383,6.25410976468943,7.30372355680632));
#73188=CARTESIAN_POINT('Ctrl Pts',(-5.11673174874588,6.31246463534114,7.30011771690248));
#73189=CARTESIAN_POINT('Ctrl Pts',(-5.04460209560563,6.3695900385748,7.29651187699863));
#73190=CARTESIAN_POINT('Ctrl Pts',(-4.88012958289725,6.49984934525757,7.28828971699106));
#73191=CARTESIAN_POINT('Ctrl Pts',(-4.71058199250573,6.62375634551582,7.28006755698349));
#73192=CARTESIAN_POINT('Ctrl Pts',(-4.53647239391172,6.74092766477856,7.27184539697592));
#73193=CARTESIAN_POINT('Ctrl Pts',(-4.36239488881203,6.85807738593814,7.26362475255306));
#73194=CARTESIAN_POINT('Ctrl Pts',(-4.1837572985887,6.96849373943008,7.25540410813019));
#73195=CARTESIAN_POINT('Ctrl Pts',(-4.00110220780467,7.07183630220614,7.24718346370733));
#73196=CARTESIAN_POINT('Ctrl Pts',(-3.8184676370875,7.17516725514264,7.2389637428184));
#73197=CARTESIAN_POINT('Ctrl Pts',(-3.63181672365398,7.27142585863154,7.23074402192947));
#73198=CARTESIAN_POINT('Ctrl Pts',(-3.4417179385002,7.36031692213766,7.22252430104054));
#73199=CARTESIAN_POINT('Ctrl Pts',(-3.25160392145396,7.44921510814652,7.21430392153664));
#73200=CARTESIAN_POINT('Ctrl Pts',(-3.05804174689303,7.53074444713321,7.20608354203274));
#73201=CARTESIAN_POINT('Ctrl Pts',(-2.86162218171216,7.6046568661336,7.19786316252884));
#73202=CARTESIAN_POINT('Ctrl Pts',(-2.66520334342744,7.67856901160394,7.18964281344636));
#73203=CARTESIAN_POINT('Ctrl Pts',(-2.46592741284939,7.74486419202678,7.18142246436389));
#73204=CARTESIAN_POINT('Ctrl Pts',(-2.26440322621074,7.80334323169412,7.17320211528141));
#73205=CARTESIAN_POINT('Ctrl Pts',(-2.0628359510097,7.8618347749611,7.16498000857852));
#73206=CARTESIAN_POINT('Ctrl Pts',(-1.8590197428969,7.91250675647965,7.15675790187563));
#73207=CARTESIAN_POINT('Ctrl Pts',(-1.65357769658261,7.9552101395164,7.14853579517274));
#73208=CARTESIAN_POINT('Ctrl Pts',(-1.56348021240926,7.97393788997609,7.14492995526886));
#73209=CARTESIAN_POINT('Ctrl Pts',(-1.47307018490379,7.99113369875667,7.14132411536497));
#73210=CARTESIAN_POINT('Ctrl Pts',(-1.38240079415703,8.00678809553581,7.13771827546109));
#73211=CARTESIAN_POINT('Ctrl Pts',(-1.1756533349293,8.0424837887921,7.12949611545351));
#73212=CARTESIAN_POINT('Ctrl Pts',(-0.967488444512142,8.07017329074264,
7.12127395544593));
#73213=CARTESIAN_POINT('Ctrl Pts',(-0.758540080192574,8.08976541744205,
7.11305179543835));
#73214=CARTESIAN_POINT('Ctrl Pts',(-0.54963023117222,8.10935393273908,7.10483115101552));
#73215=CARTESIAN_POINT('Ctrl Pts',(-0.339937490192298,8.12084802423565,
7.09661050659268));
#73216=CARTESIAN_POINT('Ctrl Pts',(-0.130101183253439,8.1242083457169,7.08838986216984));
#73217=CARTESIAN_POINT('Ctrl Pts',(0.079711549991263,8.12756828968869,7.08017014128097));
#73218=CARTESIAN_POINT('Ctrl Pts',(0.289667522005959,8.12279628320706,7.07195042039211));
#73219=CARTESIAN_POINT('Ctrl Pts',(0.499126315780342,8.10990508473407,7.06373069950324));
#73220=CARTESIAN_POINT('Ctrl Pts',(0.708601892691915,8.09701285333834,7.05551031999937));
#73221=CARTESIAN_POINT('Ctrl Pts',(0.917579917001217,8.07600014547325,7.0472899404955));
#73222=CARTESIAN_POINT('Ctrl Pts',(1.12542293549719,8.04693176178081,7.03906956099163));
#73223=CARTESIAN_POINT('Ctrl Pts',(1.33326518482319,8.01786348566248,7.03084921190914));
#73224=CARTESIAN_POINT('Ctrl Pts',(1.53997214480885,7.98073963687538,7.02262886282664));
#73225=CARTESIAN_POINT('Ctrl Pts',(1.7449138889492,7.93567659892036,7.01440851374414));
#73226=CARTESIAN_POINT('Ctrl Pts',(1.94989945237117,7.89060392588606,7.00618640704123));
#73227=CARTESIAN_POINT('Ctrl Pts',(2.15311875760632,7.83758873579499,6.99796430033833));
#73228=CARTESIAN_POINT('Ctrl Pts',(2.35395334534642,7.77679826216627,6.98974219363543));
#73229=CARTESIAN_POINT('Ctrl Pts',(2.44203020894514,7.7501383411131,6.98613635373148));
#73230=CARTESIAN_POINT('Ctrl Pts',(2.52964859970418,7.72198365208525,6.98253051382753));
#73231=CARTESIAN_POINT('Ctrl Pts',(2.61675728791372,7.69235132184239,6.97892467392359));
#73232=CARTESIAN_POINT('Ctrl Pts',(2.81538378825199,7.62478325057437,6.97070258522472));
#73233=CARTESIAN_POINT('Ctrl Pts',(3.01142462280939,7.5495067262633,6.96248049652585));
#73234=CARTESIAN_POINT('Ctrl Pts',(3.20427948755665,7.46674497543097,6.95425840782698));
#73235=CARTESIAN_POINT('Ctrl Pts',(3.39710413541919,7.38399619187477,6.94603760738136));
#73236=CARTESIAN_POINT('Ctrl Pts',(3.58674353824727,7.29376463787685,6.93781680693574));
#73237=CARTESIAN_POINT('Ctrl Pts',(3.7726174297204,7.19632165008415,6.92959600649013));
#73238=CARTESIAN_POINT('Ctrl Pts',(3.95846688806202,7.09889147117664,6.9213762866691));
#73239=CARTESIAN_POINT('Ctrl Pts',(4.14055156224465,6.99425188856954,6.91315656684808));
#73240=CARTESIAN_POINT('Ctrl Pts',(4.31831518978921,6.88272050021906,6.90493684702706));
#73241=CARTESIAN_POINT('Ctrl Pts',(4.4960786909369,6.77118919117176,6.89671713305057));
#73242=CARTESIAN_POINT('Ctrl Pts',(4.66952090125097,6.65276624237792,6.88849741907409));
#73243=CARTESIAN_POINT('Ctrl Pts',(4.8381131863584,6.52781344390945,6.88027770509761));
#73244=CARTESIAN_POINT('Ctrl Pts',(4.87455687045246,6.50080307204604,6.87850089390301));
#73245=CARTESIAN_POINT('Ctrl Pts',(4.9107740419292,6.47348773790737,6.8767240827084));
#73246=CARTESIAN_POINT('Ctrl Pts',(4.94675954817621,6.44587135576157,6.8749472715138));
#73247=CARTESIAN_POINT('Ctrl Pts',(4.9467595481762,6.44587135576158,8.87494054454767));
#73248=CARTESIAN_POINT('Ctrl Pts',(5.11320844408724,6.31813336353569,8.86671903882184));
#73249=CARTESIAN_POINT('Ctrl Pts',(5.27473107141465,6.18392618048737,8.85849753309601));
#73250=CARTESIAN_POINT('Ctrl Pts',(5.43083107949353,6.0436546351117,8.85027602737019));
#73251=CARTESIAN_POINT('Ctrl Pts',(5.58690664532328,5.90340505355332,8.84205580897351));
#73252=CARTESIAN_POINT('Ctrl Pts',(5.73756106725395,5.75709320220086,8.83383559057684));
#73253=CARTESIAN_POINT('Ctrl Pts',(5.88233252242706,5.60516294661421,8.82561537218016));
#73254=CARTESIAN_POINT('Ctrl Pts',(6.02903899773482,5.45120198612603,8.81728528206817));
#73255=CARTESIAN_POINT('Ctrl Pts',(6.16970388967293,5.29147156466319,8.80895519195618));
#73256=CARTESIAN_POINT('Ctrl Pts',(6.30388591896933,5.12647148466859,8.80062510184419));
#73257=CARTESIAN_POINT('Ctrl Pts',(6.43629937652069,4.96364617040781,8.79240480558524));
#73258=CARTESIAN_POINT('Ctrl Pts',(6.56239963966013,4.7956895020486,8.7841845093263));
#73259=CARTESIAN_POINT('Ctrl Pts',(6.6818033980155,4.62311484961909,8.77596421306735));
#73260=CARTESIAN_POINT('Ctrl Pts',(6.80359936918501,4.44708272398585,8.76757922602884));
#73261=CARTESIAN_POINT('Ctrl Pts',(6.91842749572302,4.26624588128782,8.75919423899032));
#73262=CARTESIAN_POINT('Ctrl Pts',(7.02592720131281,4.08118053072303,8.75080925195181));
#73263=CARTESIAN_POINT('Ctrl Pts',(7.13342690690261,3.89611518015824,8.74242426491329));
#73264=CARTESIAN_POINT('Ctrl Pts',(7.23359803514733,3.70682160736471,8.73403927787478));
#73265=CARTESIAN_POINT('Ctrl Pts',(7.32612922650988,3.51390354434748,8.72565429083627));
#73266=CARTESIAN_POINT('Ctrl Pts',(7.41686356605974,3.32473173344402,8.7174321308287));
#73267=CARTESIAN_POINT('Ctrl Pts',(7.50028190538392,3.13201247964481,8.70920997082113));
#73268=CARTESIAN_POINT('Ctrl Pts',(7.57612360073261,2.93633083097296,8.70098781081357));
#73269=CARTESIAN_POINT('Ctrl Pts',(7.65195131623721,2.74068525215593,8.69276716639072));
#73270=CARTESIAN_POINT('Ctrl Pts',(7.72020506857548,2.54207864337667,8.68454652196788));
#73271=CARTESIAN_POINT('Ctrl Pts',(7.78067262180944,2.34111535698798,8.67632587754504));
#73272=CARTESIAN_POINT('Ctrl Pts',(7.84113338192164,2.14017464746909,8.66810615665615));
#73273=CARTESIAN_POINT('Ctrl Pts',(7.89380960425461,1.93687807142458,8.65988643576727));
#73274=CARTESIAN_POINT('Ctrl Pts',(7.93853888428697,1.73184524284469,8.65166671487838));
#73275=CARTESIAN_POINT('Ctrl Pts',(7.98327174830661,1.5267959857632,8.64344633537448));
#73276=CARTESIAN_POINT('Ctrl Pts',(8.02005633214138,1.32001048596106,8.63522595587059));
#73277=CARTESIAN_POINT('Ctrl Pts',(8.04878110854307,1.11211970095856,8.6270055763667));
#73278=CARTESIAN_POINT('Ctrl Pts',(8.07750577864218,0.904229685303227,8.61878522728419));
#73279=CARTESIAN_POINT('Ctrl Pts',(8.0981706632209,0.695234685361304,8.61056487820168));
#73280=CARTESIAN_POINT('Ctrl Pts',(8.11071591497123,0.485772487006474,8.60234452911917));
#73281=CARTESIAN_POINT('Ctrl Pts',(8.12326384906389,0.276265502836732,8.59412242241627));
#73282=CARTESIAN_POINT('Ctrl Pts',(8.12768866431693,0.0662914153624913,
8.58590031571336));
#73283=CARTESIAN_POINT('Ctrl Pts',(8.123982563112,-0.143509152154886,8.57767820901045));
#73284=CARTESIAN_POINT('Ctrl Pts',(8.12235723664817,-0.235518084360483,
8.57407236910655));
#73285=CARTESIAN_POINT('Ctrl Pts',(8.11916876765902,-0.327493638605861,
8.57046652920265));
#73286=CARTESIAN_POINT('Ctrl Pts',(8.11441966015929,-0.419381856212609,
8.56686068929876));
#73287=CARTESIAN_POINT('Ctrl Pts',(8.10359058210908,-0.62890852631129,8.55863852929119));
#73288=CARTESIAN_POINT('Ctrl Pts',(8.08463993274142,-0.838050112345938,
8.55041636928362));
#73289=CARTESIAN_POINT('Ctrl Pts',(8.05761873788753,-1.04616816876821,8.54219420927605));
#73290=CARTESIAN_POINT('Ctrl Pts',(8.03060252383067,-1.25424786294171,8.53397356485321));
#73291=CARTESIAN_POINT('Ctrl Pts',(7.99551877138917,-1.46130411151605,8.52575292043037));
#73292=CARTESIAN_POINT('Ctrl Pts',(7.95247025031508,-1.66670467700599,8.51753227600752));
#73293=CARTESIAN_POINT('Ctrl Pts',(7.90942656545197,-1.87208216712783,8.50931255511864));
#73294=CARTESIAN_POINT('Ctrl Pts',(7.85841995885542,-2.0758040567574,8.50109283422974));
#73295=CARTESIAN_POINT('Ctrl Pts',(7.79960426016178,-2.27724854756045,8.49287311334086));
#73296=CARTESIAN_POINT('Ctrl Pts',(7.74078384878968,-2.47870917934514,8.48465273383696));
#73297=CARTESIAN_POINT('Ctrl Pts',(7.67415317518488,-2.67789176360212,8.47643235433307));
#73298=CARTESIAN_POINT('Ctrl Pts',(7.59991617272585,-2.87418888210919,8.46821197482918));
#73299=CARTESIAN_POINT('Ctrl Pts',(7.52567944499771,-3.07048527417417,8.45999162574667));
#73300=CARTESIAN_POINT('Ctrl Pts',(7.44383655162332,-3.26389594673264,8.45177127666416));
#73301=CARTESIAN_POINT('Ctrl Pts',(7.35464007437481,-3.45383221058871,8.44355092758165));
#73302=CARTESIAN_POINT('Ctrl Pts',(7.26542452572847,-3.64380908535411,8.43532882087874));
#73303=CARTESIAN_POINT('Ctrl Pts',(7.16885237755272,-3.83030980009103,8.42710671417583));
#73304=CARTESIAN_POINT('Ctrl Pts',(7.06522327530623,-4.01276807610048,8.41888460747293));
#73305=CARTESIAN_POINT('Ctrl Pts',(7.01977629126834,-4.0927859299429,8.41527876756903));
#73306=CARTESIAN_POINT('Ctrl Pts',(6.97297263975525,-4.17202662099389,8.41167292766515));
#73307=CARTESIAN_POINT('Ctrl Pts',(6.92484033500501,-4.25044396471565,8.40806708776126));
#73308=CARTESIAN_POINT('Ctrl Pts',(6.81508740039395,-4.42925388546487,8.39984492775369));
#73309=CARTESIAN_POINT('Ctrl Pts',(6.69838693633129,-4.60384005848017,8.39162276774611));
#73310=CARTESIAN_POINT('Ctrl Pts',(6.57508920080886,-4.77366626021412,8.38340060773854));
#73311=CARTESIAN_POINT('Ctrl Pts',(6.45181419266758,-4.94346115800889,8.37517996331569));
#73312=CARTESIAN_POINT('Ctrl Pts',(6.32194451348697,-5.10849759698116,8.36695931889285));
#73313=CARTESIAN_POINT('Ctrl Pts',(6.18587288883578,-5.26826956083935,8.35873867447));
#73314=CARTESIAN_POINT('Ctrl Pts',(6.04981655091383,-5.42802357539506,8.3505189535811));
#73315=CARTESIAN_POINT('Ctrl Pts',(5.90755984981741,-5.58251407097313,8.34229923269221));
#73316=CARTESIAN_POINT('Ctrl Pts',(5.75953535374654,-5.73126862670419,8.33407951180331));
#73317=CARTESIAN_POINT('Ctrl Pts',(5.61149899703531,-5.8800351015725,8.32585913229942));
#73318=CARTESIAN_POINT('Ctrl Pts',(5.45769412818033,-6.02306450712544,8.31763875279552));
#73319=CARTESIAN_POINT('Ctrl Pts',(5.29859043292924,-6.15992102113093,8.30941837329163));
#73320=CARTESIAN_POINT('Ctrl Pts',(5.13948732647769,-6.29677702866765,8.30119802420912));
#73321=CARTESIAN_POINT('Ctrl Pts',(4.97508565835178,-6.42745999991004,8.29297767512662));
#73322=CARTESIAN_POINT('Ctrl Pts',(4.80588887322038,-6.55157383387813,8.28475732604412));
#73323=CARTESIAN_POINT('Ctrl Pts',(4.63665591155685,-6.67571420504135,8.2765352193412));
#73324=CARTESIAN_POINT('Ctrl Pts',(4.462626022647,-6.79328245826792,8.2683131126383));
#73325=CARTESIAN_POINT('Ctrl Pts',(4.28433325718575,-6.90392468845599,8.26009100593539));
#73326=CARTESIAN_POINT('Ctrl Pts',(4.20614220573086,-6.95244730961417,8.2564851660315));
#73327=CARTESIAN_POINT('Ctrl Pts',(4.12713164619852,-6.99963841466141,8.2528793261276));
#73328=CARTESIAN_POINT('Ctrl Pts',(4.04734827464875,-7.0454708505676,8.24927348622371));
#73329=CARTESIAN_POINT('Ctrl Pts',(3.8654234903237,-7.14997954524122,8.24105132621614));
#73330=CARTESIAN_POINT('Ctrl Pts',(3.67941866156424,-7.24745535659331,8.23282916620857));
#73331=CARTESIAN_POINT('Ctrl Pts',(3.48989790400209,-7.33759498624323,8.224607006201));
#73332=CARTESIAN_POINT('Ctrl Pts',(3.30041208066243,-7.4277180005212,8.21638636177816));
#73333=CARTESIAN_POINT('Ctrl Pts',(3.10741188841331,-7.51050740534339,8.20816571735532));
#73334=CARTESIAN_POINT('Ctrl Pts',(2.91148428275235,-7.58570674583364,8.19994507293248));
#73335=CARTESIAN_POINT('Ctrl Pts',(2.71557868823589,-7.66089763818539,8.19172535204357));
#73336=CARTESIAN_POINT('Ctrl Pts',(2.5167466123199,-7.72850006283006,8.18350563115468));
#73337=CARTESIAN_POINT('Ctrl Pts',(2.31559392433724,-7.78830612778366,8.17528591026577));
#73338=CARTESIAN_POINT('Ctrl Pts',(2.11442511875439,-7.84811698476988,8.16706553076188));
#73339=CARTESIAN_POINT('Ctrl Pts',(1.91093561171014,-7.90013014713468,8.15884515125798));
#73340=CARTESIAN_POINT('Ctrl Pts',(1.70574635657988,-7.9441876192292,8.15062477175409));
#73341=CARTESIAN_POINT('Ctrl Pts',(1.50055786079896,-7.98824492827905,8.14240442267157));
#73342=CARTESIAN_POINT('Ctrl Pts',(1.29366991864227,-8.02434654660311,8.13418407358906));
#73343=CARTESIAN_POINT('Ctrl Pts',(1.08571412428032,-8.05238551007329,8.12596372450655));
#73344=CARTESIAN_POINT('Ctrl Pts',(0.877713866193068,-8.0804304686482,8.11774161780365));
#73345=CARTESIAN_POINT('Ctrl Pts',(0.668645592315945,-8.10040928889974,
8.10951951110075));
#73346=CARTESIAN_POINT('Ctrl Pts',(0.459147585041741,-8.11226670281804,
8.10129740439785));
#73347=CARTESIAN_POINT('Ctrl Pts',(0.367271341919506,-8.1174668221802,8.09769156449397));
#73348=CARTESIAN_POINT('Ctrl Pts',(0.275312503188222,-8.12110562587664,
8.09408572459009));
#73349=CARTESIAN_POINT('Ctrl Pts',(0.183325064680515,-8.12318161086898,
8.09047988468621));
#73350=CARTESIAN_POINT('Ctrl Pts',(-0.0264278523258185,-8.12791534315752,
8.08225772467864));
#73351=CARTESIAN_POINT('Ctrl Pts',(-0.23639882799153,-8.12452130448339,
8.07403556467107));
#73352=CARTESIAN_POINT('Ctrl Pts',(-0.445947390837542,-8.11300304986416,
8.0658134046635));
#73353=CARTESIAN_POINT('Ctrl Pts',(-0.655457327750723,-8.10148691839635,
8.05759276024066));
#73354=CARTESIAN_POINT('Ctrl Pts',(-0.864544712698323,-8.08184957603862,
8.04937211581781));
#73355=CARTESIAN_POINT('Ctrl Pts',(-1.07257142920726,-8.0541466395732,8.04115147139497));
#73356=CARTESIAN_POINT('Ctrl Pts',(-1.28057477531725,-8.0264468153459,8.03293175050609));
#73357=CARTESIAN_POINT('Ctrl Pts',(-1.48751739843576,-7.99068324495086,
8.02471202961722));
#73358=CARTESIAN_POINT('Ctrl Pts',(-1.69276780725117,-7.94696323844738,
8.01649230872834));
#73359=CARTESIAN_POINT('Ctrl Pts',(-1.89803466200229,-7.90323972882582,
8.00827192922445));
#73360=CARTESIAN_POINT('Ctrl Pts',(-2.10160874228074,-7.85155856808936,
8.00005154972057));
#73361=CARTESIAN_POINT('Ctrl Pts',(-2.30286918293556,-7.79207809822166,
7.99183117021667));
#73362=CARTESIAN_POINT('Ctrl Pts',(-2.50412887878015,-7.73259784847503,
7.98361082113418));
#73363=CARTESIAN_POINT('Ctrl Pts',(-2.70307466984352,-7.66531843354412,
7.97539047205168));
#73364=CARTESIAN_POINT('Ctrl Pts',(-2.89910076197325,-7.59044809839486,
7.96717012296918));
#73365=CARTESIAN_POINT('Ctrl Pts',(-3.0951687670989,-7.51556175496824,7.95894801626629));
#73366=CARTESIAN_POINT('Ctrl Pts',(-3.28831555034599,-7.43308135413365,
7.95072590956339));
#73367=CARTESIAN_POINT('Ctrl Pts',(-3.47795417738127,-7.34326373641422,
7.9425038028605));
#73368=CARTESIAN_POINT('Ctrl Pts',(-3.56112100474076,-7.30387383772379,
7.93889796295656));
#73369=CARTESIAN_POINT('Ctrl Pts',(-3.64361338276509,-7.26307339065166,
7.93529212305263));
#73370=CARTESIAN_POINT('Ctrl Pts',(-3.72538317719994,-7.22088690851309,
7.9316862831487));
#73371=CARTESIAN_POINT('Ctrl Pts',(-3.9118374712177,-7.12469184285827,7.92346412314114));
#73372=CARTESIAN_POINT('Ctrl Pts',(-4.09459468685995,-7.02125524270543,
7.91524196313357));
#73373=CARTESIAN_POINT('Ctrl Pts',(-4.27309411014204,-6.91088664994365,
7.90701980312601));
#73374=CARTESIAN_POINT('Ctrl Pts',(-4.4515606307568,-6.80053840134335,7.89879915870315));
#73375=CARTESIAN_POINT('Ctrl Pts',(-4.6257706745293,-6.68326086552329,7.89057851428029));
#73376=CARTESIAN_POINT('Ctrl Pts',(-4.79519050332591,-6.5594081744707,7.88235786985743));
#73377=CARTESIAN_POINT('Ctrl Pts',(-4.96459129894741,-6.43556939743261,
7.87413814896852));
#73378=CARTESIAN_POINT('Ctrl Pts',(-5.12920271579681,-6.30515711398618,
7.86591842807962));
#73379=CARTESIAN_POINT('Ctrl Pts',(-5.28852156503186,-6.16856767967192,
7.85769870719072));
#73380=CARTESIAN_POINT('Ctrl Pts',(-5.44785317988055,-6.03196730096561,
7.84947832768683));
#73381=CARTESIAN_POINT('Ctrl Pts',(-5.60189115392101,-5.88918897246384,
7.84125794818294));
#73382=CARTESIAN_POINT('Ctrl Pts',(-5.7501660445744,-5.74066877831525,7.83303756867906));
#73383=CARTESIAN_POINT('Ctrl Pts',(-5.89844038650325,-5.59214913379901,
7.82481721959653));
#73384=CARTESIAN_POINT('Ctrl Pts',(-6.04095148107157,-5.43788787689858,
7.81659687051401));
#73385=CARTESIAN_POINT('Ctrl Pts',(-6.17726699497406,-5.27835770247755,
7.80837652143148));
#73386=CARTESIAN_POINT('Ctrl Pts',(-6.3136116549533,-5.11879341837543,7.80015441472858));
#73387=CARTESIAN_POINT('Ctrl Pts',(-6.44375789600635,-4.95395819052529,
7.79193230802567));
#73388=CARTESIAN_POINT('Ctrl Pts',(-6.56731319565416,-4.78435836373977,
7.78371020132277));
#73389=CARTESIAN_POINT('Ctrl Pts',(-6.62149889840672,-4.70997963755579,
7.78010436141891));
#73390=CARTESIAN_POINT('Ctrl Pts',(-6.6744175022403,-4.6346849479598,7.77649852151505));
#73391=CARTESIAN_POINT('Ctrl Pts',(-6.72603846708451,-4.55851884956062,
7.77289268161119));
#73392=CARTESIAN_POINT('Ctrl Pts',(-6.84374636427645,-4.38484229572363,
7.76467052160362));
#73393=CARTESIAN_POINT('Ctrl Pts',(-6.95474319978445,-4.20657555000885,
7.75644836159605));
#73394=CARTESIAN_POINT('Ctrl Pts',(-7.05868468976772,-4.02425869110558,
7.74822620158848));
#73395=CARTESIAN_POINT('Ctrl Pts',(-7.16260702029215,-3.84197543853559,
7.74000555716566));
#73396=CARTESIAN_POINT('Ctrl Pts',(-7.25947645481937,-3.65564381906843,
7.73178491274283));
#73397=CARTESIAN_POINT('Ctrl Pts',(-7.34899373090753,-3.46583016109876,
7.72356426832001));
#73398=CARTESIAN_POINT('Ctrl Pts',(-7.4385009503334,-3.2760378274135,7.71534454743114));
#73399=CARTESIAN_POINT('Ctrl Pts',(-7.52065753445803,-3.08276450303734,
7.70712482654229));
#73400=CARTESIAN_POINT('Ctrl Pts',(-7.59521124794654,-2.88659897830758,
7.69890510565342));
#73401=CARTESIAN_POINT('Ctrl Pts',(-7.66977093514102,-2.69041773557919,
7.69068472614954));
#73402=CARTESIAN_POINT('Ctrl Pts',(-7.73672642706943,-2.49134410438495,
7.68246434664565));
#73403=CARTESIAN_POINT('Ctrl Pts',(-7.79587412919473,-2.28998561660382,
7.67424396714176));
#73404=CARTESIAN_POINT('Ctrl Pts',(-7.85502161243047,-2.08862787399564,
7.66602361805926));
#73405=CARTESIAN_POINT('Ctrl Pts',(-7.90636128304193,-1.88498557564683,
7.65780326897677));
#73406=CARTESIAN_POINT('Ctrl Pts',(-7.94973964874673,-1.67968064811268,
7.64958291989427));
#73407=CARTESIAN_POINT('Ctrl Pts',(-7.99312728932537,-1.47433182364348,
7.64136081319136));
#73408=CARTESIAN_POINT('Ctrl Pts',(-8.02855016324043,-1.26731994861156,
7.63313870648846));
#73409=CARTESIAN_POINT('Ctrl Pts',(-8.05590583625226,-1.05927745182114,
7.62491659978555));
#73410=CARTESIAN_POINT('Ctrl Pts',(-8.06790278313099,-0.968039529016909,
7.62131075988159));
#73411=CARTESIAN_POINT('Ctrl Pts',(-8.07834883374,-0.876603491590593,7.61770491997762));
#73412=CARTESIAN_POINT('Ctrl Pts',(-8.08723848625962,-0.785023075368658,
7.61409908007365));
#73413=CARTESIAN_POINT('Ctrl Pts',(-8.10880793006934,-0.56281656758756,
7.60535003605603));
#73414=CARTESIAN_POINT('Ctrl Pts',(-8.12121555449676,-0.339714641363502,
7.59660099203841));
#73415=CARTESIAN_POINT('Ctrl Pts',(-8.12441558747629,-0.116442794849301,
7.58785194802079));
#73416=CARTESIAN_POINT('Ctrl Pts',(-8.12497086969009,-0.0776997925098787,
7.58633377975132));
#73417=CARTESIAN_POINT('Ctrl Pts',(-8.1252490328812,-0.0389516823687162,
7.58481561148186));
#73418=CARTESIAN_POINT('Ctrl Pts',(-8.12524999748248,-0.000202264369551694,
7.58329744321239));
#73419=CARTESIAN_POINT('Origin',(0.,0.,24.4167025567876));
#73420=CARTESIAN_POINT('',(4.94675954817619,6.44587135576159,10.8749423500932));
#73421=CARTESIAN_POINT('',(4.9467595481762,6.44587135576158,10.7083502273763));
#73422=CARTESIAN_POINT('',(4.9467595481762,6.44587135576158,24.4167025567876));
#73423=CARTESIAN_POINT('',(-8.12524999762442,0.000196479806862634,9.41670255674903));
#73424=CARTESIAN_POINT('Ctrl Pts',(4.9467595481762,6.44587135576158,10.7083502273763));
#73425=CARTESIAN_POINT('Ctrl Pts',(5.11325096527104,6.31810073147397,10.7001299359995));
#73426=CARTESIAN_POINT('Ctrl Pts',(5.27478576238475,6.18387897582806,10.6919096446227));
#73427=CARTESIAN_POINT('Ctrl Pts',(5.43087265766335,6.04361727268899,10.6836893532459));
#73428=CARTESIAN_POINT('Ctrl Pts',(5.5869968406379,5.90332206234399,10.6754670981186));
#73429=CARTESIAN_POINT('Ctrl Pts',(5.73767030074121,5.75698421778979,10.6672448429912));
#73430=CARTESIAN_POINT('Ctrl Pts',(5.88243667227605,5.60505364462838,10.6590225878639));
#73431=CARTESIAN_POINT('Ctrl Pts',(5.99894154973237,5.48278317103445,10.6524054929138));
#73432=CARTESIAN_POINT('Ctrl Pts',(6.11162122338302,5.35689124117962,10.6457883979637));
#73433=CARTESIAN_POINT('Ctrl Pts',(6.22025579367875,5.2276290441945,10.6391713030136));
#73434=CARTESIAN_POINT('Ctrl Pts',(6.35524113483892,5.06701256905541,10.630949143006));
#73435=CARTESIAN_POINT('Ctrl Pts',(6.4840243824159,4.90113850458407,10.6227269829984));
#73436=CARTESIAN_POINT('Ctrl Pts',(6.60620740934068,4.73050855905286,10.6145048229909));
#73437=CARTESIAN_POINT('Ctrl Pts',(6.72836791435707,4.55991006561525,10.606284178568));
#73438=CARTESIAN_POINT('Ctrl Pts',(6.84393045516928,4.38455768063056,10.5980635341452));
#73439=CARTESIAN_POINT('Ctrl Pts',(6.95253898010046,4.20498386354617,10.5898428897224));
#73440=CARTESIAN_POINT('Ctrl Pts',(7.06113530359661,4.02543022036859,10.5816231688335));
#73441=CARTESIAN_POINT('Ctrl Pts',(7.16277901821338,3.84165634434287,10.5734034479446));
#73442=CARTESIAN_POINT('Ctrl Pts',(7.25715853317428,3.65422188528224,10.5651837270558));
#73443=CARTESIAN_POINT('Ctrl Pts',(7.35154561040727,3.46677240781028,10.5569633475519));
#73444=CARTESIAN_POINT('Ctrl Pts',(7.43866718980509,3.27566202363514,10.548742968048));
#73445=CARTESIAN_POINT('Ctrl Pts',(7.51825813012694,3.08147403871591,10.5405225885441));
#73446=CARTESIAN_POINT('Ctrl Pts',(7.59784877590435,2.88728677243362,10.5323022394616));
#73447=CARTESIAN_POINT('Ctrl Pts',(7.66990872889148,2.69002220229786,10.5240818903791));
#73448=CARTESIAN_POINT('Ctrl Pts',(7.73422119917883,2.49028311737297,10.5158615412966));
#73449=CARTESIAN_POINT('Ctrl Pts',(7.79854742033114,2.29050132556445,10.5076394345937));
#73450=CARTESIAN_POINT('Ctrl Pts',(7.85512275891198,2.08824424295622,10.4994173278907));
#73451=CARTESIAN_POINT('Ctrl Pts',(7.90378012831557,1.88413036856366,10.4911952211878));
#73452=CARTESIAN_POINT('Ctrl Pts',(7.92511902484832,1.79461535984148,10.4875893812839));
#73453=CARTESIAN_POINT('Ctrl Pts',(7.94493571247724,1.70474340757218,10.48398354138));
#73454=CARTESIAN_POINT('Ctrl Pts',(7.96321917898028,1.61456739407823,10.4803777014761));
#73455=CARTESIAN_POINT('Ctrl Pts',(8.00490976732789,1.40894495061114,10.4721555414685));
#73456=CARTESIAN_POINT('Ctrl Pts',(8.03863875133913,1.20167294150668,10.463933381461));
#73457=CARTESIAN_POINT('Ctrl Pts',(8.06429655698148,0.993382405499821,10.4557112214534));
#73458=CARTESIAN_POINT('Ctrl Pts',(8.08994963313922,0.785130263535682,10.4474905770306));
#73459=CARTESIAN_POINT('Ctrl Pts',(8.10753446421489,0.575860262162351,10.4392699326078));
#73460=CARTESIAN_POINT('Ctrl Pts',(8.11699313593587,0.36621031344013,10.4310492881849));
#73461=CARTESIAN_POINT('Ctrl Pts',(8.12645074503888,0.156583917475535,10.4228295672961));
#73462=CARTESIAN_POINT('Ctrl Pts',(8.127784004069,-0.0534220458940956,10.4146098464072));
#73463=CARTESIAN_POINT('Ctrl Pts',(8.1209870496964,-0.263167059419303,10.4063901255184));
#73464=CARTESIAN_POINT('Ctrl Pts',(8.11418955070965,-0.472928879016114,
10.3981697460145));
#73465=CARTESIAN_POINT('Ctrl Pts',(8.09926054350255,-0.682429411903492,
10.3899493665106));
#73466=CARTESIAN_POINT('Ctrl Pts',(8.07624627108753,-0.891029590555041,
10.3817289870067));
#73467=CARTESIAN_POINT('Ctrl Pts',(8.05323208384199,-1.0996289972349,10.3735086379242));
#73468=CARTESIAN_POINT('Ctrl Pts',(8.02213272626158,-1.30732776327298,10.3652882888416));
#73469=CARTESIAN_POINT('Ctrl Pts',(7.98304622121398,-1.51349284519658,10.3570679397591));
#73470=CARTESIAN_POINT('Ctrl Pts',(7.94395135894986,-1.7197020079666,10.3488458330562));
#73471=CARTESIAN_POINT('Ctrl Pts',(7.89686599243614,-1.92437654146016,10.3406237263533));
#73472=CARTESIAN_POINT('Ctrl Pts',(7.84193930641168,-2.12689338638669,10.3324016196504));
#73473=CARTESIAN_POINT('Ctrl Pts',(7.81785097438013,-2.21570801103744,10.3287957797465));
#73474=CARTESIAN_POINT('Ctrl Pts',(7.7922551786284,-2.30410780828417,10.3251899398425));
#73475=CARTESIAN_POINT('Ctrl Pts',(7.76516754947252,-2.39204107220568,10.3215840999386));
#73476=CARTESIAN_POINT('Ctrl Pts',(7.70340140702625,-2.59254952105839,10.313361939931));
#73477=CARTESIAN_POINT('Ctrl Pts',(7.63385477089133,-2.79069743430204,10.3051397799235));
#73478=CARTESIAN_POINT('Ctrl Pts',(7.55673332847167,-2.98587825687275,10.2969176199159));
#73479=CARTESIAN_POINT('Ctrl Pts',(7.47962610179115,-3.18102310190504,10.2886969754931));
#73480=CARTESIAN_POINT('Ctrl Pts',(7.39494696397008,-3.37320167349059,10.2804763310703));
#73481=CARTESIAN_POINT('Ctrl Pts',(7.30295025460098,-3.56182609644596,10.2722556866475));
#73482=CARTESIAN_POINT('Ctrl Pts',(7.2109638804418,-3.75042932871941,10.2640359657586));
#73483=CARTESIAN_POINT('Ctrl Pts',(7.11166170528859,-3.9354789443369,10.2558162448697));
#73484=CARTESIAN_POINT('Ctrl Pts',(7.00534502243036,-4.11640968311102,10.2475965239809));
#73485=CARTESIAN_POINT('Ctrl Pts',(6.89901982081973,-4.29735491917872,10.239376144477));
#73486=CARTESIAN_POINT('Ctrl Pts',(6.78567913565673,-4.47418036311471,10.2311557649731));
#73487=CARTESIAN_POINT('Ctrl Pts',(6.66566932258686,-4.64634695695708,10.2229353854692));
#73488=CARTESIAN_POINT('Ctrl Pts',(6.54565995364141,-4.81851291365667,10.2147150363867));
#73489=CARTESIAN_POINT('Ctrl Pts',(6.41898167712468,-4.98601981415219,10.2064946873043));
#73490=CARTESIAN_POINT('Ctrl Pts',(6.28602343584947,-5.14835866334613,10.1982743382218));
#73491=CARTESIAN_POINT('Ctrl Pts',(6.15303676632627,-5.31073222275451,10.1900522315189));
#73492=CARTESIAN_POINT('Ctrl Pts',(6.01376763655867,-5.4679352949076,10.181830124816));
#73493=CARTESIAN_POINT('Ctrl Pts',(5.86864513921844,-5.61949212940349,10.1736080181131));
#73494=CARTESIAN_POINT('Ctrl Pts',(5.80500105008321,-5.68595802449553,10.1700021782091));
#73495=CARTESIAN_POINT('Ctrl Pts',(5.7402316829715,-5.75133843438792,10.1663963383051));
#73496=CARTESIAN_POINT('Ctrl Pts',(5.6743755008865,-5.81559543275142,10.1627904984011));
#73497=CARTESIAN_POINT('Ctrl Pts',(5.52420797237592,-5.9621164476092,10.1545683383935));
#73498=CARTESIAN_POINT('Ctrl Pts',(5.36833753695209,-6.10284220033841,10.146346178386));
#73499=CARTESIAN_POINT('Ctrl Pts',(5.20723500765842,-6.23733846584555,10.1381240183784));
#73500=CARTESIAN_POINT('Ctrl Pts',(5.04616217427546,-6.37180993975503,10.1299033739556));
#73501=CARTESIAN_POINT('Ctrl Pts',(4.87985939833995,-6.50005402919111,10.1216827295327));
#73502=CARTESIAN_POINT('Ctrl Pts',(4.70883127866183,-6.62167618897179,10.1134620851099));
#73503=CARTESIAN_POINT('Ctrl Pts',(4.5378223728397,-6.74328468532293,10.105242364221));
#73504=CARTESIAN_POINT('Ctrl Pts',(4.36208942353297,-6.85827256624359,10.0970226433321));
#73505=CARTESIAN_POINT('Ctrl Pts',(4.18216744115413,-6.96628760938352,10.0888029224432));
#73506=CARTESIAN_POINT('Ctrl Pts',(4.00223104231048,-7.07431130735843,10.0805825429393));
#73507=CARTESIAN_POINT('Ctrl Pts',(3.81810519137809,-7.1753608969403,10.0723621634355));
#73508=CARTESIAN_POINT('Ctrl Pts',(3.63035193330211,-7.26912872377905,10.0641417839316));
#73509=CARTESIAN_POINT('Ctrl Pts',(3.44259937005134,-7.36289620360784,10.0559214348491));
#73510=CARTESIAN_POINT('Ctrl Pts',(3.25121969174863,-7.4493818451175,10.0477010857667));
#73511=CARTESIAN_POINT('Ctrl Pts',(3.0567979573016,-7.52832476788407,10.0394807366843));
#73512=CARTESIAN_POINT('Ctrl Pts',(2.86233465288943,-7.60728456970255,10.0312586299813));
#73513=CARTESIAN_POINT('Ctrl Pts',(2.66482826641217,-7.67869831979012,10.0230365232784));
#73514=CARTESIAN_POINT('Ctrl Pts',(2.46488320819504,-7.74235353961947,10.0148144165755));
#73515=CARTESIAN_POINT('Ctrl Pts',(2.377196451556,-7.77026980731696,10.0112085766715));
#73516=CARTESIAN_POINT('Ctrl Pts',(2.28904088641286,-7.79669451635676,10.0076027367676));
#73517=CARTESIAN_POINT('Ctrl Pts',(2.20046843319389,-7.82161276445064,10.0039968968636));
#73518=CARTESIAN_POINT('Ctrl Pts',(1.99850248295017,-7.87843220968209,9.99577473685601));
#73519=CARTESIAN_POINT('Ctrl Pts',(1.79430128204897,-7.92743424710151,9.98755257684843));
#73520=CARTESIAN_POINT('Ctrl Pts',(1.58848600965627,-7.96846282288035,9.97933041684084));
#73521=CARTESIAN_POINT('Ctrl Pts',(1.38270867504208,-8.00948383589185,9.97110977241799));
#73522=CARTESIAN_POINT('Ctrl Pts',(1.1753181520486,-8.04253426299419,9.96288912799513));
#73523=CARTESIAN_POINT('Ctrl Pts',(0.966946303989035,-8.06750905842082,
9.95466848357228));
#73524=CARTESIAN_POINT('Ctrl Pts',(0.758597865100385,-8.09248104809773,
9.94644876268335));
#73525=CARTESIAN_POINT('Ctrl Pts',(0.549268614172991,-8.10937918223538,
9.93822904179442));
#73526=CARTESIAN_POINT('Ctrl Pts',(0.339596871275645,-8.11815012964898,
9.93000932090549));
#73527=CARTESIAN_POINT('Ctrl Pts',(0.129908328179361,-8.12692177984522,
9.9217889414016));
#73528=CARTESIAN_POINT('Ctrl Pts',(-0.0801224669385747,-8.12756492708978,
9.91356856189771));
#73529=CARTESIAN_POINT('Ctrl Pts',(-0.289854776901162,-8.1200783106327,
9.90534818239382));
#73530=CARTESIAN_POINT('Ctrl Pts',(-0.499586310701988,-8.11259172188153,
9.89712783331131));
#73531=CARTESIAN_POINT('Ctrl Pts',(-0.709019066696316,-8.0969754428084,
9.88890748422879));
#73532=CARTESIAN_POINT('Ctrl Pts',(-0.917514476546098,-8.0732802966222,
9.88068713514627));
#73533=CARTESIAN_POINT('Ctrl Pts',(-1.12605446549789,-8.04958008409743,
9.87246502844338));
#73534=CARTESIAN_POINT('Ctrl Pts',(-1.33365641459504,-8.01779758684553,
9.86424292174049));
#73535=CARTESIAN_POINT('Ctrl Pts',(-1.53968791938338,-7.97803538933019,
9.8560208150376));
#73536=CARTESIAN_POINT('Ctrl Pts',(-1.63004391307954,-7.9605975083045,9.85241497513375));
#73537=CARTESIAN_POINT('Ctrl Pts',(-1.72009797489201,-7.94162555890349,
9.8488091352299));
#73538=CARTESIAN_POINT('Ctrl Pts',(-1.80979738244364,-7.92113129527596,
9.84520329532605));
#73539=CARTESIAN_POINT('Ctrl Pts',(-2.01433305267289,-7.8743995713847,9.83698113531849));
#73540=CARTESIAN_POINT('Ctrl Pts',(-2.21709148047456,-7.81973376785216,
9.82875897531093));
#73541=CARTESIAN_POINT('Ctrl Pts',(-2.41745253144821,-7.75729403985015,
9.82053681530337));
#73542=CARTESIAN_POINT('Ctrl Pts',(-2.61777665001656,-7.69486582131732,
9.81231617088052));
#73543=CARTESIAN_POINT('Ctrl Pts',(-2.81570399210626,-7.62466662607666,
9.80409552645767));
#73544=CARTESIAN_POINT('Ctrl Pts',(-3.01062944502338,-7.54690651242337,
9.79587488203482));
#73545=CARTESIAN_POINT('Ctrl Pts',(-3.20553299938062,-7.46915513459436,
9.78765516114593));
#73546=CARTESIAN_POINT('Ctrl Pts',(-3.39743506381779,-7.38384464347193,
9.77943544025704));
#73547=CARTESIAN_POINT('Ctrl Pts',(-3.58574959755062,-7.29123359838138,
9.77121571936814));
#73548=CARTESIAN_POINT('Ctrl Pts',(-3.77407922021035,-7.19861513272025,
9.7629953398643));
#73549=CARTESIAN_POINT('Ctrl Pts',(-3.95882047173939,-7.09869507207521,
9.75477496036045));
#73550=CARTESIAN_POINT('Ctrl Pts',(-4.13941010083388,-6.99177885660112,
9.7465545808566));
#73551=CARTESIAN_POINT('Ctrl Pts',(-4.31999906161615,-6.88486303679434,
9.73833423177411));
#73552=CARTESIAN_POINT('Ctrl Pts',(-4.49643617808616,-6.77095126660788,
9.73011388269161));
#73553=CARTESIAN_POINT('Ctrl Pts',(-4.66818502193127,-6.65039368485179,
9.72189353360911));
#73554=CARTESIAN_POINT('Ctrl Pts',(-4.83997058797186,-6.52981032627539,
9.71367142690625));
#73555=CARTESIAN_POINT('Ctrl Pts',(-5.00706563713683,-6.40257848692383,
9.70544932020339));
#73556=CARTESIAN_POINT('Ctrl Pts',(-5.16896391786744,-6.26909080954204,
9.69722721350052));
#73557=CARTESIAN_POINT('Ctrl Pts',(-5.23996509823912,-6.21054922024035,
9.69362137359653));
#73558=CARTESIAN_POINT('Ctrl Pts',(-5.30996720149048,-6.15080497822461,
9.69001553369255));
#73559=CARTESIAN_POINT('Ctrl Pts',(-5.37892955424479,-6.08989362903589,
9.68640969378856));
#73560=CARTESIAN_POINT('Ctrl Pts',(-5.53617987981134,-5.95100147834681,
9.67818753378101));
#73561=CARTESIAN_POINT('Ctrl Pts',(-5.68807366831926,-5.80599248851161,
9.66996537377346));
#73562=CARTESIAN_POINT('Ctrl Pts',(-5.83414298636272,-5.65530398627472,
9.66174321376591));
#73563=CARTESIAN_POINT('Ctrl Pts',(-5.98018537955678,-5.50464326033803,
9.65352256934304));
#73564=CARTESIAN_POINT('Ctrl Pts',(-6.12040523976354,-5.34830532328191,
9.64530192492017));
#73565=CARTESIAN_POINT('Ctrl Pts',(-6.25437169963365,-5.18676413627241,
9.6370812804973));
#73566=CARTESIAN_POINT('Ctrl Pts',(-6.38832310927675,-5.02524109732429,
9.62886155960831));
#73567=CARTESIAN_POINT('Ctrl Pts',(-6.51602233279856,-4.85851620253131,
9.62064183871932));
#73568=CARTESIAN_POINT('Ctrl Pts',(-6.63707845469368,-4.68709687853164,
9.61242211783033));
#73569=CARTESIAN_POINT('Ctrl Pts',(-6.75814427635433,-4.51566381935504,
9.60420173832644));
#73570=CARTESIAN_POINT('Ctrl Pts',(-6.87256576033579,-4.33953581891294,
9.59598135882255));
#73571=CARTESIAN_POINT('Ctrl Pts',(-6.97999443232209,-4.15925056798129,
9.58776097931866));
#73572=CARTESIAN_POINT('Ctrl Pts',(-7.08742270674293,-3.97896598423826,
9.57954063023625));
#73573=CARTESIAN_POINT('Ctrl Pts',(-7.18785807214671,-3.79452443569092,
9.57132028115384));
#73574=CARTESIAN_POINT('Ctrl Pts',(-7.28099699332299,-3.60649003127994,
9.56309993207143));
#73575=CARTESIAN_POINT('Ctrl Pts',(-7.37415582884511,-3.41841542260084,
9.55487782536855));
#73576=CARTESIAN_POINT('Ctrl Pts',(-7.46001497237877,-3.22674668787325,
9.54665571866566));
#73577=CARTESIAN_POINT('Ctrl Pts',(-7.53831772282828,-3.03207082242369,
9.53843361196278));
#73578=CARTESIAN_POINT('Ctrl Pts',(-7.57265772744753,-2.94669489270962,
9.53482777205886));
#73579=CARTESIAN_POINT('Ctrl Pts',(-7.60554503229144,-2.86074086957279,
9.53122193215495));
#73580=CARTESIAN_POINT('Ctrl Pts',(-7.6369609270188,-2.77425942580864,9.52761609225104));
#73581=CARTESIAN_POINT('Ctrl Pts',(-7.70849460051845,-2.57734205593301,
9.51940563138029));
#73582=CARTESIAN_POINT('Ctrl Pts',(-7.77242068385816,-2.3776215238446,9.51119517050955));
#73583=CARTESIAN_POINT('Ctrl Pts',(-7.82853754939877,-2.17570388613743,
9.5029847096388));
#73584=CARTESIAN_POINT('Ctrl Pts',(-7.88464584510249,-1.97381708410153,
9.49477550262124));
#73585=CARTESIAN_POINT('Ctrl Pts',(-7.93294722207455,-1.76973413150191,
9.48656629560367));
#73586=CARTESIAN_POINT('Ctrl Pts',(-7.97329009568077,-1.56407564159122,
9.47835708858611));
#73587=CARTESIAN_POINT('Ctrl Pts',(-8.0136274393253,-1.35844534212574,9.47014900683793));
#73588=CARTESIAN_POINT('Ctrl Pts',(-8.04600840102247,-1.15124022782422,
9.46194092508974));
#73589=CARTESIAN_POINT('Ctrl Pts',(-8.07033249590858,-0.943091176918756,
9.45373284334155));
#73590=CARTESIAN_POINT('Ctrl Pts',(-8.0946573894938,-0.734935291289829,
9.44552449207511));
#73591=CARTESIAN_POINT('Ctrl Pts',(-8.11092485171777,-0.525835701756375,
9.43731614080867));
#73592=CARTESIAN_POINT('Ctrl Pts',(-8.11908615222914,-0.31642947900122,
9.42910778954223));
#73593=CARTESIAN_POINT('Ctrl Pts',(-8.12319752730466,-0.210938016740431,
9.42497271195736));
#73594=CARTESIAN_POINT('Ctrl Pts',(-8.12525255032656,-0.105368806605526,
9.42083763437249));
#73595=CARTESIAN_POINT('Ctrl Pts',(-8.12524999762445,0.000196478821525156,
9.41670255678762));
#73596=CARTESIAN_POINT('Ctrl Pts',(-8.12524999762442,0.000196479806864624,
9.41670255674902));
#73597=CARTESIAN_POINT('Ctrl Pts',(-8.12524471491808,0.218658164704561,
9.40814523591463));
#73598=CARTESIAN_POINT('Ctrl Pts',(-8.11642450034241,0.437076972197306,
9.39958791508024));
#73599=CARTESIAN_POINT('Ctrl Pts',(-8.09882569277387,0.65475946771759,9.39103059424584));
#73600=CARTESIAN_POINT('Ctrl Pts',(-8.0836014519127,0.843070563804878,9.38362789306841));
#73601=CARTESIAN_POINT('Ctrl Pts',(-8.0618085813484,1.03083057646112,9.37622519189097));
#73602=CARTESIAN_POINT('Ctrl Pts',(-8.0335019284137,1.21759366320348,9.36882249071354));
#73603=CARTESIAN_POINT('Ctrl Pts',(-8.00206180620298,1.42503091426872,9.36060033070596));
#73604=CARTESIAN_POINT('Ctrl Pts',(-7.96257768277085,1.63128399695455,9.35237817069839));
#73605=CARTESIAN_POINT('Ctrl Pts',(-7.91516329965985,1.83572261036843,9.34415601069081));
#73606=CARTESIAN_POINT('Ctrl Pts',(-7.86775765640737,2.04012353976234,9.33593536626797));
#73607=CARTESIAN_POINT('Ctrl Pts',(-7.81242473763258,2.24271038005284,9.32771472184513));
#73608=CARTESIAN_POINT('Ctrl Pts',(-7.74932916429956,2.44286411120968,9.31949407742229));
#73609=CARTESIAN_POINT('Ctrl Pts',(-7.68624067932869,2.64299535644468,9.31127435653341));
#73610=CARTESIAN_POINT('Ctrl Pts',(-7.6153913695498,2.84069375687948,9.30305463564453));
#73611=CARTESIAN_POINT('Ctrl Pts',(-7.53699563737041,3.03535571634684,9.29483491475565));
#73612=CARTESIAN_POINT('Ctrl Pts',(-7.45859362363877,3.23003327333762,9.28661453525176));
#73613=CARTESIAN_POINT('Ctrl Pts',(-7.37264408705129,3.42167362842161,9.27839415574786));
#73614=CARTESIAN_POINT('Ctrl Pts',(-7.27940987131439,3.6096924367473,9.27017377624397));
#73615=CARTESIAN_POINT('Ctrl Pts',(-7.18617600061185,3.79771054926673,9.26195342716146));
#73616=CARTESIAN_POINT('Ctrl Pts',(-7.08565763819809,3.98210687860411,9.25373307807894));
#73617=CARTESIAN_POINT('Ctrl Pts',(-6.9781641919283,4.1623205154084,9.24551272899642));
#73618=CARTESIAN_POINT('Ctrl Pts',(-6.87064776212451,4.34257268429433,9.23729062229352));
#73619=CARTESIAN_POINT('Ctrl Pts',(-6.75615342022911,4.51864012045031,9.22906851559062));
#73620=CARTESIAN_POINT('Ctrl Pts',(-6.63503519819217,4.68998885726299,9.22084640888772));
#73621=CARTESIAN_POINT('Ctrl Pts',(-6.58191828620201,4.76513457538729,9.2172405689838));
#73622=CARTESIAN_POINT('Ctrl Pts',(-6.52752796543296,4.83937312278643,9.2136347290799));
#73623=CARTESIAN_POINT('Ctrl Pts',(-6.47189666834279,4.91266130287785,9.21002888917599));
#73624=CARTESIAN_POINT('Ctrl Pts',(-6.34504427381251,5.07977552853205,9.20180672916842));
#73625=CARTESIAN_POINT('Ctrl Pts',(-6.21169477128387,5.24200142133564,9.19358456916085));
#73626=CARTESIAN_POINT('Ctrl Pts',(-6.07224959442057,5.39883991479273,9.18536240915328));
#73627=CARTESIAN_POINT('Ctrl Pts',(-5.93283012138445,5.55564949832535,9.17714176473043));
#73628=CARTESIAN_POINT('Ctrl Pts',(-5.78731741259613,5.70707344405449,9.16892112030758));
#73629=CARTESIAN_POINT('Ctrl Pts',(-5.63615218318239,5.85264693369662,9.16070047588474));
#73630=CARTESIAN_POINT('Ctrl Pts',(-5.48500393616324,5.99820406913843,9.15248075499588));
#73631=CARTESIAN_POINT('Ctrl Pts',(-5.32820464880557,6.137911856017,9.14426103410703));
#73632=CARTESIAN_POINT('Ctrl Pts',(-5.16623137140413,6.27134283703417,9.13604131321817));
#73633=CARTESIAN_POINT('Ctrl Pts',(-5.0042451156988,6.40478450936936,9.12782093371428));
#73634=CARTESIAN_POINT('Ctrl Pts',(-4.83708426766641,6.53194818115257,9.11960055421039));
#73635=CARTESIAN_POINT('Ctrl Pts',(-4.66525920478921,6.65244647589363,9.1113801747065));
#73636=CARTESIAN_POINT('Ctrl Pts',(-4.49343477778953,6.77294432470348,9.10315982562398));
#73637=CARTESIAN_POINT('Ctrl Pts',(-4.31694641365142,6.88677667853716,9.09493947654147));
#73638=CARTESIAN_POINT('Ctrl Pts',(-4.13633416683445,6.99359901787184,9.08671912745896));
#73639=CARTESIAN_POINT('Ctrl Pts',(-3.95568330270774,7.10044419724886,9.07849702075606));
#73640=CARTESIAN_POINT('Ctrl Pts',(-3.77090704844366,7.20027621746656,9.07027491405315));
#73641=CARTESIAN_POINT('Ctrl Pts',(-3.58257175390296,7.29279556758838,9.06205280735025));
#73642=CARTESIAN_POINT('Ctrl Pts',(-3.49997650855884,7.33337032252757,9.05844696744633));
#73643=CARTESIAN_POINT('Ctrl Pts',(-3.4166970663496,7.37253923135409,9.05484112754241));
#73644=CARTESIAN_POINT('Ctrl Pts',(-3.33278257356546,7.41027987864415,9.05123528763849));
#73645=CARTESIAN_POINT('Ctrl Pts',(-3.14143786470172,7.49633739896573,9.04301312763092));
#73646=CARTESIAN_POINT('Ctrl Pts',(-2.94672659509682,7.57499394102922,9.03479096762335));
#73647=CARTESIAN_POINT('Ctrl Pts',(-2.74924004207116,7.64600331896165,9.02656880761579));
#73648=CARTESIAN_POINT('Ctrl Pts',(-2.55178989159727,7.71699960778742,9.01834816319296));
#73649=CARTESIAN_POINT('Ctrl Pts',(-2.3515657563126,7.78035144602788,9.01012751877012));
#73650=CARTESIAN_POINT('Ctrl Pts',(-2.14917702228249,7.83586151545527,9.00190687434729));
#73651=CARTESIAN_POINT('Ctrl Pts',(-1.94681102526134,7.89136534870083,8.9936871534584));
#73652=CARTESIAN_POINT('Ctrl Pts',(-1.742281199502,7.93902909389111,8.98546743256951));
#73653=CARTESIAN_POINT('Ctrl Pts',(-1.53621096335487,7.97870562425813,8.97724771168062));
#73654=CARTESIAN_POINT('Ctrl Pts',(-1.33012421558289,8.01838533375473,8.96902733217674));
#73655=CARTESIAN_POINT('Ctrl Pts',(-1.12249710011702,8.0500764911892,8.96080695267286));
#73656=CARTESIAN_POINT('Ctrl Pts',(-0.913963124964075,8.07368311049585,
8.95258657316898));
#73657=CARTESIAN_POINT('Ctrl Pts',(-0.705429921538258,8.09728964244086,
8.94436622408647));
#73658=CARTESIAN_POINT('Ctrl Pts',(-0.495990158709673,8.11281166555987,
8.93614587500396));
#73659=CARTESIAN_POINT('Ctrl Pts',(-0.28628290060111,8.12020502594136,8.92792552592145));
#73660=CARTESIAN_POINT('Ctrl Pts',(-0.0765308042804336,8.12759996712204,
8.91970341921853));
#73661=CARTESIAN_POINT('Ctrl Pts',(0.133488606562358,8.12686276294456,8.91148131251562));
#73662=CARTESIAN_POINT('Ctrl Pts',(0.343134710536223,8.1180013632005,8.9032592058127));
#73663=CARTESIAN_POINT('Ctrl Pts',(0.435075902097195,8.11411515861132,8.89965336590879));
#73664=CARTESIAN_POINT('Ctrl Pts',(0.526945307312809,8.10866710404108,8.89604752600489));
#73665=CARTESIAN_POINT('Ctrl Pts',(0.618689045347321,8.10166102892902,8.89244168610098));
#73666=CARTESIAN_POINT('Ctrl Pts',(0.827886268162179,8.08568553580354,8.88421952609341));
#73667=CARTESIAN_POINT('Ctrl Pts',(1.0364989135919,8.06160038919091,8.87599736608584));
#73668=CARTESIAN_POINT('Ctrl Pts',(1.24388998304645,8.02947229103985,8.86777520607827));
#73669=CARTESIAN_POINT('Ctrl Pts',(1.45124282425733,7.99735011503754,8.85955456165543));
#73670=CARTESIAN_POINT('Ctrl Pts',(1.65737424738856,7.95718799162515,8.85133391723258));
#73671=CARTESIAN_POINT('Ctrl Pts',(1.86165473178512,7.90910419846155,8.84311327280973));
#73672=CARTESIAN_POINT('Ctrl Pts',(2.06591226664706,7.8610258071878,8.83489355192084));
#73673=CARTESIAN_POINT('Ctrl Pts',(2.26831899073408,7.80502759047416,8.82667383103195));
#73674=CARTESIAN_POINT('Ctrl Pts',(2.46825707432388,7.74127861386929,8.81845411014306));
#73675=CARTESIAN_POINT('Ctrl Pts',(2.66821117819268,7.67752452930114,8.81023373063917));
#73676=CARTESIAN_POINT('Ctrl Pts',(2.86569596429976,7.60601853100322,8.80201335113527));
#73677=CARTESIAN_POINT('Ctrl Pts',(3.06010921012636,7.52697941970083,8.79379297163138));
#73678=CARTESIAN_POINT('Ctrl Pts',(3.25452173648234,7.44794060090072,8.78557262254887));
#73679=CARTESIAN_POINT('Ctrl Pts',(3.44586247288917,7.3613688384916,8.77735227346638));
#73680=CARTESIAN_POINT('Ctrl Pts',(3.63354911586303,7.26753110658021,8.76913192438387));
#73681=CARTESIAN_POINT('Ctrl Pts',(3.82127588874745,7.17367331090867,8.76090981768097));
#73682=CARTESIAN_POINT('Ctrl Pts',(4.00534674328393,7.07254657403411,8.75268771097805));
#73683=CARTESIAN_POINT('Ctrl Pts',(4.18520293643357,6.96446436873417,8.74446560427515));
#73684=CARTESIAN_POINT('Ctrl Pts',(4.26407963575847,6.91706445739098,8.74085976437125));
#73685=CARTESIAN_POINT('Ctrl Pts',(4.342146063272,6.86832738927524,8.73725392446735));
#73686=CARTESIAN_POINT('Ctrl Pts',(4.41935673691357,6.81828230527284,8.73364808456345));
#73687=CARTESIAN_POINT('Ctrl Pts',(4.59997103006115,6.70121484495554,8.72521315976963));
#73688=CARTESIAN_POINT('Ctrl Pts',(4.77596165233416,6.57694690403634,8.71677823497582));
#73689=CARTESIAN_POINT('Ctrl Pts',(4.94675954817621,6.44587135576157,8.708343310182));
#73690=CARTESIAN_POINT('',(-8.12524999914414,0.000117932813409655,9.58329744318989));
#73691=CARTESIAN_POINT('Ctrl Pts',(-8.12524999914414,0.000117932813416063,
9.58329744318989));
#73692=CARTESIAN_POINT('Ctrl Pts',(-8.12524687827972,0.215137000972684,
9.57487617318252));
#73693=CARTESIAN_POINT('Ctrl Pts',(-8.11670432117231,0.430123072685182,
9.56645490317514));
#73694=CARTESIAN_POINT('Ctrl Pts',(-8.09965616022477,0.644404879429754,
9.55803363316777));
#73695=CARTESIAN_POINT('Ctrl Pts',(-8.08260242067832,0.858756804720182,
9.54960960750319));
#73696=CARTESIAN_POINT('Ctrl Pts',(-8.05703753698575,1.07240374231327,9.5411855818386));
#73697=CARTESIAN_POINT('Ctrl Pts',(-8.0230472757909,1.2846789376822,9.53276155617401));
#73698=CARTESIAN_POINT('Ctrl Pts',(-8.00537532901957,1.39504337212792,9.52838180362397));
#73699=CARTESIAN_POINT('Ctrl Pts',(-7.98542678141814,1.50503712219184,9.52400205107392));
#73700=CARTESIAN_POINT('Ctrl Pts',(-7.96321917898033,1.614567394078,9.51962229852387));
#73701=CARTESIAN_POINT('Ctrl Pts',(-7.92152859063276,1.82018983754495,9.5114001385163));
#73702=CARTESIAN_POINT('Ctrl Pts',(-7.87186263879791,2.02423057697928,9.50317797850873));
#73703=CARTESIAN_POINT('Ctrl Pts',(-7.81436618878319,2.22606572906147,9.49495581850116));
#73704=CARTESIAN_POINT('Ctrl Pts',(-7.75688033704689,2.42786367701829,9.48673517407831));
#73705=CARTESIAN_POINT('Ctrl Pts',(-7.69156694875712,2.62745656534174,9.47851452965545));
#73706=CARTESIAN_POINT('Ctrl Pts',(-7.61862114646925,2.82423430137648,9.4702938852326));
#73707=CARTESIAN_POINT('Ctrl Pts',(-7.5456835391503,3.02098993075972,9.4620741643437));
#73708=CARTESIAN_POINT('Ctrl Pts',(-7.4651153322199,3.21493076262044,9.4538544434548));
#73709=CARTESIAN_POINT('Ctrl Pts',(-7.37716060335633,3.40546457840736,9.4456347225659));
#73710=CARTESIAN_POINT('Ctrl Pts',(-7.28919882701457,3.59601366094492,9.43741434306201));
#73711=CARTESIAN_POINT('Ctrl Pts',(-7.19384946738251,3.78315491282193,9.42919396355811));
#73712=CARTESIAN_POINT('Ctrl Pts',(-7.09140402891963,3.9663177458598,9.42097358405421));
#73713=CARTESIAN_POINT('Ctrl Pts',(-6.98895896957954,4.1494799010617,9.41275323497171));
#73714=CARTESIAN_POINT('Ctrl Pts',(-6.87941803034309,4.32866341058893,9.40453288588921));
#73715=CARTESIAN_POINT('Ctrl Pts',(-6.76311806007029,4.50332340256072,9.39631253680671));
#73716=CARTESIAN_POINT('Ctrl Pts',(-6.64679322331064,4.6780207391714,9.38809043010379));
#73717=CARTESIAN_POINT('Ctrl Pts',(-6.52370663195679,4.84819238025677,9.37986832340088));
#73718=CARTESIAN_POINT('Ctrl Pts',(-6.39423836763975,5.01332257692478,9.37164621669796));
#73719=CARTESIAN_POINT('Ctrl Pts',(-6.33745950905437,5.08574112778933,9.36804037679409));
#73720=CARTESIAN_POINT('Ctrl Pts',(-6.27945380601907,5.15719046178532,9.36443453689022));
#73721=CARTESIAN_POINT('Ctrl Pts',(-6.22025579367882,5.22762904419442,9.36082869698635));
#73722=CARTESIAN_POINT('Ctrl Pts',(-6.08527045251885,5.38824551933327,9.35260653697878));
#73723=CARTESIAN_POINT('Ctrl Pts',(-5.94403846854405,5.54365741341841,9.34438437697121));
#73724=CARTESIAN_POINT('Ctrl Pts',(-5.79698553565942,5.69338618590514,9.33616221696363));
#73725=CARTESIAN_POINT('Ctrl Pts',(-5.64995970893422,5.84308735899689,9.32794157254079));
#73726=CARTESIAN_POINT('Ctrl Pts',(-5.49711528150511,5.98710729082194,9.31972092811796));
#73727=CARTESIAN_POINT('Ctrl Pts',(-5.33891548163119,6.12500359530496,9.31150028369512));
#73728=CARTESIAN_POINT('Ctrl Pts',(-5.18073345443798,6.26288440806808,9.30328056280625));
#73729=CARTESIAN_POINT('Ctrl Pts',(-5.01719747833007,6.39464277307387,9.29506084191737));
#73730=CARTESIAN_POINT('Ctrl Pts',(-4.84880521885444,6.51987542151765,9.2868411210285));
#73731=CARTESIAN_POINT('Ctrl Pts',(-4.68039946674644,6.64511810437804,9.2786207415246));
#73732=CARTESIAN_POINT('Ctrl Pts',(-4.50713688898706,6.76383384758233,9.2704003620207));
#73733=CARTESIAN_POINT('Ctrl Pts',(-4.32954644922633,6.87566106687143,9.2621799825168));
#73734=CARTESIAN_POINT('Ctrl Pts',(-4.15195666667983,6.98748787231822,9.2539596334343));
#73735=CARTESIAN_POINT('Ctrl Pts',(-3.97003930534624,7.09242604983562,9.24573928435181));
#73736=CARTESIAN_POINT('Ctrl Pts',(-3.7843508435604,7.19015829139691,9.23751893526931));
#73737=CARTESIAN_POINT('Ctrl Pts',(-3.59862267910182,7.28791142941651,9.22929682856641));
#73738=CARTESIAN_POINT('Ctrl Pts',(-3.40912206456737,7.37845541591847,9.22107472186351));
#73739=CARTESIAN_POINT('Ctrl Pts',(-3.21642950883962,7.46151920034826,9.21285261516061));
#73740=CARTESIAN_POINT('Ctrl Pts',(-3.13192336804865,7.49794717669194,9.20924677525668));
#73741=CARTESIAN_POINT('Ctrl Pts',(-3.04680360442628,7.53293710030239,9.20564093535275));
#73742=CARTESIAN_POINT('Ctrl Pts',(-2.96112041560347,7.56646902106896,9.20203509544882));
#73743=CARTESIAN_POINT('Ctrl Pts',(-2.76574266527916,7.64292965860399,9.19381293544125));
#73744=CARTESIAN_POINT('Ctrl Pts',(-2.56736959657649,7.71183144184668,9.18559077543368));
#73745=CARTESIAN_POINT('Ctrl Pts',(-2.3666039701597,7.77295781610349,9.17736861542611));
#73746=CARTESIAN_POINT('Ctrl Pts',(-2.16587535072395,7.83407292298046,9.16914797100329));
#73747=CARTESIAN_POINT('Ctrl Pts',(-1.96275533599007,7.88741539549,9.16092732658046));
#73748=CARTESIAN_POINT('Ctrl Pts',(-1.75786234917643,7.93281838465043,9.15270668215763));
#73749=CARTESIAN_POINT('Ctrl Pts',(-1.55299238070759,7.97821627309134,9.14448696126874));
#73750=CARTESIAN_POINT('Ctrl Pts',(-1.34635012585057,8.01567639506547,9.13626724037985));
#73751=CARTESIAN_POINT('Ctrl Pts',(-1.13856553327261,8.04508272729023,9.12804751949097));
#73752=CARTESIAN_POINT('Ctrl Pts',(-0.930764291704717,8.07449141573266,
9.11982713998708));
#73753=CARTESIAN_POINT('Ctrl Pts',(-0.721820821386084,8.09584498095052,
9.11160676048318));
#73754=CARTESIAN_POINT('Ctrl Pts',(-0.512372611573524,8.1090789778747,9.10338638097929));
#73755=CARTESIAN_POINT('Ctrl Pts',(-0.302925176871561,8.12231292582346,
9.09516603189678));
#73756=CARTESIAN_POINT('Ctrl Pts',(-0.0929733011369583,8.12742734963881,
9.08694568281426));
#73757=CARTESIAN_POINT('Ctrl Pts',(0.116842548040901,8.12440984819619,9.07872533373175));
#73758=CARTESIAN_POINT('Ctrl Pts',(0.326703258648862,8.12139170157148,9.07050322702884));
#73759=CARTESIAN_POINT('Ctrl Pts',(0.536427589422058,8.11023816032079,9.06228112032593));
#73760=CARTESIAN_POINT('Ctrl Pts',(0.745376101833266,8.09098894013061,9.05405901362302));
#73761=CARTESIAN_POINT('Ctrl Pts',(0.837011361644048,8.08254711265394,9.05045317371912));
#73762=CARTESIAN_POINT('Ctrl Pts',(0.928497453617433,8.07254891838278,9.04684733381522));
#73763=CARTESIAN_POINT('Ctrl Pts',(1.01978075318514,8.06100085460442,9.04324149391132));
#73764=CARTESIAN_POINT('Ctrl Pts',(1.22792806839248,8.03466856290712,9.03501933390375));
#73765=CARTESIAN_POINT('Ctrl Pts',(1.43508927608202,8.00026559575085,9.02679717389618));
#73766=CARTESIAN_POINT('Ctrl Pts',(1.64063147025403,7.95789016896514,9.01857501388861));
#73767=CARTESIAN_POINT('Ctrl Pts',(1.84613577698402,7.9155225532108,9.01035436946577));
#73768=CARTESIAN_POINT('Ctrl Pts',(2.05002137690645,7.86518547042578,9.00213372504293));
#73769=CARTESIAN_POINT('Ctrl Pts',(2.25166539097638,7.80702827774943,8.99391308062009));
#73770=CARTESIAN_POINT('Ctrl Pts',(2.45328675170146,7.74887761864139,8.9856933597312));
#73771=CARTESIAN_POINT('Ctrl Pts',(2.65266674585659,7.68290868533619,8.97747363884231));
#73772=CARTESIAN_POINT('Ctrl Pts',(2.84919669008664,7.60932098046201,8.96925391795342));
#73773=CARTESIAN_POINT('Ctrl Pts',(3.04574238151431,7.53572737928467,8.96103353844953));
#73774=CARTESIAN_POINT('Ctrl Pts',(3.2394372893541,7.4545138877133,8.95281315894564));
#73775=CARTESIAN_POINT('Ctrl Pts',(3.42969078517489,7.36592890819525,8.94459277944175));
#73776=CARTESIAN_POINT('Ctrl Pts',(3.61994357691957,7.27734425650596,8.93637243035924));
#73777=CARTESIAN_POINT('Ctrl Pts',(3.80675471568613,7.18138829844081,8.92815208127672));
#73778=CARTESIAN_POINT('Ctrl Pts',(3.98955585702429,7.07835656252094,8.9199317321942));
#73779=CARTESIAN_POINT('Ctrl Pts',(4.17239608368721,6.97530279704025,8.91170962549129));
#73780=CARTESIAN_POINT('Ctrl Pts',(4.35122434285274,6.86517037618022,8.90348751878839));
#73781=CARTESIAN_POINT('Ctrl Pts',(4.52549812791133,6.7483001012678,8.89526541208548));
#73782=CARTESIAN_POINT('Ctrl Pts',(4.60192663839813,6.69704614457698,8.89165957218159));
#73783=CARTESIAN_POINT('Ctrl Pts',(4.67747954967086,6.6444968675941,8.88805373227769));
#73784=CARTESIAN_POINT('Ctrl Pts',(4.75211288108001,6.59068363130665,8.8844478923738));
#73785=CARTESIAN_POINT('Ctrl Pts',(4.81770694146005,6.54338802485793,8.88127877643176));
#73786=CARTESIAN_POINT('Ctrl Pts',(4.88259905651463,6.49511008660576,8.87810966048971));
#73787=CARTESIAN_POINT('Ctrl Pts',(4.9467595481762,6.44587135576158,8.87494054454767));
#73788=CARTESIAN_POINT('Ctrl Pts',(4.94675954817619,6.44587135576158,10.8749423500932));
#73789=CARTESIAN_POINT('Ctrl Pts',(5.11325382428399,6.31809853737967,10.8667219683852));
#73790=CARTESIAN_POINT('Ctrl Pts',(5.27479679333856,6.18387015657815,10.8585015866772));
#73791=CARTESIAN_POINT('Ctrl Pts',(5.43089607779182,6.04359622697657,10.8502812049692));
#73792=CARTESIAN_POINT('Ctrl Pts',(5.58699470910173,5.90332288430262,10.8420608576566));
#73793=CARTESIAN_POINT('Ctrl Pts',(5.73764948361426,5.75700424267344,10.8338405103439));
#73794=CARTESIAN_POINT('Ctrl Pts',(5.88240309512541,5.6050888832345,10.8256201630313));
#73795=CARTESIAN_POINT('Ctrl Pts',(6.02718771561716,5.45314098063215,10.8173980547636));
#73796=CARTESIAN_POINT('Ctrl Pts',(6.16606844392976,5.29559417869845,10.809175946496));
#73797=CARTESIAN_POINT('Ctrl Pts',(6.29862590212076,5.13293281736996,10.8009538382284));
#73798=CARTESIAN_POINT('Ctrl Pts',(6.35764735912206,5.06050754100724,10.7972929290936));
#73799=CARTESIAN_POINT('Ctrl Pts',(6.41541575706434,4.98706875720691,10.7936320199588));
#73800=CARTESIAN_POINT('Ctrl Pts',(6.47189666834309,4.91266130287745,10.789971110824));
#73801=CARTESIAN_POINT('Ctrl Pts',(6.59874906287325,4.74554707722338,10.7817489508164));
#73802=CARTESIAN_POINT('Ctrl Pts',(6.71914621451919,4.57348936598663,10.7735267908089));
#73803=CARTESIAN_POINT('Ctrl Pts',(6.83271537167142,4.39700900752148,10.7653046308013));
#73804=CARTESIAN_POINT('Ctrl Pts',(6.94626359470415,4.22056117955148,10.7570839863785));
#73805=CARTESIAN_POINT('Ctrl Pts',(7.05298617559616,4.03969257949409,10.7488633419556));
#73806=CARTESIAN_POINT('Ctrl Pts',(7.15255391163893,3.85495267203096,10.7406426975328));
#73807=CARTESIAN_POINT('Ctrl Pts',(7.25211046191814,3.67023351885036,10.7324229766439));
#73808=CARTESIAN_POINT('Ctrl Pts',(7.34451363210237,3.48164418625025,10.724203255755));
#73809=CARTESIAN_POINT('Ctrl Pts',(7.42947997433496,3.28975909048913,10.7159835348662));
#73810=CARTESIAN_POINT('Ctrl Pts',(7.51445312459773,3.09785861970432,10.7077631553623));
#73811=CARTESIAN_POINT('Ctrl Pts',(7.59198813427315,2.90266212688007,10.6995427758584));
#73812=CARTESIAN_POINT('Ctrl Pts',(7.66184912124185,2.70476535134297,10.6913223963545));
#73813=CARTESIAN_POINT('Ctrl Pts',(7.73170984967406,2.50686930816796,10.683102047272));
#73814=CARTESIAN_POINT('Ctrl Pts',(7.79389651647753,2.30627328146959,10.6748816981895));
#73815=CARTESIAN_POINT('Ctrl Pts',(7.84822249773654,2.10359007140697,10.666661349107));
#73816=CARTESIAN_POINT('Ctrl Pts',(7.90256009461575,1.90086352496766,10.6584392424041));
#73817=CARTESIAN_POINT('Ctrl Pts',(7.94903357177258,1.69604918874693,10.6502171357012));
#73818=CARTESIAN_POINT('Ctrl Pts',(7.98750672664966,1.48977308816695,10.6419950289983));
#73819=CARTESIAN_POINT('Ctrl Pts',(8.00437929253806,1.39930982594273,10.6383891890944));
#73820=CARTESIAN_POINT('Ctrl Pts',(8.01971381833703,1.3085655631382,10.6347833491904));
#73821=CARTESIAN_POINT('Ctrl Pts',(8.03350192841366,1.21759366320376,10.6311775092865));
#73822=CARTESIAN_POINT('Ctrl Pts',(8.06494205062438,1.01015641213862,10.6229553492789));
#73823=CARTESIAN_POINT('Ctrl Pts',(8.08834854780176,0.801466532148104,10.6147331892714));
#73824=CARTESIAN_POINT('Ctrl Pts',(8.10364328115617,0.59215972023803,10.6065110292638));
#73825=CARTESIAN_POINT('Ctrl Pts',(8.1189351952436,0.38289148969915,10.5982903848409));
#73826=CARTESIAN_POINT('Ctrl Pts',(8.12611830829277,0.173006848417312,10.5900697404181));
#73827=CARTESIAN_POINT('Ctrl Pts',(8.12516641861186,-0.0368542041301155,
10.5818490959953));
#73828=CARTESIAN_POINT('Ctrl Pts',(8.12421463586934,-0.246691680203768,
10.5736293751064));
#73829=CARTESIAN_POINT('Ctrl Pts',(8.11512967629721,-0.456505277809638,
10.5654096542175));
#73830=CARTESIAN_POINT('Ctrl Pts',(8.09793745429763,-0.665654977284556,
10.5571899333286));
#73831=CARTESIAN_POINT('Ctrl Pts',(8.08074385475061,-0.874821435130248,
10.5489695538247));
#73832=CARTESIAN_POINT('Ctrl Pts',(8.05544171626132,-1.08332359416993,10.5407491743208));
#73833=CARTESIAN_POINT('Ctrl Pts',(8.022108923528,-1.29052546722349,10.5325287948169));
#73834=CARTESIAN_POINT('Ctrl Pts',(7.98877625415026,-1.49772657347944,10.5243084457344));
#73835=CARTESIAN_POINT('Ctrl Pts',(7.94741303949096,-1.70362711240172,10.5160880966519));
#73836=CARTESIAN_POINT('Ctrl Pts',(7.89814858156644,-1.90759968179911,10.5078677475694));
#73837=CARTESIAN_POINT('Ctrl Pts',(7.848873590243,-2.11161586325541,10.4996456408665));
#73838=CARTESIAN_POINT('Ctrl Pts',(7.79169404988503,-2.31370296468734,10.4914235341636));
#73839=CARTESIAN_POINT('Ctrl Pts',(7.72678986617589,-2.51324609349373,10.4832014274606));
#73840=CARTESIAN_POINT('Ctrl Pts',(7.69832586005151,-2.60075658227635,10.4795955875568));
#73841=CARTESIAN_POINT('Ctrl Pts',(7.66837682174596,-2.68777798204506,10.4759897476529));
#73842=CARTESIAN_POINT('Ctrl Pts',(7.63696092701891,-2.77425942580834,10.472383907749));
#73843=CARTESIAN_POINT('Ctrl Pts',(7.56532532474245,-2.97145738447055,10.4641617477414));
#73844=CARTESIAN_POINT('Ctrl Pts',(7.48603589155157,-3.16591179019283,10.4559395877339));
#73845=CARTESIAN_POINT('Ctrl Pts',(7.39932814761351,-3.35702703689356,10.4477174277263));
#73846=CARTESIAN_POINT('Ctrl Pts',(7.31263638645032,-3.548107055461,10.4394967833035));
#73847=CARTESIAN_POINT('Ctrl Pts',(7.21852916558492,-3.7358488748302,10.4312761388806));
#73848=CARTESIAN_POINT('Ctrl Pts',(7.11728967093991,-3.91967795902061,10.4230554944578));
#73849=CARTESIAN_POINT('Ctrl Pts',(7.01606154986932,-4.10348639125324,10.4148357735689));
#73850=CARTESIAN_POINT('Ctrl Pts',(6.90770289700708,-4.28338270744836,10.40661605268));
#73851=CARTESIAN_POINT('Ctrl Pts',(6.79254267244258,-4.45881728775093,10.3983963317911));
#73852=CARTESIAN_POINT('Ctrl Pts',(6.67737322052681,-4.6342659249599,10.3901759522872));
#73853=CARTESIAN_POINT('Ctrl Pts',(6.5554012676622,-4.80525186371131,10.3819555727833));
#73854=CARTESIAN_POINT('Ctrl Pts',(6.42699948116171,-4.97125388927653,10.3737351932794));
#73855=CARTESIAN_POINT('Ctrl Pts',(6.29859816984121,-5.13725530051354,10.3655148441969));
#73856=CARTESIAN_POINT('Ctrl Pts',(6.16376725517245,-5.29827260363649,10.3572944951144));
#73857=CARTESIAN_POINT('Ctrl Pts',(6.02292044805656,-5.45381672215725,10.3490741460319));
#73858=CARTESIAN_POINT('Ctrl Pts',(5.88204352601259,-5.60939409808753,10.340852039329));
#73859=CARTESIAN_POINT('Ctrl Pts',(5.73514833993392,-5.75949573268095,10.3326299326261));
#73860=CARTESIAN_POINT('Ctrl Pts',(5.58268705217846,-5.90366774471082,10.3244078259232));
#73861=CARTESIAN_POINT('Ctrl Pts',(5.51582450526036,-5.96689499446413,10.3208019860193));
#73862=CARTESIAN_POINT('Ctrl Pts',(5.44789190699709,-6.02898227984894,10.3171961461154));
#73863=CARTESIAN_POINT('Ctrl Pts',(5.3789295542444,-6.08989362903624,10.3135903062115));
#73864=CARTESIAN_POINT('Ctrl Pts',(5.22167922867744,-6.22878577972567,10.3053681462039));
#73865=CARTESIAN_POINT('Ctrl Pts',(5.05902046870411,-6.36160692986553,10.2971459861963));
#73866=CARTESIAN_POINT('Ctrl Pts',(4.89144504598925,-6.48794674181032,10.2889238261888));
#73867=CARTESIAN_POINT('Ctrl Pts',(4.72390051232906,-6.61426326563032,10.2807031817659));
#73868=CARTESIAN_POINT('Ctrl Pts',(4.55144136029741,-6.73410065812387,10.2724825373431));
#73869=CARTESIAN_POINT('Ctrl Pts',(4.37459113756181,-6.84708988853408,10.2642618929202));
#73870=CARTESIAN_POINT('Ctrl Pts',(4.19776078275603,-6.96006642536627,10.2560421720313));
#73871=CARTESIAN_POINT('Ctrl Pts',(4.01654059071647,-7.0661961772169,10.2478224511424));
#73872=CARTESIAN_POINT('Ctrl Pts',(3.83148238401016,-7.16515389252176,10.2396027302535));
#73873=CARTESIAN_POINT('Ctrl Pts',(3.64640934929288,-7.26411953693237,10.2313823507496));
#73874=CARTESIAN_POINT('Ctrl Pts',(3.45749794443206,-7.35591185496512,10.2231619712457));
#73875=CARTESIAN_POINT('Ctrl Pts',(3.26532478261787,-7.44025144914616,10.2149415917418));
#73876=CARTESIAN_POINT('Ctrl Pts',(3.07315233198413,-7.52459073120938,10.2067212426593));
#73877=CARTESIAN_POINT('Ctrl Pts',(2.87771841987778,-7.60147722842589,10.1985008935768));
#73878=CARTESIAN_POINT('Ctrl Pts',(2.67962032507399,-7.67067940119716,10.1902805444943));
#73879=CARTESIAN_POINT('Ctrl Pts',(2.48147987425246,-7.73989637031698,10.1820584377914));
#73880=CARTESIAN_POINT('Ctrl Pts',(2.28067438139625,-7.80142563521947,10.1738363310885));
#73881=CARTESIAN_POINT('Ctrl Pts',(2.07781805207946,-7.85508495848089,10.1656142243856));
#73882=CARTESIAN_POINT('Ctrl Pts',(1.98885454510534,-7.87861748317593,10.1620083844817));
#73883=CARTESIAN_POINT('Ctrl Pts',(1.89949678999567,-7.90063703164834,10.1584025445778));
#73884=CARTESIAN_POINT('Ctrl Pts',(1.80979738244314,-7.92113129527607,10.1547967046739));
#73885=CARTESIAN_POINT('Ctrl Pts',(1.60526171221374,-7.96786301916735,10.1465745446664));
#73886=CARTESIAN_POINT('Ctrl Pts',(1.39888129661992,-8.00667608629494,10.1383523846588));
#73887=CARTESIAN_POINT('Ctrl Pts',(1.19128429069491,-8.03744544623747,10.1301302246512));
#73888=CARTESIAN_POINT('Ctrl Pts',(0.983725550973688,-8.06820913448647,
10.1219095802284));
#73889=CARTESIAN_POINT('Ctrl Pts',(0.774950960306297,-8.0909320315456,10.1136889358055));
#73890=CARTESIAN_POINT('Ctrl Pts',(0.565596814653767,-8.10554056221752,
10.1054682913827));
#73891=CARTESIAN_POINT('Ctrl Pts',(0.356266188527402,-8.12014745171955,
10.0972485704938));
#73892=CARTESIAN_POINT('Ctrl Pts',(0.146356431712985,-8.12664177423147,
10.0890288496049));
#73893=CARTESIAN_POINT('Ctrl Pts',(-0.0634922761331844,-8.12500192574571,
10.080809128716));
#73894=CARTESIAN_POINT('Ctrl Pts',(-0.273357798358859,-8.12336194586511,
10.0725887492121));
#73895=CARTESIAN_POINT('Ctrl Pts',(-0.48316196667668,-8.11358649228104,
10.0643683697082));
#73896=CARTESIAN_POINT('Ctrl Pts',(-0.692264770060775,-8.09570608721887,
10.0561479902043));
#73897=CARTESIAN_POINT('Ctrl Pts',(-0.901366799612261,-8.07782574832722,
10.0479276411218));
#73898=CARTESIAN_POINT('Ctrl Pts',(-1.10976717557884,-8.05184054576274,
10.0397072920393));
#73899=CARTESIAN_POINT('Ctrl Pts',(-1.31683063653816,-8.017832914022,10.0314869429568));
#73900=CARTESIAN_POINT('Ctrl Pts',(-1.52393837043037,-7.98381801099548,
10.0232648362539));
#73901=CARTESIAN_POINT('Ctrl Pts',(-1.72970832694089,-7.9417772997943,10.015042729551));
#73902=CARTESIAN_POINT('Ctrl Pts',(-1.93351396837177,-7.89184460671973,
10.0068206228481));
#73903=CARTESIAN_POINT('Ctrl Pts',(-2.02289380021593,-7.86994641156086,
10.0032147829442));
#73904=CARTESIAN_POINT('Ctrl Pts',(-2.11189597997634,-7.84653101254412,
9.99960894304032));
#73905=CARTESIAN_POINT('Ctrl Pts',(-2.2004684331936,-7.82161276445072,9.99600310313642));
#73906=CARTESIAN_POINT('Ctrl Pts',(-2.40243438343677,-7.76479331921943,
9.98778094312886));
#73907=CARTESIAN_POINT('Ctrl Pts',(-2.60223173787426,-7.70013771404643,
9.97955878312129));
#73908=CARTESIAN_POINT('Ctrl Pts',(-2.79924906934294,-7.62783666646597,
9.97133662311373));
#73909=CARTESIAN_POINT('Ctrl Pts',(-2.99623008475156,-7.55554894608453,
9.96311597869088));
#73910=CARTESIAN_POINT('Ctrl Pts',(-3.19043182301468,-7.47561869765075,
9.95489533426804));
#73911=CARTESIAN_POINT('Ctrl Pts',(-3.38126033544734,-7.38828573529953,
9.94667468984519));
#73912=CARTESIAN_POINT('Ctrl Pts',(-3.57206740958418,-7.30096258421738,
9.93845496895628));
#73913=CARTESIAN_POINT('Ctrl Pts',(-3.75950174618789,-7.2062385023116,9.93023524806737));
#73914=CARTESIAN_POINT('Ctrl Pts',(-3.94299085072363,-7.10440079905475,
9.92201552717846));
#73915=CARTESIAN_POINT('Ctrl Pts',(-4.12649465754374,-7.00255493592989,
9.91379514767456));
#73916=CARTESIAN_POINT('Ctrl Pts',(-4.30605234126817,-6.8935944534058,9.90557476817066));
#73917=CARTESIAN_POINT('Ctrl Pts',(-4.4811164941428,-6.77785235369002,9.89735438866676));
#73918=CARTESIAN_POINT('Ctrl Pts',(-4.65617999915263,-6.66211068230426,
9.88913403958425));
#73919=CARTESIAN_POINT('Ctrl Pts',(-4.82674976184907,-6.53958760893002,
9.88091369050175));
#73920=CARTESIAN_POINT('Ctrl Pts',(-4.99230738156593,-6.41065944895393,
9.87269334141924));
#73921=CARTESIAN_POINT('Ctrl Pts',(-5.15790039971245,-6.28170372241576,
9.86447123471634));
#73922=CARTESIAN_POINT('Ctrl Pts',(-5.3184789009949,-6.14634035467356,9.85624912801343));
#73923=CARTESIAN_POINT('Ctrl Pts',(-5.47355673260854,-6.00498661592311,
9.84802702131052));
#73924=CARTESIAN_POINT('Ctrl Pts',(-5.54156677597637,-5.94299533191693,
9.84442118140665));
#73925=CARTESIAN_POINT('Ctrl Pts',(-5.60851931880421,-5.87985243111227,
9.84081534150277));
#73926=CARTESIAN_POINT('Ctrl Pts',(-5.67437550088683,-5.81559543275109,
9.83720950159889));
#73927=CARTESIAN_POINT('Ctrl Pts',(-5.8245430293976,-5.66907441789309,9.82898734159132));
#73928=CARTESIAN_POINT('Ctrl Pts',(-5.96905721080625,-5.51670978455476,
9.82076518158375));
#73929=CARTESIAN_POINT('Ctrl Pts',(-6.10747237968127,-5.35896153129787,
9.81254302157618));
#73930=CARTESIAN_POINT('Ctrl Pts',(-6.24586203458983,-5.20124235566068,
9.80432237715334));
#73931=CARTESIAN_POINT('Ctrl Pts',(-6.37815472620382,-5.03814176245311,
9.79610173273049));
#73932=CARTESIAN_POINT('Ctrl Pts',(-6.50394362663989,-4.87015450103899,
9.78788108830764));
#73933=CARTESIAN_POINT('Ctrl Pts',(-6.62971839554145,-4.7021861118606,9.77966136741874));
#73934=CARTESIAN_POINT('Ctrl Pts',(-6.74899065513564,-4.5293323866415,9.77144164652984));
#73935=CARTESIAN_POINT('Ctrl Pts',(-6.86139514013848,-4.3521195173598,9.76322192564094));
#73936=CARTESIAN_POINT('Ctrl Pts',(-6.97380863168544,-4.17489244868447,
9.75500154613706));
#73937=CARTESIAN_POINT('Ctrl Pts',(-7.07935308871106,-3.99330578582776,
9.74678116663316));
#73938=CARTESIAN_POINT('Ctrl Pts',(-7.17770713602157,-3.80791384251338,
9.73856078712928));
#73939=CARTESIAN_POINT('Ctrl Pts',(-7.27606081935097,-3.62252258528328,
9.73034043804673));
#73940=CARTESIAN_POINT('Ctrl Pts',(-7.36722401023294,-3.4333263377414,9.7221200889642));
#73941=CARTESIAN_POINT('Ctrl Pts',(-7.45092152763993,-3.24090357021801,
9.71389973988166));
#73942=CARTESIAN_POINT('Ctrl Pts',(-7.53463694069338,-3.04843966013836,
9.70567763317876));
#73943=CARTESIAN_POINT('Ctrl Pts',(-7.6108833735059,-2.85274812254923,9.69745552647585));
#73944=CARTESIAN_POINT('Ctrl Pts',(-7.67943355671181,-2.65442796296086,
9.68923341977295));
#73945=CARTESIAN_POINT('Ctrl Pts',(-7.70949653143982,-2.56745381253664,
9.6856275798691));
#73946=CARTESIAN_POINT('Ctrl Pts',(-7.7380799203174,-2.47997433612477,9.68202173996524));
#73947=CARTESIAN_POINT('Ctrl Pts',(-7.76516754947262,-2.39204107220535,
9.67841590006139));
#73948=CARTESIAN_POINT('Ctrl Pts',(-7.82718015449563,-2.19073254377822,
9.67016093154966));
#73949=CARTESIAN_POINT('Ctrl Pts',(-7.88136995031025,-1.98698011876507,
9.66190596303793));
#73950=CARTESIAN_POINT('Ctrl Pts',(-7.92756461528397,-1.78140585858405,
9.6536509945262));
#73951=CARTESIAN_POINT('Ctrl Pts',(-7.97374954254046,-1.57587493293127,
9.64539776614071));
#73952=CARTESIAN_POINT('Ctrl Pts',(-8.01194263992958,-1.36852322183758,
9.63714453775523));
#73953=CARTESIAN_POINT('Ctrl Pts',(-8.0420223270444,-1.15998467826921,9.62889130936975));
#73954=CARTESIAN_POINT('Ctrl Pts',(-8.07209976663542,-0.951461716489887,
9.62063869765714));
#73955=CARTESIAN_POINT('Ctrl Pts',(-8.09406496248538,-0.741752386149109,
9.61238608594453));
#73956=CARTESIAN_POINT('Ctrl Pts',(-8.10784785788655,-0.531498519155556,
9.60413347423193));
#73957=CARTESIAN_POINT('Ctrl Pts',(-8.11944745189462,-0.354550249233417,
9.59718813055875));
#73958=CARTESIAN_POINT('Ctrl Pts',(-8.12525257302793,-0.177216522463021,
9.59024278688558));
#73959=CARTESIAN_POINT('Ctrl Pts',(-8.12524999914415,0.000117932238638647,
9.5832974432124));
#73960=CARTESIAN_POINT('Origin',(0.,0.,24.4167025567876));
#73961=CARTESIAN_POINT('',(4.94675954817619,6.44587135576159,12.8749480452876));
#73962=CARTESIAN_POINT('',(4.94717300284007,6.4464104346866,12.7083501623644));
#73963=CARTESIAN_POINT('',(4.9467595481762,6.44587135576158,24.4167025567876));
#73964=CARTESIAN_POINT('',(-8.12524999887474,-0.000135225956416249,11.4167025567876));
#73965=CARTESIAN_POINT('Ctrl Pts',(4.94717300284021,6.44641043468649,12.7083501623644));
#73966=CARTESIAN_POINT('Ctrl Pts',(4.97999127047003,6.42124041604394,12.7067294825768));
#73967=CARTESIAN_POINT('Ctrl Pts',(6.0780585597953,5.56544170535072,12.6521776022766));
#73968=CARTESIAN_POINT('Ctrl Pts',(7.79448477834709,3.31475408317713,12.5446945214639));
#73969=CARTESIAN_POINT('Ctrl Pts',(8.43041607796892,-0.818335105043671,
12.3859009199263));
#73970=CARTESIAN_POINT('Ctrl Pts',(7.01145427209639,-4.75195713176425,12.2271073183889));
#73971=CARTESIAN_POINT('Ctrl Pts',(3.88346779769395,-7.52730133953051,12.0683137168513));
#73972=CARTESIAN_POINT('Ctrl Pts',(-0.191104364661067,-8.46788442963361,
11.9095201153138));
#73973=CARTESIAN_POINT('Ctrl Pts',(-4.21909530993973,-7.34444159602813,
11.7507265137763));
#73974=CARTESIAN_POINT('Ctrl Pts',(-7.21869218977298,-4.43080925578325,
11.5919329122388));
#73975=CARTESIAN_POINT('Ctrl Pts',(-8.08818406800785,-1.63059466065753,
11.4805915932426));
#73976=CARTESIAN_POINT('Ctrl Pts',(-8.12586896382392,-0.139963263173689,
11.4221814747588));
#73977=CARTESIAN_POINT('Ctrl Pts',(-8.12575905226067,-0.000135234428430032,
11.4167025567876));
#73978=CARTESIAN_POINT('Ctrl Pts',(-8.12524999887474,-0.000135225956416249,
11.4167025567876));
#73979=CARTESIAN_POINT('Ctrl Pts',(-8.12525347870505,0.208955484150721,
11.4085091877829));
#73980=CARTESIAN_POINT('Ctrl Pts',(-8.11718167762833,0.418082135971698,
11.4003158187783));
#73981=CARTESIAN_POINT('Ctrl Pts',(-8.10105234256317,0.626608734021274,
11.3921224497736));
#73982=CARTESIAN_POINT('Ctrl Pts',(-8.08492580849104,0.835099119694661,
11.3839305036156));
#73983=CARTESIAN_POINT('Ctrl Pts',(-8.06074455612332,1.0429893613643,11.3757385574575));
#73984=CARTESIAN_POINT('Ctrl Pts',(-8.02857832661406,1.24964699652463,11.3675466112995));
#73985=CARTESIAN_POINT('Ctrl Pts',(-7.99641086333345,1.45631255826735,11.3593543509303));
#73986=CARTESIAN_POINT('Ctrl Pts',(-7.95625785296927,1.66174512272453,11.351162090561));
#73987=CARTESIAN_POINT('Ctrl Pts',(-7.90824060897219,1.86531982059464,11.3429698301918));
#73988=CARTESIAN_POINT('Ctrl Pts',(-7.86022522159834,2.0688866470943,11.3347778865826));
#73989=CARTESIAN_POINT('Ctrl Pts',(-7.80434627867582,2.27059545968444,11.3265859429733));
#73990=CARTESIAN_POINT('Ctrl Pts',(-7.74077579324093,2.46983353311014,11.3183939993641));
#73991=CARTESIAN_POINT('Ctrl Pts',(-7.67718969083417,2.66912055213322,11.3102000432902));
#73992=CARTESIAN_POINT('Ctrl Pts',(-7.60590836011643,2.86593533353154,11.3020060872164));
#73993=CARTESIAN_POINT('Ctrl Pts',(-7.52715345565799,3.05968109734919,11.2938121311425));
#73994=CARTESIAN_POINT('Ctrl Pts',(-7.46478731695495,3.21310868719226,11.2873233238162));
#73995=CARTESIAN_POINT('Ctrl Pts',(-7.39773542812496,3.36461194318915,11.28083451649));
#73996=CARTESIAN_POINT('Ctrl Pts',(-7.32612922650967,3.5139035443479,11.2743457091637));
#73997=CARTESIAN_POINT('Ctrl Pts',(-7.23539488695969,3.70307535525159,11.2661235491561));
#73998=CARTESIAN_POINT('Ctrl Pts',(-7.13731460211681,3.88876215565963,11.2579013891486));
#73999=CARTESIAN_POINT('Ctrl Pts',(-7.03218148356007,4.07039447041375,11.249679229141));
#74000=CARTESIAN_POINT('Ctrl Pts',(-6.92706774411427,4.25199330501598,11.2414585847182));
#74001=CARTESIAN_POINT('Ctrl Pts',(-6.81490391344161,4.42953889028286,11.2332379402953));
#74002=CARTESIAN_POINT('Ctrl Pts',(-6.6960284585416,4.60248741930936,11.2250172958725));
#74003=CARTESIAN_POINT('Ctrl Pts',(-6.57716635849726,4.77541651873498,11.2167975749836));
#74004=CARTESIAN_POINT('Ctrl Pts',(-6.45159430666074,4.94374934984069,11.2085778540948));
#74005=CARTESIAN_POINT('Ctrl Pts',(-6.31969386378421,5.10697141469856,11.2003581332059));
#74006=CARTESIAN_POINT('Ctrl Pts',(-6.18778285222611,5.27020655792062,11.192137753702));
#74007=CARTESIAN_POINT('Ctrl Pts',(-6.04954261984108,5.4283298853786,11.1839173741981));
#74008=CARTESIAN_POINT('Ctrl Pts',(-5.90539542017655,5.58085947626867,11.1756969946942));
#74009=CARTESIAN_POINT('Ctrl Pts',(-5.76124875396172,5.73338850268808,11.1674766456117));
#74010=CARTESIAN_POINT('Ctrl Pts',(-5.61119536885646,5.8803236212733,11.1592562965292));
#74011=CARTESIAN_POINT('Ctrl Pts',(-5.45569519238787,6.02121894056808,11.1510359474468));
#74012=CARTESIAN_POINT('Ctrl Pts',(-5.30016176790476,6.16214438516388,11.1428138407438));
#74013=CARTESIAN_POINT('Ctrl Pts',(-5.13917944418118,6.29702725230902,11.1345917340409));
#74014=CARTESIAN_POINT('Ctrl Pts',(-4.97324294174114,6.42546046637297,11.126369627338));
#74015=CARTESIAN_POINT('Ctrl Pts',(-4.90047078204565,6.48178539926375,11.1227637874341));
#74016=CARTESIAN_POINT('Ctrl Pts',(-4.8267462124903,6.53687039501838,11.1191579475301));
#74017=CARTESIAN_POINT('Ctrl Pts',(-4.75211288108026,6.59068363130647,11.1155521076262));
#74018=CARTESIAN_POINT('Ctrl Pts',(-4.58193139518513,6.71339042114571,11.1073299476186));
#74019=CARTESIAN_POINT('Ctrl Pts',(-4.40696657212852,6.8295224185167,11.0991077876111));
#74020=CARTESIAN_POINT('Ctrl Pts',(-4.22774825431306,6.93871978542533,11.0908856276035));
#74021=CARTESIAN_POINT('Ctrl Pts',(-4.04856297167875,7.04789702406336,11.0826649831806));
#74022=CARTESIAN_POINT('Ctrl Pts',(-3.8651260110447,7.15014202996808,11.0744443387578));
#74023=CARTESIAN_POINT('Ctrl Pts',(-3.67799476216117,7.24513920446081,11.0662236943349));
#74024=CARTESIAN_POINT('Ctrl Pts',(-3.49088453621112,7.34012570666181,11.0580039734461));
#74025=CARTESIAN_POINT('Ctrl Pts',(-3.30008111365677,7.42786586948591,11.0497842525571));
#74026=CARTESIAN_POINT('Ctrl Pts',(-3.10616570373832,7.50809044853749,11.0415645316683));
#74027=CARTESIAN_POINT('Ctrl Pts',(-2.91223475611538,7.58832145567955,11.0333441521644));
#74028=CARTESIAN_POINT('Ctrl Pts',(-2.71519159458971,7.66103556044727,11.0251237726605));
#74029=CARTESIAN_POINT('Ctrl Pts',(-2.51563757597134,7.72601159388601,11.0169033931566));
#74030=CARTESIAN_POINT('Ctrl Pts',(-2.3160842958477,7.79098738686626,11.0086830440741));
#74031=CARTESIAN_POINT('Ctrl Pts',(-2.11402045868706,7.84822507696063,11.0004626949916));
#74032=CARTESIAN_POINT('Ctrl Pts',(-1.91006326632435,7.89755315785455,10.9922423459091));
#74033=CARTESIAN_POINT('Ctrl Pts',(-1.70606246519036,7.94689178575087,10.9840202392062));
#74034=CARTESIAN_POINT('Ctrl Pts',(-1.50016778702453,7.98831735640183,10.9757981325032));
#74035=CARTESIAN_POINT('Ctrl Pts',(-1.29300841568809,8.02170909466678,10.9675760258003));
#74036=CARTESIAN_POINT('Ctrl Pts',(-1.20215779131438,8.03635318366321,10.9639701858964));
#74037=CARTESIAN_POINT('Ctrl Pts',(-1.11106405275177,8.0494527908262,10.9603643459926));
#74038=CARTESIAN_POINT('Ctrl Pts',(-1.01978075318463,8.06100085460448,10.9567585060887));
#74039=CARTESIAN_POINT('Ctrl Pts',(-0.811633437977397,8.08733314630175,
10.9485363460811));
#74040=CARTESIAN_POINT('Ctrl Pts',(-0.602431320363802,8.1056034529901,10.9403141860736));
#74041=CARTESIAN_POINT('Ctrl Pts',(-0.392811825792572,8.11574928346222,
10.932092026066));
#74042=CARTESIAN_POINT('Ctrl Pts',(-0.183230970229024,8.12589324376085,
10.9238713816432));
#74043=CARTESIAN_POINT('Ctrl Pts',(0.0267668140914816,8.12791570254229,
10.9156507372203));
#74044=CARTESIAN_POINT('Ctrl Pts',(0.236541077043419,8.12180619575296,10.9074300927975));
#74045=CARTESIAN_POINT('Ctrl Pts',(0.446291773272173,8.11569737532549,10.8992103719086));
#74046=CARTESIAN_POINT('Ctrl Pts',(0.655818703362964,8.1014584217971,10.8909906510197));
#74047=CARTESIAN_POINT('Ctrl Pts',(0.864482677904975,8.07913097196117,10.8827709301308));
#74048=CARTESIAN_POINT('Ctrl Pts',(1.07316337189805,8.05680173311156,10.8745505506269));
#74049=CARTESIAN_POINT('Ctrl Pts',(1.2809806784145,8.0263827316729,10.866330171123));
#74050=CARTESIAN_POINT('Ctrl Pts',(1.48730071661944,7.98796745992642,10.8581097916191));
#74051=CARTESIAN_POINT('Ctrl Pts',(1.69361999129065,7.94955233034429,10.8498894425366));
#74052=CARTESIAN_POINT('Ctrl Pts',(1.89844171906582,7.90314104629872,10.8416690934541));
#74053=CARTESIAN_POINT('Ctrl Pts',(2.10114186522571,7.8488782908576,10.8334487443715));
#74054=CARTESIAN_POINT('Ctrl Pts',(2.30388535138336,7.79460393331484,10.8252266376686));
#74055=CARTESIAN_POINT('Ctrl Pts',(2.50450606451344,7.73247482689936,10.8170045309657));
#74056=CARTESIAN_POINT('Ctrl Pts',(2.70239371943027,7.66268593560273,10.8087824242628));
#74057=CARTESIAN_POINT('Ctrl Pts',(2.78917819308923,7.63207972016717,10.8051765843589));
#74058=CARTESIAN_POINT('Ctrl Pts',(2.87543722678284,7.60000094183469,10.801570744455));
#74059=CARTESIAN_POINT('Ctrl Pts',(2.96112041560399,7.56646902106876,10.7979649045512));
#74060=CARTESIAN_POINT('Ctrl Pts',(3.15650058942059,7.49000743510553,10.7897426425548));
#74061=CARTESIAN_POINT('Ctrl Pts',(3.34894985265458,7.40596157228609,10.7815203805584));
#74062=CARTESIAN_POINT('Ctrl Pts',(3.5378785458744,7.31458152987179,10.7732981185621));
#74063=CARTESIAN_POINT('Ctrl Pts',(3.72676958833246,7.22321969818107,10.7650774951439));
#74064=CARTESIAN_POINT('Ctrl Pts',(3.91214119575806,7.12452673301637,10.7568568717256));
#74065=CARTESIAN_POINT('Ctrl Pts',(4.09342597040225,7.01879985377389,10.7486362483074));
#74066=CARTESIAN_POINT('Ctrl Pts',(4.27470096158518,6.9130786803323,10.7404160685346));
#74067=CARTESIAN_POINT('Ctrl Pts',(4.45188930434596,6.80032449748332,10.7321958887617));
#74068=CARTESIAN_POINT('Ctrl Pts',(4.6244495403283,6.6808797333478,10.7239757089889));
#74069=CARTESIAN_POINT('Ctrl Pts',(4.7337876516959,6.60519679950745,10.718767215118));
#74070=CARTESIAN_POINT('Ctrl Pts',(4.84126821146589,6.52682864583457,10.7135587212472));
#74071=CARTESIAN_POINT('Ctrl Pts',(4.9467595481762,6.44587135576158,10.7083502273763));
#74072=CARTESIAN_POINT('',(-8.12524999999793,-5.8050124092788E-6,11.5832974432392));
#74073=CARTESIAN_POINT('Ctrl Pts',(-8.12524999999793,-5.80432776886074E-6,
11.5832974432124));
#74074=CARTESIAN_POINT('Ctrl Pts',(-8.1252501498455,0.209759912077751,11.575076876068));
#74075=CARTESIAN_POINT('Ctrl Pts',(-8.11712282336244,0.419560513241832,
11.5668563089237));
#74076=CARTESIAN_POINT('Ctrl Pts',(-8.10088596652066,0.628756009854853,
11.5586357417793));
#74077=CARTESIAN_POINT('Ctrl Pts',(-8.0846521127155,0.837912815374886,11.550416695044));
#74078=CARTESIAN_POINT('Ctrl Pts',(-8.06031174491846,1.04646444536909,11.5421976483087));
#74079=CARTESIAN_POINT('Ctrl Pts',(-8.02793480465863,1.25377443531546,11.5339786015733));
#74080=CARTESIAN_POINT('Ctrl Pts',(-7.99556150104078,1.46106113979361,11.5257604780176));
#74081=CARTESIAN_POINT('Ctrl Pts',(-7.95515347266073,1.66710619092948,11.5175423544619));
#74082=CARTESIAN_POINT('Ctrl Pts',(-7.90683219188853,1.87128091205336,11.5093242309062));
#74083=CARTESIAN_POINT('Ctrl Pts',(-7.85850705403901,2.0754719307106,11.5011054513675));
#74084=CARTESIAN_POINT('Ctrl Pts',(-7.80226746711589,2.27779203299136,11.4928866718287));
#74085=CARTESIAN_POINT('Ctrl Pts',(-7.73828568192483,2.47762431926577,11.48466789229));
#74086=CARTESIAN_POINT('Ctrl Pts',(-7.67430403741296,2.67745616616131,11.4764491308223));
#74087=CARTESIAN_POINT('Ctrl Pts',(-7.60258032135703,2.87479992751923,11.4682303693545));
#74088=CARTESIAN_POINT('Ctrl Pts',(-7.52333633373635,3.06905489882188,11.4600116078867));
#74089=CARTESIAN_POINT('Ctrl Pts',(-7.44407546709598,3.26335124655675,11.4517910958176));
#74090=CARTESIAN_POINT('Ctrl Pts',(-7.35729124047569,3.45455721635805,11.4435705837484));
#74091=CARTESIAN_POINT('Ctrl Pts',(-7.26325360681933,3.64209206439458,11.4353500716792));
#74092=CARTESIAN_POINT('Ctrl Pts',(-7.22434231723412,3.71969102659236,11.4319485534442));
#74093=CARTESIAN_POINT('Ctrl Pts',(-7.18418967585113,3.79666169270989,11.4285470352091));
#74094=CARTESIAN_POINT('Ctrl Pts',(-7.14281713462595,3.87296410308615,11.4251455169741));
#74095=CARTESIAN_POINT('Ctrl Pts',(-7.04281130476781,4.05740251667848,11.4169233569665));
#74096=CARTESIAN_POINT('Ctrl Pts',(-6.93564143296636,4.23799584074839,11.408701196959));
#74097=CARTESIAN_POINT('Ctrl Pts',(-6.82162851674016,4.41418983983442,11.4004790369514));
#74098=CARTESIAN_POINT('Ctrl Pts',(-6.70763661643125,4.59035136120973,11.3922583925285));
#74099=CARTESIAN_POINT('Ctrl Pts',(-6.58680434948576,4.76211492842893,11.3840377481057));
#74100=CARTESIAN_POINT('Ctrl Pts',(-6.45949673983474,4.92895419237837,11.3758171036829));
#74101=CARTESIAN_POINT('Ctrl Pts',(-6.33220343233532,5.09577471306139,11.367597382794));
#74102=CARTESIAN_POINT('Ctrl Pts',(-6.19843641342503,5.25767180038029,11.3593776619051));
#74103=CARTESIAN_POINT('Ctrl Pts',(-6.05860229397876,5.41415051562988,11.3511579410163));
#74104=CARTESIAN_POINT('Ctrl Pts',(-5.91875697015549,5.57064176892473,11.3429375615124));
#74105=CARTESIAN_POINT('Ctrl Pts',(-5.7728437690881,5.72171356076734,11.3347171820085));
#74106=CARTESIAN_POINT('Ctrl Pts',(-5.62130832848872,5.86690550789454,11.3264968025046));
#74107=CARTESIAN_POINT('Ctrl Pts',(-5.46977344868068,6.01209691770594,11.3182764534221));
#74108=CARTESIAN_POINT('Ctrl Pts',(-5.31261658591901,6.15140832406688,11.3100561043396));
#74109=CARTESIAN_POINT('Ctrl Pts',(-5.15031921841847,6.28441719739303,11.3018357552571));
#74110=CARTESIAN_POINT('Ctrl Pts',(-4.98798714957372,6.41745450979228,11.2936136485542));
#74111=CARTESIAN_POINT('Ctrl Pts',(-4.82051260850807,6.54418640986268,11.2853915418513));
#74112=CARTESIAN_POINT('Ctrl Pts',(-4.64840989828935,6.66423086184637,11.2771694351484));
#74113=CARTESIAN_POINT('Ctrl Pts',(-4.57293352191708,6.71687686740787,11.2735635952444));
#74114=CARTESIAN_POINT('Ctrl Pts',(-4.49656741055537,6.76823722127028,11.2699577553405));
#74115=CARTESIAN_POINT('Ctrl Pts',(-4.41935673691317,6.81828230527309,11.2663519154366));
#74116=CARTESIAN_POINT('Ctrl Pts',(-4.24329830672989,6.93239682483752,11.258129755429));
#74117=CARTESIAN_POINT('Ctrl Pts',(-4.06278854574039,7.03970738493306,11.2499075954214));
#74118=CARTESIAN_POINT('Ctrl Pts',(-3.87837449260932,7.13988087138556,11.2416854354139));
#74119=CARTESIAN_POINT('Ctrl Pts',(-3.69399443238534,7.24003589293281,11.233464790991));
#74120=CARTESIAN_POINT('Ctrl Pts',(-3.50571177561206,7.3330563257284,11.2252441465682));
#74121=CARTESIAN_POINT('Ctrl Pts',(-3.31409888006422,7.41865460684463,11.2170235021453));
#74122=CARTESIAN_POINT('Ctrl Pts',(-3.12250751093267,7.50424327157139,11.2088037812564));
#74123=CARTESIAN_POINT('Ctrl Pts',(-2.92758691932108,7.58241132896441,11.2005840603675));
#74124=CARTESIAN_POINT('Ctrl Pts',(-2.72993095394003,7.65291869480005,11.1923643394786));
#74125=CARTESIAN_POINT('Ctrl Pts',(-2.5322591511377,7.72343171012293,11.1841439599747));
#74126=CARTESIAN_POINT('Ctrl Pts',(-2.33185181371052,7.78628270567305,11.1759235804709));
#74127=CARTESIAN_POINT('Ctrl Pts',(-2.12932052853281,7.84128061283798,11.167703200967));
#74128=CARTESIAN_POINT('Ctrl Pts',(-1.92678999286815,7.89627831647065,11.1594828518844));
#74129=CARTESIAN_POINT('Ctrl Pts',(-1.7221358107046,7.94342291508327,11.1512625028019));
#74130=CARTESIAN_POINT('Ctrl Pts',(-1.51598293110405,7.98257372750801,11.1430421537194));
#74131=CARTESIAN_POINT('Ctrl Pts',(-1.30978597326509,8.02173291089924,11.1348200470165));
#74132=CARTESIAN_POINT('Ctrl Pts',(-1.10208996782934,8.05289483841846,11.1265979403136));
#74133=CARTESIAN_POINT('Ctrl Pts',(-0.893529314802037,8.07597009195115,
11.1183758336107));
#74134=CARTESIAN_POINT('Ctrl Pts',(-0.802064152375844,8.08608984264121,
11.1147699937068));
#74135=CARTESIAN_POINT('Ctrl Pts',(-0.710432783381724,8.09465495381696,
11.1111641538029));
#74136=CARTESIAN_POINT('Ctrl Pts',(-0.618689045347654,8.10166102892899,
11.107558313899));
#74137=CARTESIAN_POINT('Ctrl Pts',(-0.40949182253276,8.11763652205449,11.0993361538915));
#74138=CARTESIAN_POINT('Ctrl Pts',(-0.19964098094302,8.12550763408714,11.0911139938839));
#74139=CARTESIAN_POINT('Ctrl Pts',(0.0102237389347411,8.12524356789765,
11.0828918338763));
#74140=CARTESIAN_POINT('Ctrl Pts',(0.22004977460258,8.12497955038329,11.0746711894535));
#74141=CARTESIAN_POINT('Ctrl Pts',(0.429889388458503,8.11658334791561,11.0664505450306));
#74142=CARTESIAN_POINT('Ctrl Pts',(0.639102399678589,8.1000762765066,11.0582299006078));
#74143=CARTESIAN_POINT('Ctrl Pts',(0.848291907227683,8.08357105955575,11.0500101797189));
#74144=CARTESIAN_POINT('Ctrl Pts',(1.0568546585658,8.05895681601877,11.04179045883));
#74145=CARTESIAN_POINT('Ctrl Pts',(1.26415431630378,8.02630683609034,11.0335707379411));
#74146=CARTESIAN_POINT('Ctrl Pts',(1.47147058417592,7.99365424004304,11.0253503584372));
#74147=CARTESIAN_POINT('Ctrl Pts',(1.67752326424249,7.9529646643056,11.0171299789334));
#74148=CARTESIAN_POINT('Ctrl Pts',(1.88168389325767,7.90436292741892,11.0089095994295));
#74149=CARTESIAN_POINT('Ctrl Pts',(2.08584376673018,7.85576137039399,11.0006892503469));
#74150=CARTESIAN_POINT('Ctrl Pts',(2.28811131665572,7.7992477817398,10.9924689012644));
#74151=CARTESIAN_POINT('Ctrl Pts',(2.48787045291621,7.73499761939243,10.9842485521819));
#74152=CARTESIAN_POINT('Ctrl Pts',(2.68767230034718,7.67073371950248,10.976026445479));
#74153=CARTESIAN_POINT('Ctrl Pts',(2.88496438160005,7.5987300315721,10.9678043387761));
#74154=CARTESIAN_POINT('Ctrl Pts',(3.07914683316719,7.51921155057473,10.9595822320732));
#74155=CARTESIAN_POINT('Ctrl Pts',(3.16430637412174,7.48433838214737,10.9559763921693));
#74156=CARTESIAN_POINT('Ctrl Pts',(3.24886808078214,7.44802052593385,10.9523705522654));
#74157=CARTESIAN_POINT('Ctrl Pts',(3.33278257356589,7.41027987864396,10.9487647123615));
#74158=CARTESIAN_POINT('Ctrl Pts',(3.52412638941611,7.3242227599563,10.9405425907271));
#74159=CARTESIAN_POINT('Ctrl Pts',(3.71216682489899,7.23073633081746,10.9323204690927));
#74160=CARTESIAN_POINT('Ctrl Pts',(3.89632738088859,7.13009961385098,10.9240983474582));
#74161=CARTESIAN_POINT('Ctrl Pts',(4.08046637411999,7.0294746801091,10.9158771885252));
#74162=CARTESIAN_POINT('Ctrl Pts',(4.26072613435067,6.92170126860998,10.9076560295922));
#74163=CARTESIAN_POINT('Ctrl Pts',(4.43655459726775,6.80710444080024,10.8994348706591));
#74164=CARTESIAN_POINT('Ctrl Pts',(4.61116429561427,6.69330194714617,10.8912706971372));
#74165=CARTESIAN_POINT('Ctrl Pts',(4.78140370353987,6.57277050688571,10.8831065236152));
#74166=CARTESIAN_POINT('Ctrl Pts',(4.94675954817619,6.44587135576158,10.8749423500932));
#74167=CARTESIAN_POINT('Ctrl Pts',(4.94675954817619,6.44587135576158,12.8749480452876));
#74168=CARTESIAN_POINT('Ctrl Pts',(5.08620153897348,6.33885929155453,12.8680613404623));
#74169=CARTESIAN_POINT('Ctrl Pts',(5.22215542942478,6.22733177311037,12.861174635637));
#74170=CARTESIAN_POINT('Ctrl Pts',(5.35433288438807,6.11153065325378,12.8542879308117));
#74171=CARTESIAN_POINT('Ctrl Pts',(5.51214191086351,5.97327362602921,12.8460657708041));
#74172=CARTESIAN_POINT('Ctrl Pts',(5.66461910540582,5.8288782131343,12.8378436107966));
#74173=CARTESIAN_POINT('Ctrl Pts',(5.81129477521856,5.67877985116675,12.829621450789));
#74174=CARTESIAN_POINT('Ctrl Pts',(5.95794340841248,5.52870915672035,12.8214008063662));
#74175=CARTESIAN_POINT('Ctrl Pts',(6.09879244506011,5.37293782227638,12.8131801619433));
#74176=CARTESIAN_POINT('Ctrl Pts',(6.23340911041919,5.21193806799764,12.8049595175205));
#74177=CARTESIAN_POINT('Ctrl Pts',(6.36801065250421,5.05095640095501,12.7967397966316));
#74178=CARTESIAN_POINT('Ctrl Pts',(6.49638103188557,4.88474771307027,12.7885200757427));
#74179=CARTESIAN_POINT('Ctrl Pts',(6.61812729041575,4.71381785078234,12.7803003548538));
#74180=CARTESIAN_POINT('Ctrl Pts',(6.73988330401075,4.54287429253442,12.7720799753499));
#74181=CARTESIAN_POINT('Ctrl Pts',(6.85501396277648,4.36720904284507,12.763859595846));
#74182=CARTESIAN_POINT('Ctrl Pts',(6.96316862739231,4.1873583831575,12.7556392163421));
#74183=CARTESIAN_POINT('Ctrl Pts',(7.071322891757,4.00750838904856,12.7474188672596));
#74184=CARTESIAN_POINT('Ctrl Pts',(7.17250106379876,3.82347327023304,12.7391985181771));
#74185=CARTESIAN_POINT('Ctrl Pts',(7.26639733642572,3.63581590728755,12.7309781690946));
#74186=CARTESIAN_POINT('Ctrl Pts',(7.36031368533006,3.44811842069108,12.7227560623917));
#74187=CARTESIAN_POINT('Ctrl Pts',(7.44694489220615,3.25679740669599,12.7145339556888));
#74188=CARTESIAN_POINT('Ctrl Pts',(7.52603189142397,3.06243882090227,12.7063118489859));
#74189=CARTESIAN_POINT('Ctrl Pts',(7.56071583167937,2.97720203553345,12.702706009082));
#74190=CARTESIAN_POINT('Ctrl Pts',(7.59394941469675,2.8913813045124,12.6991001691781));
#74191=CARTESIAN_POINT('Ctrl Pts',(7.62571372598674,2.80502722478721,12.6954943292742));
#74192=CARTESIAN_POINT('Ctrl Pts',(7.69814379967779,2.60811968597999,12.6872721692666));
#74193=CARTESIAN_POINT('Ctrl Pts',(7.76295507009928,2.40837277274515,12.6790500092591));
#74194=CARTESIAN_POINT('Ctrl Pts',(7.81994341318432,2.20639356804157,12.6708278492515));
#74195=CARTESIAN_POINT('Ctrl Pts',(7.87692125164993,2.00445159401645,12.6626072048287));
#74196=CARTESIAN_POINT('Ctrl Pts',(7.92607896069587,1.80027843368315,12.6543865604058));
#74197=CARTESIAN_POINT('Ctrl Pts',(7.96726243329179,1.59449580794602,12.646165915983));
#74198=CARTESIAN_POINT('Ctrl Pts',(8.00844127920236,1.38873630049881,12.6379461950941));
#74199=CARTESIAN_POINT('Ctrl Pts',(8.04164761927169,1.18136797791785,12.6297264742052));
#74200=CARTESIAN_POINT('Ctrl Pts',(8.06677839825177,0.973023039808759,12.6215067533163));
#74201=CARTESIAN_POINT('Ctrl Pts',(8.0919111908656,0.764661407811974,12.6132863738124));
#74202=CARTESIAN_POINT('Ctrl Pts',(8.10896709143555,0.555323296633125,12.6050659943085));
#74203=CARTESIAN_POINT('Ctrl Pts',(8.11789476697463,0.345647385099121,12.5968456148046));
#74204=CARTESIAN_POINT('Ctrl Pts',(8.12682240947486,0.135972249517645,12.5886252657221));
#74205=CARTESIAN_POINT('Ctrl Pts',(8.1276218772276,-0.0740403889280623,
12.5804049166396));
#74206=CARTESIAN_POINT('Ctrl Pts',(8.12029393139912,-0.283749943053032,
12.5721845675571));
#74207=CARTESIAN_POINT('Ctrl Pts',(8.112964418758,-0.493504335880073,12.5639624608542));
#74208=CARTESIAN_POINT('Ctrl Pts',(8.09750403115892,-0.702955219897917,
12.5557403541513));
#74209=CARTESIAN_POINT('Ctrl Pts',(8.07396561443259,-0.911464107609391,
12.5475182474484));
#74210=CARTESIAN_POINT('Ctrl Pts',(8.06364274155181,-1.00290656813609,12.5439124075445));
#74211=CARTESIAN_POINT('Ctrl Pts',(8.05176689539146,-1.09416791368378,12.5403065676406));
#74212=CARTESIAN_POINT('Ctrl Pts',(8.03834567368995,-1.18519466450457,12.5367007277367));
#74213=CARTESIAN_POINT('Ctrl Pts',(8.00774214295416,-1.39275698844776,12.5284785677291));
#74214=CARTESIAN_POINT('Ctrl Pts',(7.96908990209952,-1.59916758506913,12.5202564077215));
#74215=CARTESIAN_POINT('Ctrl Pts',(7.92250015052607,-1.80379570002106,12.512034247714));
#74216=CARTESIAN_POINT('Ctrl Pts',(7.8759189868075,-2.00838609602195,12.5038136032911));
#74217=CARTESIAN_POINT('Ctrl Pts',(7.82140329803518,-2.21119437848746,12.4955929588683));
#74218=CARTESIAN_POINT('Ctrl Pts',(7.75911520809883,-2.41160086870723,12.4873723144455));
#74219=CARTESIAN_POINT('Ctrl Pts',(7.69683411580874,-2.6119848446112,12.4791525935565));
#74220=CARTESIAN_POINT('Ctrl Pts',(7.62678245315554,-2.80996728522362,12.4709328726676));
#74221=CARTESIAN_POINT('Ctrl Pts',(7.54917218725299,-3.00494373486524,12.4627131517786));
#74222=CARTESIAN_POINT('Ctrl Pts',(7.47155570273525,-3.19993580722762,12.4544927722747));
#74223=CARTESIAN_POINT('Ctrl Pts',(7.38637951145395,-3.39192113212285,12.4462723927708));
#74224=CARTESIAN_POINT('Ctrl Pts',(7.29390409904462,-3.58031430972758,12.438052013267));
#74225=CARTESIAN_POINT('Ctrl Pts',(7.20142902886164,-3.7687067901404,12.4298316641844));
#74226=CARTESIAN_POINT('Ctrl Pts',(7.10165492403412,-3.95350688608519,12.4216113151019));
#74227=CARTESIAN_POINT('Ctrl Pts',(6.99488892845406,-4.1341524453134,12.4133909660194));
#74228=CARTESIAN_POINT('Ctrl Pts',(6.88810010487836,-4.31483662897457,12.4051688593165));
#74229=CARTESIAN_POINT('Ctrl Pts',(6.77431655411192,-4.49136424714162,12.3969467526136));
#74230=CARTESIAN_POINT('Ctrl Pts',(6.65389015240542,-4.66319991017135,12.3887246459107));
#74231=CARTESIAN_POINT('Ctrl Pts',(6.60107664116816,-4.73855917185967,12.3851188060069));
#74232=CARTESIAN_POINT('Ctrl Pts',(6.54698607401266,-4.81301640426677,12.381512966103));
#74233=CARTESIAN_POINT('Ctrl Pts',(6.49165070897511,-4.88652828040143,12.3779071261992));
#74234=CARTESIAN_POINT('Ctrl Pts',(6.3654731088736,-5.0541525854609,12.3696849661916));
#74235=CARTESIAN_POINT('Ctrl Pts',(6.23277874502435,-5.21691479214037,12.3614628061841));
#74236=CARTESIAN_POINT('Ctrl Pts',(6.09396703571509,-5.37431421951842,12.3532406461765));
#74237=CARTESIAN_POINT('Ctrl Pts',(5.95518091346581,-5.53168463357612,12.3450200017536));
#74238=CARTESIAN_POINT('Ctrl Pts',(5.81027989142122,-5.6836940200293,12.3367993573307));
#74239=CARTESIAN_POINT('Ctrl Pts',(5.65970280709325,-5.82987578751732,12.3285787129079));
#74240=CARTESIAN_POINT('Ctrl Pts',(5.50914263908526,-5.97604113246958,12.320358992019));
#74241=CARTESIAN_POINT('Ctrl Pts',(5.35290789353397,-6.11637996000327,12.31213927113));
#74242=CARTESIAN_POINT('Ctrl Pts',(5.19147389345428,-6.25046289294502,12.3039195502411));
#74243=CARTESIAN_POINT('Ctrl Pts',(5.03002695828155,-6.38455656944272,12.2956991707372));
#74244=CARTESIAN_POINT('Ctrl Pts',(4.86338016148537,-6.5123931590959,12.2874787912333));
#74245=CARTESIAN_POINT('Ctrl Pts',(4.69204231459319,-6.63358323084643,12.2792584117294));
#74246=CARTESIAN_POINT('Ctrl Pts',(4.52070510177493,-6.75477285410607,12.2710380626468));
#74247=CARTESIAN_POINT('Ctrl Pts',(4.34467711608927,-6.86931584041031,12.2628177135642));
#74248=CARTESIAN_POINT('Ctrl Pts',(4.16449701858858,-6.97686549566973,12.2545973644817));
#74249=CARTESIAN_POINT('Ctrl Pts',(3.98427839617798,-7.08443814648103,12.2463752577787));
#74250=CARTESIAN_POINT('Ctrl Pts',(3.79990614182762,-7.1850143276905,12.2381531510758));
#74251=CARTESIAN_POINT('Ctrl Pts',(3.6119453932408,-7.27829224741262,12.2299310443729));
#74252=CARTESIAN_POINT('Ctrl Pts',(3.52951440662434,-7.3191996762776,12.2263252044691));
#74253=CARTESIAN_POINT('Ctrl Pts',(3.44639356067816,-7.35870402896952,12.2227193645654));
#74254=CARTESIAN_POINT('Ctrl Pts',(3.36263191091955,-7.39678269210104,12.2191135246617));
#74255=CARTESIAN_POINT('Ctrl Pts',(3.17163571996251,-7.4836109677596,12.2108913646541));
#74256=CARTESIAN_POINT('Ctrl Pts',(2.97724315670334,-7.56305189845629,12.2026692046466));
#74257=CARTESIAN_POINT('Ctrl Pts',(2.78004450109596,-7.6348569164344,12.194447044639));
#74258=CARTESIAN_POINT('Ctrl Pts',(2.58288219497156,-7.70664869864641,12.1862264002162));
#74259=CARTESIAN_POINT('Ctrl Pts',(2.38291510603868,-7.77080727642779,12.1780057557933));
#74260=CARTESIAN_POINT('Ctrl Pts',(2.18075181987134,-7.82713287625985,12.1697851113704));
#74261=CARTESIAN_POINT('Ctrl Pts',(1.97861124538436,-7.88345214829104,12.1615653904815));
#74262=CARTESIAN_POINT('Ctrl Pts',(1.77427525044028,-7.93194012001247,12.1533456695925));
#74263=CARTESIAN_POINT('Ctrl Pts',(1.56836665514373,-7.97244715238259,12.1451259487036));
#74264=CARTESIAN_POINT('Ctrl Pts',(1.3624415611755,-8.01295743042696,12.1369055691997));
#74265=CARTESIAN_POINT('Ctrl Pts',(1.15494390415697,-8.04548543172001,12.1286851896958));
#74266=CARTESIAN_POINT('Ctrl Pts',(0.946506799953877,-8.06993261682779,
12.1204648101919));
#74267=CARTESIAN_POINT('Ctrl Pts',(0.73807046712045,-8.09437971146312,12.1122444611094));
#74268=CARTESIAN_POINT('Ctrl Pts',(0.528694987502466,-8.11074601800417,
12.1040241120269));
#74269=CARTESIAN_POINT('Ctrl Pts',(0.319019242010997,-8.11898480634905,
12.0958037629444));
#74270=CARTESIAN_POINT('Ctrl Pts',(0.109298665043695,-8.12722535625695,
12.0875816562415));
#74271=CARTESIAN_POINT('Ctrl Pts',(-0.10072201108176,-8.12733490464745,
12.0793595495385));
#74272=CARTESIAN_POINT('Ctrl Pts',(-0.310402138129443,-8.11931881841972,
12.0711374428356));
#74273=CARTESIAN_POINT('Ctrl Pts',(-0.402358250652034,-8.11580332967253,
12.0675316029318));
#74274=CARTESIAN_POINT('Ctrl Pts',(-0.494248874407456,-8.11072571421347,
12.0639257630279));
#74275=CARTESIAN_POINT('Ctrl Pts',(-0.58602011355852,-8.10408958421641,
12.0603199231241));
#74276=CARTESIAN_POINT('Ctrl Pts',(-0.795280045368397,-8.08895765264925,
12.0520977631165));
#74277=CARTESIAN_POINT('Ctrl Pts',(-1.00398810067131,-8.06571377663445,
12.043875603109));
#74278=CARTESIAN_POINT('Ctrl Pts',(-1.21150701712862,-8.03442208935703,
12.0356534431014));
#74279=CARTESIAN_POINT('Ctrl Pts',(-1.41898768177649,-8.00313617005334,
12.0274327986786));
#74280=CARTESIAN_POINT('Ctrl Pts',(-1.62527935336111,-7.96380544422755,
12.0192121542557));
#74281=CARTESIAN_POINT('Ctrl Pts',(-1.82975203947748,-7.9165456505049,12.0109915098328));
#74282=CARTESIAN_POINT('Ctrl Pts',(-2.03420175446741,-7.86929116610114,
12.0027717889439));
#74283=CARTESIAN_POINT('Ctrl Pts',(-2.23683260451198,-7.81410945861269,
11.994552068055));
#74284=CARTESIAN_POINT('Ctrl Pts',(-2.43702608327965,-7.75116710127673,
11.9863323471661));
#74285=CARTESIAN_POINT('Ctrl Pts',(-2.63723560278937,-7.68821970060906,
11.9781119676622));
#74286=CARTESIAN_POINT('Ctrl Pts',(-2.83500707841521,-7.61751049353422,
11.9698915881583));
#74287=CARTESIAN_POINT('Ctrl Pts',(-3.02973741038233,-7.53925585098621,
11.9616712086544));
#74288=CARTESIAN_POINT('Ctrl Pts',(-3.22446702170616,-7.46100149803706,
11.9534508595718));
#74289=CARTESIAN_POINT('Ctrl Pts',(-3.41615523902162,-7.37520187800216,
11.9452305104893));
#74290=CARTESIAN_POINT('Ctrl Pts',(-3.60421868720372,-7.28212161511406,
11.9370101614068));
#74291=CARTESIAN_POINT('Ctrl Pts',(-3.79232234586194,-7.18902145042302,
11.9287880547038));
#74292=CARTESIAN_POINT('Ctrl Pts',(-3.97679942246783,-7.08863766384462,
11.9205659480009));
#74293=CARTESIAN_POINT('Ctrl Pts',(-4.15708991467862,-6.98128147289431,
11.912343841298));
#74294=CARTESIAN_POINT('Ctrl Pts',(-4.23615707770353,-6.93419995823697,
11.9087380013942));
#74295=CARTESIAN_POINT('Ctrl Pts',(-4.31441936658964,-6.88577803085844,
11.9051321614904));
#74296=CARTESIAN_POINT('Ctrl Pts',(-4.39183118215718,-6.83604464803528,
11.9015263215866));
#74297=CARTESIAN_POINT('Ctrl Pts',(-4.56834826307476,-6.72264088020296,
11.893304161579));
#74298=CARTESIAN_POINT('Ctrl Pts',(-4.74049973721233,-6.60237783486906,
11.8850820015714));
#74299=CARTESIAN_POINT('Ctrl Pts',(-4.90775669096825,-6.47561671385486,
11.8768598415638));
#74300=CARTESIAN_POINT('Ctrl Pts',(-5.07498281437133,-6.34887895862604,
11.868639197141));
#74301=CARTESIAN_POINT('Ctrl Pts',(-5.23731598296318,-6.21564569651201,
11.8604185527182));
#74302=CARTESIAN_POINT('Ctrl Pts',(-5.39425835660122,-6.07631996727771,
11.8521979082954));
#74303=CARTESIAN_POINT('Ctrl Pts',(-5.55118309882289,-5.93700989034871,
11.8439781874066));
#74304=CARTESIAN_POINT('Ctrl Pts',(-5.70271803453674,-5.79160890861574,
11.8357584665177));
#74305=CARTESIAN_POINT('Ctrl Pts',(-5.84839973057559,-5.64055920577946,
11.8275387456288));
#74306=CARTESIAN_POINT('Ctrl Pts',(-5.99409309953547,-5.48949739990415,
11.8193183661249));
#74307=CARTESIAN_POINT('Ctrl Pts',(-6.13393208485477,-5.33278617911478,
11.811097986621));
#74308=CARTESIAN_POINT('Ctrl Pts',(-6.26749060693072,-5.17090408483228,
11.8028776071171));
#74309=CARTESIAN_POINT('Ctrl Pts',(-6.40104863474234,-5.00902258963207,
11.7946572580346));
#74310=CARTESIAN_POINT('Ctrl Pts',(-6.52832606003354,-4.84197048857877,
11.7864369089521));
#74311=CARTESIAN_POINT('Ctrl Pts',(-6.64893720971182,-4.67025925873603,
11.7782165598696));
#74312=CARTESIAN_POINT('Ctrl Pts',(-6.76957414766483,-4.49851131473889,
11.7699944531667));
#74313=CARTESIAN_POINT('Ctrl Pts',(-6.8835417927768,-4.32210249333724,11.7617723464638));
#74314=CARTESIAN_POINT('Ctrl Pts',(-6.99049728778659,-4.14157400416173,
11.7535502397609));
#74315=CARTESIAN_POINT('Ctrl Pts',(-7.03740307553505,-4.06240246655126,
11.749944399857));
#74316=CARTESIAN_POINT('Ctrl Pts',(-7.08296078985721,-3.98243895250165,
11.746338559953));
#74317=CARTESIAN_POINT('Ctrl Pts',(-7.12714424291815,-3.90173070612756,
11.7427327200491));
#74318=CARTESIAN_POINT('Ctrl Pts',(-7.22789287026477,-3.71769699046193,
11.7345105600415));
#74319=CARTESIAN_POINT('Ctrl Pts',(-7.32152626643292,-3.5297285961973,11.726288400034));
#74320=CARTESIAN_POINT('Ctrl Pts',(-7.4077527879426,-3.33839575173895,11.7180662400264));
#74321=CARTESIAN_POINT('Ctrl Pts',(-7.49396341538069,-3.14709817552375,
11.7098455956036));
#74322=CARTESIAN_POINT('Ctrl Pts',(-7.57276977191474,-2.95243765582687,
11.7016249511808));
#74323=CARTESIAN_POINT('Ctrl Pts',(-7.64392751697024,-2.75500629360535,
11.693404306758));
#74324=CARTESIAN_POINT('Ctrl Pts',(-7.71507726793335,-2.55759711146489,
11.6851845858691));
#74325=CARTESIAN_POINT('Ctrl Pts',(-7.77858002285569,-2.35741798580953,
11.6769648649802));
#74326=CARTESIAN_POINT('Ctrl Pts',(-7.83424038242487,-2.15507892961798,
11.6687451440913));
#74327=CARTESIAN_POINT('Ctrl Pts',(-7.88990520184711,-1.95272366076694,
11.6605247645874));
#74328=CARTESIAN_POINT('Ctrl Pts',(-7.93772628943084,-1.74820839943263,
11.6523043850835));
#74329=CARTESIAN_POINT('Ctrl Pts',(-7.97755844159658,-1.54215721423307,
11.6440840055796));
#74330=CARTESIAN_POINT('Ctrl Pts',(-8.01739044635451,-1.33610679157212,
11.635863656497));
#74331=CARTESIAN_POINT('Ctrl Pts',(-8.04923352143823,-1.12852074670183,
11.6276433074145));
#74332=CARTESIAN_POINT('Ctrl Pts',(-8.07299370265186,-0.92003273824542,
11.619422958332));
#74333=CARTESIAN_POINT('Ctrl Pts',(-8.09675896410922,-0.711500152271334,
11.6112008516291));
#74334=CARTESIAN_POINT('Ctrl Pts',(-8.11243784560138,-0.502065510735809,
11.6029787449263));
#74335=CARTESIAN_POINT('Ctrl Pts',(-8.11998820555982,-0.292368096873512,
11.5947566382235));
#74336=CARTESIAN_POINT('Ctrl Pts',(-8.12329944806874,-0.200404403140544,
11.5911507983195));
#74337=CARTESIAN_POINT('Ctrl Pts',(-8.12504800743336,-0.10839021155237,
11.5875449584156));
#74338=CARTESIAN_POINT('Ctrl Pts',(-8.12523349038375,-0.0163795374253974,
11.5839391185116));
#74339=CARTESIAN_POINT('Ctrl Pts',(-8.12524449288903,-0.0109216345524287,
11.5837252267631));
#74340=CARTESIAN_POINT('Ctrl Pts',(-8.12524999609811,-0.00546372059166464,
11.5835113350146));
#74341=CARTESIAN_POINT('Ctrl Pts',(-8.12524999999793,-5.80569704969686E-6,
11.5832974432661));
#74342=CARTESIAN_POINT('Origin',(0.,0.,24.4167025567876));
#74343=CARTESIAN_POINT('',(4.94675954817619,6.44587135576159,14.8749382835934));
#74344=CARTESIAN_POINT('',(4.94675954817621,6.44587135576157,14.708345136374));
#74345=CARTESIAN_POINT('',(4.9467595481762,6.44587135576158,24.4167025567876));
#74346=CARTESIAN_POINT('',(-8.12518161405221,1.07740023602867E-5,13.4167025566898));
#74347=CARTESIAN_POINT('Ctrl Pts',(4.94675954817621,6.44587135576157,14.708345136374));
#74348=CARTESIAN_POINT('Ctrl Pts',(5.114411914168,6.31720978365264,14.7000673201305));
#74349=CARTESIAN_POINT('Ctrl Pts',(5.2770488708113,6.18199860132526,14.691789503887));
#74350=CARTESIAN_POINT('Ctrl Pts',(5.43416681847959,6.04065547365808,14.6835116876434));
#74351=CARTESIAN_POINT('Ctrl Pts',(5.59019297142775,5.90029452328386,14.675291393002));
#74352=CARTESIAN_POINT('Ctrl Pts',(5.74077637035415,5.75388679711431,14.6670710983606));
#74353=CARTESIAN_POINT('Ctrl Pts',(5.88545887966758,5.60188016100327,14.6588508037191));
#74354=CARTESIAN_POINT('Ctrl Pts',(6.0316600151547,5.44827802273188,14.6505442266745));
#74355=CARTESIAN_POINT('Ctrl Pts',(6.1718354600305,5.28895898314362,14.6422376496299));
#74356=CARTESIAN_POINT('Ctrl Pts',(6.30555199892502,5.12442206998533,14.6339310725854));
#74357=CARTESIAN_POINT('Ctrl Pts',(6.43926853781952,4.95988515682704,14.6256244955408));
#74358=CARTESIAN_POINT('Ctrl Pts',(6.5665259809629,4.79013061612021,14.6173179184962));
#74359=CARTESIAN_POINT('Ctrl Pts',(6.6869338165474,4.61569103121243,14.6090113414516));
#74360=CARTESIAN_POINT('Ctrl Pts',(6.80611798651609,4.4430242189905,14.600789181444));
#74361=CARTESIAN_POINT('Ctrl Pts',(6.91863046891195,4.2657101715334,14.5925670214365));
#74362=CARTESIAN_POINT('Ctrl Pts',(7.02412238836637,4.08428601297097,14.5843448614289));
#74363=CARTESIAN_POINT('Ctrl Pts',(7.12959486257268,3.90289529619058,14.5761242170061));
#74364=CARTESIAN_POINT('Ctrl Pts',(7.22804920838932,3.71739623541434,14.5679035725832));
#74365=CARTESIAN_POINT('Ctrl Pts',(7.31918134643846,3.52835258731993,14.5596829281604));
#74366=CARTESIAN_POINT('Ctrl Pts',(7.41030324640646,3.33933017700453,14.5514632072715));
#74367=CARTESIAN_POINT('Ctrl Pts',(7.49410445275709,3.14676424012889,14.5432434863826));
#74368=CARTESIAN_POINT('Ctrl Pts',(7.57032772002814,2.95124139539169,14.5350237654938));
#74369=CARTESIAN_POINT('Ctrl Pts',(7.64655709478004,2.7557028841517,14.5268033859899));
#74370=CARTESIAN_POINT('Ctrl Pts',(7.71520720747419,2.55720726565261,14.518583006486));
#74371=CARTESIAN_POINT('Ctrl Pts',(7.77606929191176,2.35636031410456,14.5103626269821));
#74372=CARTESIAN_POINT('Ctrl Pts',(7.83693115111535,2.15551410583629,14.5021422778996));
#74373=CARTESIAN_POINT('Ctrl Pts',(7.89000495667738,1.95231686515983,14.4939219288171));
#74374=CARTESIAN_POINT('Ctrl Pts',(7.93513192012207,1.74738918754804,14.4857015797346));
#74375=CARTESIAN_POINT('Ctrl Pts',(7.9802685323141,1.5424176936625,14.4774794730317));
#74376=CARTESIAN_POINT('Ctrl Pts',(8.01745484434982,1.33571531196892,14.4692573663288));
#74377=CARTESIAN_POINT('Ctrl Pts',(8.04658303441186,1.12791357506469,14.4610352596259));
#74378=CARTESIAN_POINT('Ctrl Pts',(8.05935732619011,1.03678123853476,14.4574294197219));
#74379=CARTESIAN_POINT('Ctrl Pts',(8.070582466931,0.945437573572713,14.453823579818));
#74380=CARTESIAN_POINT('Ctrl Pts',(8.08025249693006,0.853936267150792,14.4502177399141));
#74381=CARTESIAN_POINT('Ctrl Pts',(8.10230243149423,0.645291845227277,14.4419955799065));
#74382=CARTESIAN_POINT('Ctrl Pts',(8.11627041002579,0.435758492998309,14.433773419899));
#74383=CARTESIAN_POINT('Ctrl Pts',(8.12210705167606,0.225974785350209,14.4255512598914));
#74384=CARTESIAN_POINT('Ctrl Pts',(8.12794261746245,0.0162297469791537,
14.4173306154685));
#74385=CARTESIAN_POINT('Ctrl Pts',(8.12564982964777,-0.193765259826035,
14.4091099710457));
#74386=CARTESIAN_POINT('Ctrl Pts',(8.11523138570146,-0.40336970514151,14.4008893266229));
#74387=CARTESIAN_POINT('Ctrl Pts',(8.10481411219706,-0.612950602811235,
14.392669605734));
#74388=CARTESIAN_POINT('Ctrl Pts',(8.08627301967335,-0.822140731925243,
14.3844498848451));
#74389=CARTESIAN_POINT('Ctrl Pts',(8.05966286954378,-1.03030189352312,14.3762301639562));
#74390=CARTESIAN_POINT('Ctrl Pts',(8.03305058724397,-1.23847973428408,14.3680097844523));
#74391=CARTESIAN_POINT('Ctrl Pts',(7.9983679901989,-1.44562814967399,14.3597894049484));
#74392=CARTESIAN_POINT('Ctrl Pts',(7.9557215752874,-1.65111531366121,14.3515690254445));
#74393=CARTESIAN_POINT('Ctrl Pts',(7.91307531819866,-1.85660171719642,14.343348676362));
#74394=CARTESIAN_POINT('Ctrl Pts',(7.86246536478753,-2.06042659318347,14.3351283272795));
#74395=CARTESIAN_POINT('Ctrl Pts',(7.80404918960463,-2.26196901144363,14.326907978197));
#74396=CARTESIAN_POINT('Ctrl Pts',(7.74562052426347,-2.46355452216395,14.3186858714941));
#74397=CARTESIAN_POINT('Ctrl Pts',(7.6793823848452,-2.66285631665436,14.3104637647912));
#74398=CARTESIAN_POINT('Ctrl Pts',(7.6055422336979,-2.859268244488,14.3022416580883));
#74399=CARTESIAN_POINT('Ctrl Pts',(7.57315932100455,-2.94540553175171,14.2986358181844));
#74400=CARTESIAN_POINT('Ctrl Pts',(7.53931495249193,-3.03098723326055,14.2950299782805));
#74401=CARTESIAN_POINT('Ctrl Pts',(7.50402958019213,-3.11596335378026,14.2914241383766));
#74402=CARTESIAN_POINT('Ctrl Pts',(7.42357066223984,-3.30972882267504,14.283201978369));
#74403=CARTESIAN_POINT('Ctrl Pts',(7.33558947662495,-3.50040824237825,14.2749798183615));
#74404=CARTESIAN_POINT('Ctrl Pts',(7.2403481734786,-3.68741723829905,14.2667576583539));
#74405=CARTESIAN_POINT('Ctrl Pts',(7.14512442609186,-3.87439176298871,14.258537013931));
#74406=CARTESIAN_POINT('Ctrl Pts',(7.04264336601514,-4.05769695136209,14.2503163695082));
#74407=CARTESIAN_POINT('Ctrl Pts',(6.93321381006366,-4.23677162783676,14.2420957250853));
#74408=CARTESIAN_POINT('Ctrl Pts',(6.82379654778472,-4.41582618647934,14.2338760041965));
#74409=CARTESIAN_POINT('Ctrl Pts',(6.70743250191391,-4.59065093032095,14.2256562833076));
#74410=CARTESIAN_POINT('Ctrl Pts',(6.58447509278105,-4.76071163956041,14.2174365624187));
#74411=CARTESIAN_POINT('Ctrl Pts',(6.46150783153811,-4.93078597511844,14.2092161829148));
#74412=CARTESIAN_POINT('Ctrl Pts',(6.3319463221571,-5.09609527256796,14.2009958034109));
#74413=CARTESIAN_POINT('Ctrl Pts',(6.19618636624322,-5.25613566009114,14.192775423907));
#74414=CARTESIAN_POINT('Ctrl Pts',(6.06042691274,-5.41617545534837,14.1845550748245));
#74415=CARTESIAN_POINT('Ctrl Pts',(5.91846925155094,-5.5709461563389,14.176334725742));
#74416=CARTESIAN_POINT('Ctrl Pts',(5.77074873622009,-5.71997784837619,14.1681143766595));
#74417=CARTESIAN_POINT('Ctrl Pts',(5.62299663627054,-5.86904140537926,14.1598922699565));
#74418=CARTESIAN_POINT('Ctrl Pts',(5.46947942834891,-6.01236329230735,14.1516701632536));
#74419=CARTESIAN_POINT('Ctrl Pts',(5.31066929053358,-6.14951048857416,14.1434480565507));
#74420=CARTESIAN_POINT('Ctrl Pts',(5.24102242838857,-6.20965697546328,14.1398422166468));
#74421=CARTESIAN_POINT('Ctrl Pts',(5.17035803189016,-6.26861638506664,14.1362363767429));
#74422=CARTESIAN_POINT('Ctrl Pts',(5.09871797967465,-6.32635460010285,14.132630536839));
#74423=CARTESIAN_POINT('Ctrl Pts',(4.93536187181506,-6.45801126130546,14.1244083768314));
#74424=CARTESIAN_POINT('Ctrl Pts',(4.7668767188342,-6.58335911069089,14.1161862168239));
#74425=CARTESIAN_POINT('Ctrl Pts',(4.5937723033958,-6.7020104138276,14.1079640568163));
#74426=CARTESIAN_POINT('Ctrl Pts',(4.42069979616723,-6.8206398460567,14.0997434123934));
#74427=CARTESIAN_POINT('Ctrl Pts',(4.24300996921065,-6.93257502888713,14.0915227679706));
#74428=CARTESIAN_POINT('Ctrl Pts',(4.0612424853508,-7.0374709262406,14.0833021235477));
#74429=CARTESIAN_POINT('Ctrl Pts',(3.87949542184197,-7.14235503924738,14.0750824026589));
#74430=CARTESIAN_POINT('Ctrl Pts',(3.69367187151863,-7.24020129812285,14.06686268177));
#74431=CARTESIAN_POINT('Ctrl Pts',(3.50433776829408,-7.33070967698269,14.0586429608811));
#74432=CARTESIAN_POINT('Ctrl Pts',(3.31498849444716,-7.42122530793507,14.0504225813772));
#74433=CARTESIAN_POINT('Ctrl Pts',(3.12212837077274,-7.50440175431621,14.0422022018733));
#74434=CARTESIAN_POINT('Ctrl Pts',(2.92634602793832,-7.57998591603372,14.0339818223694));
#74435=CARTESIAN_POINT('Ctrl Pts',(2.73056440964105,-7.65556979803483,14.0257614732869));
#74436=CARTESIAN_POINT('Ctrl Pts',(2.53186087011539,-7.72356134776954,14.0175411242044));
#74437=CARTESIAN_POINT('Ctrl Pts',(2.3308425255473,-7.7837562065882,14.0093207751219));
#74438=CARTESIAN_POINT('Ctrl Pts',(2.12978120057295,-7.84396393587145,14.001098668419));
#74439=CARTESIAN_POINT('Ctrl Pts',(1.92640436456651,-7.89637155914005,13.9928765617161));
#74440=CARTESIAN_POINT('Ctrl Pts',(1.72133381909578,-7.94082473334711,13.9846544550132));
#74441=CARTESIAN_POINT('Ctrl Pts',(1.63139925819907,-7.96031986217509,13.9810486151093));
#74442=CARTESIAN_POINT('Ctrl Pts',(1.54113910590134,-7.9782857693441,13.9774427752054));
#74443=CARTESIAN_POINT('Ctrl Pts',(1.45060645962889,-7.99471253152876,13.9738369353015));
#74444=CARTESIAN_POINT('Ctrl Pts',(1.24417080984958,-8.03216939891287,13.9656147752939));
#74445=CARTESIAN_POINT('Ctrl Pts',(1.03624952957575,-8.06163244915906,13.9573926152864));
#74446=CARTESIAN_POINT('Ctrl Pts',(0.827475775738013,-8.08300509730551,
13.9491704552788));
#74447=CARTESIAN_POINT('Ctrl Pts',(0.618740505013095,-8.1043738058474,13.940949810856));
#74448=CARTESIAN_POINT('Ctrl Pts',(0.40915336780636,-8.11765505867199,13.9327291664331));
#74449=CARTESIAN_POINT('Ctrl Pts',(0.199353331470842,-8.12280406089741,
13.9245085220103));
#74450=CARTESIAN_POINT('Ctrl Pts',(-0.0104231352455265,-8.12795248466715,
13.9162888011214));
#74451=CARTESIAN_POINT('Ctrl Pts',(-0.22041215840231,-8.12497047454427,
13.9080690802325));
#74452=CARTESIAN_POINT('Ctrl Pts',(-0.429973235496852,-8.1138653291299,
13.8998493593436));
#74453=CARTESIAN_POINT('Ctrl Pts',(-0.639551103924294,-8.10275929390243,
13.8916289798397));
#74454=CARTESIAN_POINT('Ctrl Pts',(-0.848700662891006,-8.08352883576082,
13.8834086003358));
#74455=CARTESIAN_POINT('Ctrl Pts',(-1.05678392993916,-8.05623331886077,
13.8751882208319));
#74456=CARTESIAN_POINT('Ctrl Pts',(-1.26486642692787,-8.02893790297398,
13.8669678717494));
#74457=CARTESIAN_POINT('Ctrl Pts',(-1.4718823476019,-7.99357752906663,13.8587475226669));
#74458=CARTESIAN_POINT('Ctrl Pts',(-1.67720079620484,-7.95026320644228,
13.8505271735844));
#74459=CARTESIAN_POINT('Ctrl Pts',(-1.88256314463373,-7.90693962263736,
13.8423050668815));
#74460=CARTESIAN_POINT('Ctrl Pts',(-2.08622700705732,-7.85565875346183,
13.8340829601786));
#74461=CARTESIAN_POINT('Ctrl Pts',(-2.28757252101541,-7.79658255414481,
13.8258608534757));
#74462=CARTESIAN_POINT('Ctrl Pts',(-2.3758734534811,-7.77067443539076,13.8222550135718));
#74463=CARTESIAN_POINT('Ctrl Pts',(-2.46372867229529,-7.74326769460846,
13.8186491736679));
#74464=CARTESIAN_POINT('Ctrl Pts',(-2.55108680360823,-7.7143790212146,13.815043333764));
#74465=CARTESIAN_POINT('Ctrl Pts',(-2.75028381533406,-7.64850607583112,
13.8068211737565));
#74466=CARTESIAN_POINT('Ctrl Pts',(-2.94696092416245,-7.57490278118075,
13.7985990137489));
#74467=CARTESIAN_POINT('Ctrl Pts',(-3.14051592933454,-7.49378724411736,
13.7903768537413));
#74468=CARTESIAN_POINT('Ctrl Pts',(-3.33403525665469,-7.41268665902133,
13.7821562093185));
#74469=CARTESIAN_POINT('Ctrl Pts',(-3.52443335685868,-7.32407670925368,
13.7739355648956));
#74470=CARTESIAN_POINT('Ctrl Pts',(-3.71112770477992,-7.22822375977078,
13.7657149204728));
#74471=CARTESIAN_POINT('Ctrl Pts',(-3.89780107885027,-7.13238157872032,
13.7574951995839));
#74472=CARTESIAN_POINT('Ctrl Pts',(-4.08077126887934,-7.02929815720436,
13.749275478695));
#74473=CARTESIAN_POINT('Ctrl Pts',(-4.25947932467885,-6.91928633929348,
13.7410557578061));
#74474=CARTESIAN_POINT('Ctrl Pts',(-4.43820169967596,-6.80926570655357,
13.7328353783022));
#74475=CARTESIAN_POINT('Ctrl Pts',(-4.61266100529772,-6.69231572058388,
13.7246149987983));
#74476=CARTESIAN_POINT('Ctrl Pts',(-4.78232541394498,-6.56879373992181,
13.7163946192944));
#74477=CARTESIAN_POINT('Ctrl Pts',(-4.95198919471046,-6.44527221638096,
13.7081742702119));
#74478=CARTESIAN_POINT('Ctrl Pts',(-5.11685787696167,-6.31517892267167,
13.6999539211294));
#74479=CARTESIAN_POINT('Ctrl Pts',(-5.27643056465477,-6.17891317780699,
13.6917335720469));
#74480=CARTESIAN_POINT('Ctrl Pts',(-5.43603737111922,-6.04261829750657,
13.683511465344));
#74481=CARTESIAN_POINT('Ctrl Pts',(-5.59034569631145,-5.90014852114324,
13.6752893586411));
#74482=CARTESIAN_POINT('Ctrl Pts',(-5.73888870682318,-5.75194262603491,
13.6670672519382));
#74483=CARTESIAN_POINT('Ctrl Pts',(-5.80403287657228,-5.68694629968139,
13.6634614120343));
#74484=CARTESIAN_POINT('Ctrl Pts',(-5.86806866921949,-5.62084723634984,
13.6598555721304));
#74485=CARTESIAN_POINT('Ctrl Pts',(-5.93095895674066,-5.55368467019489,
13.6562497322265));
#74486=CARTESIAN_POINT('Ctrl Pts',(-6.07436355059454,-5.40053827984976,
13.6480275722189));
#74487=CARTESIAN_POINT('Ctrl Pts',(-6.21185692826895,-5.24180926165742,
13.6398054122113));
#74488=CARTESIAN_POINT('Ctrl Pts',(-6.34301463012504,-5.07797725128025,
13.6315832522037));
#74489=CARTESIAN_POINT('Ctrl Pts',(-6.47414815577779,-4.91417543993784,
13.6233626077809));
#74490=CARTESIAN_POINT('Ctrl Pts',(-6.59894815212011,-4.74527274406864,
13.6151419633581));
#74491=CARTESIAN_POINT('Ctrl Pts',(-6.71703052524307,-4.57178176266681,
13.6069213189352));
#74492=CARTESIAN_POINT('Ctrl Pts',(-6.83509963260764,-4.39831027180688,
13.5987015980464));
#74493=CARTESIAN_POINT('Ctrl Pts',(-6.94645245741672,-4.22025176839447,
13.5904818771575));
#74494=CARTESIAN_POINT('Ctrl Pts',(-7.05074784452481,-4.03814838699976,
13.5822621562686));
#74495=CARTESIAN_POINT('Ctrl Pts',(-7.1550515884264,-3.8560304143523,13.5740417767647));
#74496=CARTESIAN_POINT('Ctrl Pts',(-7.25229661567336,-3.66986717090157,
13.5658213972608));
#74497=CARTESIAN_POINT('Ctrl Pts',(-7.34218688518948,-3.48022690430547,
13.5576010177569));
#74498=CARTESIAN_POINT('Ctrl Pts',(-7.43207682204622,-3.2905873395163,13.5493806686744));
#74499=CARTESIAN_POINT('Ctrl Pts',(-7.51461193161352,-3.09747104516457,
13.5411603195919));
#74500=CARTESIAN_POINT('Ctrl Pts',(-7.58954340973417,-2.9014683169493,13.5329399705094));
#74501=CARTESIAN_POINT('Ctrl Pts',(-7.66449090920535,-2.70542368073367,
13.5247178638065));
#74502=CARTESIAN_POINT('Ctrl Pts',(-7.7318314238663,-2.50649165343321,13.5164957571036));
#74503=CARTESIAN_POINT('Ctrl Pts',(-7.79136493885135,-2.30528088356667,
13.5082736504007));
#74504=CARTESIAN_POINT('Ctrl Pts',(-7.81747361533904,-2.21703904369537,
13.5046678104968));
#74505=CARTESIAN_POINT('Ctrl Pts',(-7.84208141545661,-2.12835914131216,
13.5010619705928));
#74506=CARTESIAN_POINT('Ctrl Pts',(-7.86517450686973,-2.03929339208129,
13.4974561306889));
#74507=CARTESIAN_POINT('Ctrl Pts',(-7.91844463505754,-1.83384043674525,
13.4891383376975));
#74508=CARTESIAN_POINT('Ctrl Pts',(-7.96366713914132,-1.6262728969258,13.4808205447061));
#74509=CARTESIAN_POINT('Ctrl Pts',(-8.000696703205,-1.41722963059086,13.4725027517147));
#74510=CARTESIAN_POINT('Ctrl Pts',(-8.03771839720457,-1.2082307931858,13.4641867265422));
#74511=CARTESIAN_POINT('Ctrl Pts',(-8.06655057873264,-0.997757131489211,
13.4558707013697));
#74512=CARTESIAN_POINT('Ctrl Pts',(-8.08709916325463,-0.786457046625093,
13.4475546761972));
#74513=CARTESIAN_POINT('Ctrl Pts',(-8.10764404340868,-0.575195053594521,
13.4392401501847));
#74514=CARTESIAN_POINT('Ctrl Pts',(-8.11990828074441,-0.363107213867596,
13.4309256241723));
#74515=CARTESIAN_POINT('Ctrl Pts',(-8.12384961901664,-0.15084737353743,
13.4226110981598));
#74516=CARTESIAN_POINT('Ctrl Pts',(-8.12478322846949,-0.100568057299159,
13.4206415843691));
#74517=CARTESIAN_POINT('Ctrl Pts',(-8.12525006666185,-0.0502791050878931,
13.4186720705783));
#74518=CARTESIAN_POINT('Ctrl Pts',(-8.12524999999286,1.07715953333801E-5,
13.4167025567876));
#74519=CARTESIAN_POINT('Ctrl Pts',(-8.12455564661523,1.07960349659537E-5,
13.4167025557943));
#74520=CARTESIAN_POINT('Ctrl Pts',(-8.12458628377602,0.664182828634124,
13.39068921358));
#74521=CARTESIAN_POINT('Ctrl Pts',(-7.88026825892223,2.67977085846249,13.3117446708532));
#74522=CARTESIAN_POINT('Ctrl Pts',(-6.23176414069403,5.73643646235047,13.1798689276139));
#74523=CARTESIAN_POINT('Ctrl Pts',(-2.72779796832367,8.01877209027872,13.0210753260764));
#74524=CARTESIAN_POINT('Ctrl Pts',(1.39851398942074,8.34320643186221,12.8639024043266));
#74525=CARTESIAN_POINT('Ctrl Pts',(3.90815072701549,7.2432900977911,12.7596606830893));
#74526=CARTESIAN_POINT('Ctrl Pts',(4.94717300284021,6.44641043468649,12.7083501623644));
#74527=CARTESIAN_POINT('',(-8.12524999926494,-0.000109293386091071,13.5832974432338));
#74528=CARTESIAN_POINT('Ctrl Pts',(-8.12524999926495,-0.000109292839731289,
13.5832974432124));
#74529=CARTESIAN_POINT('Ctrl Pts',(-8.12525283523286,0.210727467548692,
13.5750400395771));
#74530=CARTESIAN_POINT('Ctrl Pts',(-8.11704503066721,0.421561740255473,
13.5667826359418));
#74531=CARTESIAN_POINT('Ctrl Pts',(-8.1006532199022,0.631747555110545,13.5585252323065));
#74532=CARTESIAN_POINT('Ctrl Pts',(-8.08426130399346,0.841934718182757,
13.5502677757049));
#74533=CARTESIAN_POINT('Ctrl Pts',(-8.05968530261826,1.05147312662298,13.5420103191033));
#74534=CARTESIAN_POINT('Ctrl Pts',(-8.02700379967336,1.25972122413236,13.5337528625017));
#74535=CARTESIAN_POINT('Ctrl Pts',(-7.9943137565393,1.46802374013491,13.5254932480971));
#74536=CARTESIAN_POINT('Ctrl Pts',(-7.95351402346721,1.67503498511879,13.5172336336926));
#74537=CARTESIAN_POINT('Ctrl Pts',(-7.90473466922945,1.88012163744318,13.5089740192881));
#74538=CARTESIAN_POINT('Ctrl Pts',(-7.86632418913691,2.04161366413042,13.5024701251793));
#74539=CARTESIAN_POINT('Ctrl Pts',(-7.82296696247514,2.20191247086353,13.4959662310706));
#74540=CARTESIAN_POINT('Ctrl Pts',(-7.77474855855956,2.36071438629835,13.4894623369618));
#74541=CARTESIAN_POINT('Ctrl Pts',(-7.7137913188393,2.56147023139319,13.4812401769542));
#74542=CARTESIAN_POINT('Ctrl Pts',(-7.64504413156814,2.75989692910004,13.4730180169467));
#74543=CARTESIAN_POINT('Ctrl Pts',(-7.56871023699752,2.95538710000382,13.4647958569391));
#74544=CARTESIAN_POINT('Ctrl Pts',(-7.49239041299751,3.15084123634824,13.4565752125162));
#74545=CARTESIAN_POINT('Ctrl Pts',(-7.40848678011347,3.34335965143663,13.4483545680934));
#74546=CARTESIAN_POINT('Ctrl Pts',(-7.31725130570271,3.53235344942885,13.4401339236705));
#74547=CARTESIAN_POINT('Ctrl Pts',(-7.22602608098177,3.72132601524338,13.4319142027816));
#74548=CARTESIAN_POINT('Ctrl Pts',(-7.12747078741842,3.9067744887932,13.4236944818926));
#74549=CARTESIAN_POINT('Ctrl Pts',(-7.02188443686295,4.08813239974464,13.4154747610037));
#74550=CARTESIAN_POINT('Ctrl Pts',(-6.91628962607497,4.26950484221541,13.4072543814998));
#74551=CARTESIAN_POINT('Ctrl Pts',(-6.80366277876538,4.44678581074138,13.3990340019959));
#74552=CARTESIAN_POINT('Ctrl Pts',(-6.68434807441564,4.61943485532115,13.390813622492));
#74553=CARTESIAN_POINT('Ctrl Pts',(-6.5650338116171,4.79208326097386,13.3825932734095));
#74554=CARTESIAN_POINT('Ctrl Pts',(-6.43903191128112,4.9600995356832,13.374372924327));
#74555=CARTESIAN_POINT('Ctrl Pts',(-6.3067292609164,5.12297312036682,13.3661525752444));
#74556=CARTESIAN_POINT('Ctrl Pts',(-6.17439832247844,5.28588152959763,13.3579304685415));
#74557=CARTESIAN_POINT('Ctrl Pts',(-6.03576412872503,5.44364482293004,13.3497083618386));
#74558=CARTESIAN_POINT('Ctrl Pts',(-5.89125385073188,5.59578552383281,13.3414862551357));
#74559=CARTESIAN_POINT('Ctrl Pts',(-5.82787825300201,5.66250747601956,13.3378804152319));
#74560=CARTESIAN_POINT('Ctrl Pts',(-5.76337301003238,5.728148488673,13.3342745753281));
#74561=CARTESIAN_POINT('Ctrl Pts',(-5.69777643160394,5.79267048069875,13.3306687354243));
#74562=CARTESIAN_POINT('Ctrl Pts',(-5.5482008602592,5.93979574321652,13.3224465754167));
#74563=CARTESIAN_POINT('Ctrl Pts',(-5.39289906328124,6.08114878342411,13.3142244154092));
#74564=CARTESIAN_POINT('Ctrl Pts',(-5.23234009919822,6.21629348155493,13.3060022554016));
#74565=CARTESIAN_POINT('Ctrl Pts',(-5.07181073083084,6.35141326856304,13.2977816109787));
#74566=CARTESIAN_POINT('Ctrl Pts',(-4.90602635513595,6.48032680755237,13.2895609665559));
#74567=CARTESIAN_POINT('Ctrl Pts',(-4.73548997611329,6.60263752212936,13.281340322133));
#74568=CARTESIAN_POINT('Ctrl Pts',(-4.56497275570302,6.72493449592221,13.2731206012441));
#74569=CARTESIAN_POINT('Ctrl Pts',(-4.38970483751106,6.84062995427466,13.2649008803552));
#74570=CARTESIAN_POINT('Ctrl Pts',(-4.21021980752773,6.94936952066885,13.2566811594664));
#74571=CARTESIAN_POINT('Ctrl Pts',(-4.03072039609063,7.0581177999515,13.2484607799625));
#74572=CARTESIAN_POINT('Ctrl Pts',(-3.84700344872614,7.15990891836325,13.2402404004585));
#74573=CARTESIAN_POINT('Ctrl Pts',(-3.65962976542472,7.25443295802762,13.2320200209546));
#74574=CARTESIAN_POINT('Ctrl Pts',(-3.47225677554188,7.34895664788447,13.2237996718721));
#74575=CARTESIAN_POINT('Ctrl Pts',(-3.28122734150666,7.43621318224071,13.2155793227896));
#74576=CARTESIAN_POINT('Ctrl Pts',(-3.08712546566586,7.51593932397923,13.207358973707));
#74577=CARTESIAN_POINT('Ctrl Pts',(-2.89298208825296,7.5956825122311,13.1991368670041));
#74578=CARTESIAN_POINT('Ctrl Pts',(-2.69576522968438,7.66789197904101,13.1909147603012));
#74579=CARTESIAN_POINT('Ctrl Pts',(-2.49607843871186,7.73235281077485,13.1826926535983));
#74580=CARTESIAN_POINT('Ctrl Pts',(-2.40850494627522,7.76062238300249,13.1790868136945));
#74581=CARTESIAN_POINT('Ctrl Pts',(-2.32045663554736,7.78740229881576,13.1754809737906));
#74582=CARTESIAN_POINT('Ctrl Pts',(-2.23198536645222,7.81267744671717,13.1718751338868));
#74583=CARTESIAN_POINT('Ctrl Pts',(-2.03025013971722,7.87031070715078,13.1636529738792));
#74584=CARTESIAN_POINT('Ctrl Pts',(-1.82624816262755,7.92013563528932,13.1554308138716));
#74585=CARTESIAN_POINT('Ctrl Pts',(-1.62059998012985,7.96199367413107,13.1472086538641));
#74586=CARTESIAN_POINT('Ctrl Pts',(-1.41498970461059,8.00384399731126,13.1389880094412));
#74587=CARTESIAN_POINT('Ctrl Pts',(-1.20773411838256,8.03773030334217,13.1307673650184));
#74588=CARTESIAN_POINT('Ctrl Pts',(-0.999464656104813,8.06354499979366,
13.1225467205955));
#74589=CARTESIAN_POINT('Ctrl Pts',(-0.791218591497348,8.089356796138,13.1143269997066));
#74590=CARTESIAN_POINT('Ctrl Pts',(-0.581959171024286,8.10709875695665,
13.1061072788178));
#74591=CARTESIAN_POINT('Ctrl Pts',(-0.372324494548209,8.11671497794886,
13.0978875579289));
#74592=CARTESIAN_POINT('Ctrl Pts',(-0.162673020841052,8.12633196945237,
13.089667178425));
#74593=CARTESIAN_POINT('Ctrl Pts',(0.0473534742294832,8.12782190394492,
13.0814467989211));
#74594=CARTESIAN_POINT('Ctrl Pts',(0.25711426377705,8.12118093739219,13.0732264194172));
#74595=CARTESIAN_POINT('Ctrl Pts',(0.466874277057171,8.11453999541588,13.0650060703347));
#74596=CARTESIAN_POINT('Ctrl Pts',(0.676368291869704,8.0997682245935,13.0567857212522));
#74597=CARTESIAN_POINT('Ctrl Pts',(0.88495754015993,8.0769138731705,13.0485653721696));
#74598=CARTESIAN_POINT('Ctrl Pts',(1.09359138761617,8.05405463518205,13.0403432654667));
#74599=CARTESIAN_POINT('Ctrl Pts',(1.30131978862463,8.02310939620984,13.0321211587638));
#74600=CARTESIAN_POINT('Ctrl Pts',(1.50750993027571,7.98417819018464,13.0238990520609));
#74601=CARTESIAN_POINT('Ctrl Pts',(1.5979354948449,7.96710474401501,13.020293212157));
#74602=CARTESIAN_POINT('Ctrl Pts',(1.68806531497049,7.94849602462319,13.0166873722531));
#74603=CARTESIAN_POINT('Ctrl Pts',(1.777846621314,7.92836357349878,13.0130815323492));
#74604=CARTESIAN_POINT('Ctrl Pts',(1.98256750933193,7.88245721013628,13.0048594338162));
#74605=CARTESIAN_POINT('Ctrl Pts',(2.18554318373643,7.82860978502314,12.9966373352832));
#74606=CARTESIAN_POINT('Ctrl Pts',(2.38615288333715,7.7669789480751,12.9884152367502));
#74607=CARTESIAN_POINT('Ctrl Pts',(2.58672500987442,7.70535965423466,12.9801946781698));
#74608=CARTESIAN_POINT('Ctrl Pts',(2.78493176410168,7.63595994484411,12.9719741195894));
#74609=CARTESIAN_POINT('Ctrl Pts',(2.98016721010928,7.55898742969516,12.963753561009));
#74610=CARTESIAN_POINT('Ctrl Pts',(3.17539843895926,7.48201657718093,12.9555331799957));
#74611=CARTESIAN_POINT('Ctrl Pts',(3.36765821197506,7.39747335061567,12.9473127989824));
#74612=CARTESIAN_POINT('Ctrl Pts',(3.55635930970939,7.3056140072374,12.9390924179691));
#74613=CARTESIAN_POINT('Ctrl Pts',(3.7450472715417,7.21376105839181,12.9308726091948));
#74614=CARTESIAN_POINT('Ctrl Pts',(3.93017678811928,7.114593140326,12.9226528004204));
#74615=CARTESIAN_POINT('Ctrl Pts',(4.11118349949156,7.0084133579583,12.9144329916461));
#74616=CARTESIAN_POINT('Ctrl Pts',(4.29221574062193,6.90221859965883,12.9062120235239));
#74617=CARTESIAN_POINT('Ctrl Pts',(4.46912375957649,6.78901014955914,12.8979910554018));
#74618=CARTESIAN_POINT('Ctrl Pts',(4.64136960010035,6.66913606082259,12.8897700872797));
#74619=CARTESIAN_POINT('Ctrl Pts',(4.74488681134554,6.59709350044014,12.8848294066156));
#74620=CARTESIAN_POINT('Ctrl Pts',(4.84672065219238,6.52264427544677,12.8798887259516));
#74621=CARTESIAN_POINT('Ctrl Pts',(4.94675954817619,6.44587135576158,12.8749480452876));
#74622=CARTESIAN_POINT('Ctrl Pts',(4.94675954817619,6.44587135576159,14.8749382835934));
#74623=CARTESIAN_POINT('Ctrl Pts',(5.11322618946787,6.31811974518586,14.8667184029981));
#74624=CARTESIAN_POINT('Ctrl Pts',(5.27475363759568,6.18390667886123,14.8584985224029));
#74625=CARTESIAN_POINT('Ctrl Pts',(5.4308477106004,6.04363969034938,14.8502786418076));
#74626=CARTESIAN_POINT('Ctrl Pts',(5.58695298024303,5.90336264047741,14.8420581715998));
#74627=CARTESIAN_POINT('Ctrl Pts',(5.73762387428406,5.75703099557787,14.833837701392));
#74628=CARTESIAN_POINT('Ctrl Pts',(5.88240082059063,5.6050912703019,14.8256172311841));
#74629=CARTESIAN_POINT('Ctrl Pts',(6.02717483279472,5.45315462429192,14.8173969275754));
#74630=CARTESIAN_POINT('Ctrl Pts',(6.16605493402484,5.29561034031495,14.8091766239666));
#74631=CARTESIAN_POINT('Ctrl Pts',(6.29861946790666,5.13294071278904,14.8009563203578));
#74632=CARTESIAN_POINT('Ctrl Pts',(6.43121433767825,4.97023386016418,14.7927341356258));
#74633=CARTESIAN_POINT('Ctrl Pts',(6.55749056529819,4.80239954892059,14.7845119508938));
#74634=CARTESIAN_POINT('Ctrl Pts',(6.67706701070395,4.62995288281307,14.7762897661618));
#74635=CARTESIAN_POINT('Ctrl Pts',(6.75695066281212,4.51474901104883,14.7707968938619));
#74636=CARTESIAN_POINT('Ctrl Pts',(6.8338450645536,4.39748732251782,14.7653040215619));
#74637=CARTESIAN_POINT('Ctrl Pts',(6.907647309015,4.27832867095993,14.7598111492619));
#74638=CARTESIAN_POINT('Ctrl Pts',(7.01812026919681,4.09996270031851,14.7515889892543));
#74639=CARTESIAN_POINT('Ctrl Pts',(7.1216992449118,3.9172861393959,14.7433668292467));
#74640=CARTESIAN_POINT('Ctrl Pts',(7.21806243230082,3.73085275585992,14.7351446692391));
#74641=CARTESIAN_POINT('Ctrl Pts',(7.31440785713417,3.54445373745283,14.7269240248163));
#74642=CARTESIAN_POINT('Ctrl Pts',(7.40354001284765,3.35429954060967,14.7187033803934));
#74643=CARTESIAN_POINT('Ctrl Pts',(7.48518315744339,3.16096831082278,14.7104827359706));
#74644=CARTESIAN_POINT('Ctrl Pts',(7.56681712998245,2.96765880049569,14.7022630150817));
#74645=CARTESIAN_POINT('Ctrl Pts',(7.64096365630516,2.77117324157322,14.6940432941928));
#74646=CARTESIAN_POINT('Ctrl Pts',(7.70739490466815,2.5721102904027,14.6858235733039));
#74647=CARTESIAN_POINT('Ctrl Pts',(7.77383147591471,2.37303138907409,14.6776031938));
#74648=CARTESIAN_POINT('Ctrl Pts',(7.83255143796145,2.17137496196681,14.6693828142961));
#74649=CARTESIAN_POINT('Ctrl Pts',(7.88337632879413,1.96775639272456,14.6611624347922));
#74650=CARTESIAN_POINT('Ctrl Pts',(7.93420103153772,1.76413857701921,14.6529420857097));
#74651=CARTESIAN_POINT('Ctrl Pts',(7.9771306526257,1.55855892070873,14.6447217366271));
#74652=CARTESIAN_POINT('Ctrl Pts',(8.01203738140362,1.35164513149385,14.6365013875446));
#74653=CARTESIAN_POINT('Ctrl Pts',(8.04695157370626,1.14468710134794,14.6282792808417));
#74654=CARTESIAN_POINT('Ctrl Pts',(8.07383939755248,0.936394659503291,14.6200571741388));
#74655=CARTESIAN_POINT('Ctrl Pts',(8.0926244887072,0.727403909307994,14.6118350674359));
#74656=CARTESIAN_POINT('Ctrl Pts',(8.10086277041895,0.635750125939142,14.6082292275321));
#74657=CARTESIAN_POINT('Ctrl Pts',(8.10754332577607,0.543962114232721,14.6046233876282));
#74658=CARTESIAN_POINT('Ctrl Pts',(8.11266286535577,0.452093790686792,14.6010175477244));
#74659=CARTESIAN_POINT('Ctrl Pts',(8.12433661535909,0.242612483704973,14.5927953877168));
#74660=CARTESIAN_POINT('Ctrl Pts',(8.12789426530707,0.0326442164661224,
14.5845732277093));
#74661=CARTESIAN_POINT('Ctrl Pts',(8.12331816930504,-0.17717077281155,14.5763510677017));
#74662=CARTESIAN_POINT('Ctrl Pts',(8.11874291681143,-0.386947087046077,
14.5681304232789));
#74663=CARTESIAN_POINT('Ctrl Pts',(8.10603691717088,-0.59656988478547,14.5599097788561));
#74664=CARTESIAN_POINT('Ctrl Pts',(8.08523463567595,-0.805399558334893,
14.5516891344332));
#74665=CARTESIAN_POINT('Ctrl Pts',(8.06443469117703,-1.01420577127899,14.5434694135444));
#74666=CARTESIAN_POINT('Ctrl Pts',(8.03554030994549,-1.22221874434522,14.5352496926555));
#74667=CARTESIAN_POINT('Ctrl Pts',(7.99863784151324,-1.42880378037446,14.5270299717666));
#74668=CARTESIAN_POINT('Ctrl Pts',(7.96173241622641,-1.63540536927775,14.5188095922627));
#74669=CARTESIAN_POINT('Ctrl Pts',(7.91681767085712,-1.8405785014969,14.5105892127588));
#74670=CARTESIAN_POINT('Ctrl Pts',(7.86403131061546,-2.04369741110557,14.502368833255));
#74671=CARTESIAN_POINT('Ctrl Pts',(7.81124514572172,-2.24681556902657,14.4941484841725));
#74672=CARTESIAN_POINT('Ctrl Pts',(7.75058750104723,-2.44787923456029,14.4859281350899));
#74673=CARTESIAN_POINT('Ctrl Pts',(7.68224645627633,-2.64627605278243,14.4777077860074));
#74674=CARTESIAN_POINT('Ctrl Pts',(7.61389079927753,-2.8447152908934,14.4694856793046));
#74675=CARTESIAN_POINT('Ctrl Pts',(7.53784855630371,-3.04048626342017,14.4612635726017));
#74676=CARTESIAN_POINT('Ctrl Pts',(7.45435700021095,-3.23299385645968,14.4530414658988));
#74677=CARTESIAN_POINT('Ctrl Pts',(7.4177414227828,-3.31741888107669,14.4494356259948));
#74678=CARTESIAN_POINT('Ctrl Pts',(7.37969374624601,-3.40121651364254,14.4458297860909));
#74679=CARTESIAN_POINT('Ctrl Pts',(7.34023687728884,-3.48433783491053,14.4422239461869));
#74680=CARTESIAN_POINT('Ctrl Pts',(7.25026596937137,-3.67387392683657,14.4340017861793));
#74681=CARTESIAN_POINT('Ctrl Pts',(7.15293512516094,-3.85995465363508,14.4257796261718));
#74682=CARTESIAN_POINT('Ctrl Pts',(7.04853515787065,-4.04200936302248,14.4175574661642));
#74683=CARTESIAN_POINT('Ctrl Pts',(6.9441544345498,-4.22403051439873,14.4093368217414));
#74684=CARTESIAN_POINT('Ctrl Pts',(6.83270733559829,-4.40202687361533,14.4011161773185));
#74685=CARTESIAN_POINT('Ctrl Pts',(6.71453013276911,-4.57545327357144,14.3928955328957));
#74686=CARTESIAN_POINT('Ctrl Pts',(6.59636620635165,-4.74886019024114,14.3846758120068));
#74687=CARTESIAN_POINT('Ctrl Pts',(6.47147385165479,-4.91769792882157,14.3764560911179));
#74688=CARTESIAN_POINT('Ctrl Pts',(6.34023255200054,-5.08145045720734,14.368236370229));
#74689=CARTESIAN_POINT('Ctrl Pts',(6.2089807364795,-5.24521610646116,14.3600159907251));
#74690=CARTESIAN_POINT('Ctrl Pts',(6.07137914198951,-5.40389549935813,14.3517956112212));
#74691=CARTESIAN_POINT('Ctrl Pts',(5.92784807566002,-5.55700501658886,14.3435752317173));
#74692=CARTESIAN_POINT('Ctrl Pts',(5.78431754049983,-5.71011396720306,14.3353548826348));
#74693=CARTESIAN_POINT('Ctrl Pts',(5.63485778119669,-5.85765286988468,14.3271345335523));
#74694=CARTESIAN_POINT('Ctrl Pts',(5.479926923815,-5.99917398248688,14.3189141844698));
#74695=CARTESIAN_POINT('Ctrl Pts',(5.32496294014724,-6.14072535419265,14.3106920777669));
#74696=CARTESIAN_POINT('Ctrl Pts',(5.1645257393401,-6.27625616617983,14.302469971064));
#74697=CARTESIAN_POINT('Ctrl Pts',(4.99910839666797,-6.40535735153503,14.294247864361));
#74698=CARTESIAN_POINT('Ctrl Pts',(4.92656391670038,-6.4619752260789,14.2906420244572));
#74699=CARTESIAN_POINT('Ctrl Pts',(4.85306203549236,-6.51735701344645,14.2870361845533));
#74700=CARTESIAN_POINT('Ctrl Pts',(4.77864627239451,-6.57147071558795,14.2834303446494));
#74701=CARTESIAN_POINT('Ctrl Pts',(4.60896089323568,-6.69486263798879,14.2752081846418));
#74702=CARTESIAN_POINT('Ctrl Pts',(4.43446570784709,-6.81169910659657,14.2669860246343));
#74703=CARTESIAN_POINT('Ctrl Pts',(4.25568910354683,-6.92161815014761,14.2587638646267));
#74704=CARTESIAN_POINT('Ctrl Pts',(4.07694545300695,-7.03151693240194,14.2505432202039));
#74705=CARTESIAN_POINT('Ctrl Pts',(3.8939222099668,-7.13450067998437,14.242322575781));
#74706=CARTESIAN_POINT('Ctrl Pts',(3.70717548723022,-7.23025154952298,14.2341019313582));
#74707=CARTESIAN_POINT('Ctrl Pts',(3.52044974422825,-7.32599166209726,14.2258822104693));
#74708=CARTESIAN_POINT('Ctrl Pts',(3.33000161918168,-7.41450038424945,14.2176624895804));
#74709=CARTESIAN_POINT('Ctrl Pts',(3.13641123107975,-7.49550613047957,14.2094427686915));
#74710=CARTESIAN_POINT('Ctrl Pts',(2.94280533131564,-7.57651836739233,14.2012223891876));
#74711=CARTESIAN_POINT('Ctrl Pts',(2.74605693664309,-7.65002631070526,14.1930020096837));
#74712=CARTESIAN_POINT('Ctrl Pts',(2.54676650728578,-7.71580636873861,14.1847816301798));
#74713=CARTESIAN_POINT('Ctrl Pts',(2.34747681544809,-7.78158618333789,14.1765612810973));
#74714=CARTESIAN_POINT('Ctrl Pts',(2.14564538885169,-7.83963807989123,14.1683409320148));
#74715=CARTESIAN_POINT('Ctrl Pts',(1.9418887328439,-7.88978806507208,14.1601205829323));
#74716=CARTESIAN_POINT('Ctrl Pts',(1.7380885109424,-7.9399487729894,14.1518984762294));
#74717=CARTESIAN_POINT('Ctrl Pts',(1.53236252390231,-7.98220412362127,14.1436763695265));
#74718=CARTESIAN_POINT('Ctrl Pts',(1.32533946353552,-8.01643080609415,14.1354542628236));
#74719=CARTESIAN_POINT('Ctrl Pts',(1.23454861891719,-8.03144106342824,14.1318484229197));
#74720=CARTESIAN_POINT('Ctrl Pts',(1.14350843511523,-8.04490783165832,14.1282425830158));
#74721=CARTESIAN_POINT('Ctrl Pts',(1.05227243640835,-8.05682383337722,14.1246367431119));
#74722=CARTESIAN_POINT('Ctrl Pts',(0.844232978248779,-8.083995109805,14.1164145831043));
#74723=CARTESIAN_POINT('Ctrl Pts',(0.635106222316402,-8.10310871945177,
14.1081924230968));
#74724=CARTESIAN_POINT('Ctrl Pts',(0.425529336930057,-8.11409960167558,
14.0999702630892));
#74725=CARTESIAN_POINT('Ctrl Pts',(0.215991082697217,-8.12508845795814,
14.0917496186663));
#74726=CARTESIAN_POINT('Ctrl Pts',(0.00600315920071098,-8.12795755968557,
14.0835289742435));
#74727=CARTESIAN_POINT('Ctrl Pts',(-0.203794030827732,-8.12269386075205,
14.0753083298207));
#74728=CARTESIAN_POINT('Ctrl Pts',(-0.413567651556558,-8.1174307531596,
14.0670886089318));
#74729=CARTESIAN_POINT('Ctrl Pts',(-0.623150286661849,-8.10403667637436,
14.0588688880429));
#74730=CARTESIAN_POINT('Ctrl Pts',(-0.831902584058519,-8.08255068979692,
14.050649167154));
#74731=CARTESIAN_POINT('Ctrl Pts',(-1.04067160798393,-8.06106298162899,
14.0424287876501));
#74732=CARTESIAN_POINT('Ctrl Pts',(-1.24860986738173,-8.03148209565615,
14.0342084081462));
#74733=CARTESIAN_POINT('Ctrl Pts',(-1.45508310963106,-7.99389896774824,
14.0259880286423));
#74734=CARTESIAN_POINT('Ctrl Pts',(-1.66155558777939,-7.95631597892521,
14.0177676795598));
#74735=CARTESIAN_POINT('Ctrl Pts',(-1.86656276972992,-7.91073086288741,
14.0095473304773));
#74736=CARTESIAN_POINT('Ctrl Pts',(-2.06948004250879,-7.85728578557238,
14.0013269813948));
#74737=CARTESIAN_POINT('Ctrl Pts',(-2.27244070170992,-7.80382928098623,
13.9931048746919));
#74738=CARTESIAN_POINT('Ctrl Pts',(-2.47331027355075,-7.74250953286885,
13.984882767989));
#74739=CARTESIAN_POINT('Ctrl Pts',(-2.6714776917589,-7.67351904310757,13.9766606612861));
#74740=CARTESIAN_POINT('Ctrl Pts',(-2.75838485680127,-7.64326297006462,
13.9730548213822));
#74741=CARTESIAN_POINT('Ctrl Pts',(-2.84477252316002,-7.61153222764843,
13.9694489814783));
#74742=CARTESIAN_POINT('Ctrl Pts',(-2.93059020803915,-7.57834603294446,
13.9658431415744));
#74743=CARTESIAN_POINT('Ctrl Pts',(-3.12627464089316,-7.50267373185202,
13.9576209815668));
#74744=CARTESIAN_POINT('Ctrl Pts',(-3.31905883691528,-7.41940558737523,
13.9493988215593));
#74745=CARTESIAN_POINT('Ctrl Pts',(-3.50835215499058,-7.32878930786477,
13.9411766615517));
#74746=CARTESIAN_POINT('Ctrl Pts',(-3.69761058076738,-7.23818973158665,
13.9329560171288));
#74747=CARTESIAN_POINT('Ctrl Pts',(-3.88337914679839,-7.14024485099647,
13.924735372706));
#74748=CARTESIAN_POINT('Ctrl Pts',(-4.06508925700879,-7.03524959721059,
13.9165147282832));
#74749=CARTESIAN_POINT('Ctrl Pts',(-4.24677895331354,-6.9302661389335,13.9082950073943));
#74750=CARTESIAN_POINT('Ctrl Pts',(-4.42441084860086,-6.81823403635945,
13.9000752865054));
#74751=CARTESIAN_POINT('Ctrl Pts',(-4.59744219818209,-6.6994934731571,13.8918555656165));
#74752=CARTESIAN_POINT('Ctrl Pts',(-4.77048741210823,-6.58074339572437,
13.8836351861126));
#74753=CARTESIAN_POINT('Ctrl Pts',(-4.93893109887327,-6.4552839483907,13.8754148066088));
#74754=CARTESIAN_POINT('Ctrl Pts',(-5.10225981096964,-6.32349842918175,
13.8671944271049));
#74755=CARTESIAN_POINT('Ctrl Pts',(-5.26558791863134,-6.19171339767478,
13.8589740780223));
#74756=CARTESIAN_POINT('Ctrl Pts',(-5.42380086146933,-6.05360252853669,
13.8507537289398));
#74757=CARTESIAN_POINT('Ctrl Pts',(-5.57641816675348,-5.90958949437283,
13.8425333798573));
#74758=CARTESIAN_POINT('Ctrl Pts',(-5.72906810365512,-5.76554566829952,
13.8343112731544));
#74759=CARTESIAN_POINT('Ctrl Pts',(-5.87611979807905,-5.61559735864673,
13.8260891664515));
#74760=CARTESIAN_POINT('Ctrl Pts',(-6.01712875518766,-5.46020595820284,
13.8178670597486));
#74761=CARTESIAN_POINT('Ctrl Pts',(-6.07896883373719,-5.39205839788885,
13.8142612198446));
#74762=CARTESIAN_POINT('Ctrl Pts',(-6.1396472022574,-5.32286443495135,13.8106553799407));
#74763=CARTESIAN_POINT('Ctrl Pts',(-6.19912872449189,-5.25266509685127,
13.8070495400368));
#74764=CARTESIAN_POINT('Ctrl Pts',(-6.33476053464949,-5.09259415480571,
13.7988273800293));
#74765=CARTESIAN_POINT('Ctrl Pts',(-6.46421149893803,-4.92724066084432,
13.7906052200217));
#74766=CARTESIAN_POINT('Ctrl Pts',(-6.58708147076001,-4.75710471401147,
13.7823830600141));
#74767=CARTESIAN_POINT('Ctrl Pts',(-6.70992879405006,-4.5870001282131,13.7741624155913));
#74768=CARTESIAN_POINT('Ctrl Pts',(-6.82619737328195,-4.41211508813729,
13.7659417711685));
#74769=CARTESIAN_POINT('Ctrl Pts',(-6.93552901292721,-4.2329806133911,13.7577211267457));
#74770=CARTESIAN_POINT('Ctrl Pts',(-7.0448483699003,-4.05386626319472,13.7495014058568));
#74771=CARTESIAN_POINT('Ctrl Pts',(-7.14723218944189,-3.87050368324245,
13.7412816849679));
#74772=CARTESIAN_POINT('Ctrl Pts',(-7.24236662693766,-3.68345126254165,
13.733061964079));
#74773=CARTESIAN_POINT('Ctrl Pts',(-7.33750868719447,-3.49638385404102,
13.7248415845751));
#74774=CARTESIAN_POINT('Ctrl Pts',(-7.42540006854169,-3.30562627589227,
13.7166212050712));
#74775=CARTESIAN_POINT('Ctrl Pts',(-7.50577328014737,-3.11176076032941,
13.7084008255673));
#74776=CARTESIAN_POINT('Ctrl Pts',(-7.58614619431361,-2.91789596221019,
13.7001804764848));
#74777=CARTESIAN_POINT('Ctrl Pts',(-7.65900088382745,-2.72092352334852,
13.6919601274023));
#74778=CARTESIAN_POINT('Ctrl Pts',(-7.72411813024424,-2.52144535386596,
13.6837397783198));
#74779=CARTESIAN_POINT('Ctrl Pts',(-7.78924929959781,-2.32192453328716,
13.6755176716169));
#74780=CARTESIAN_POINT('Ctrl Pts',(-7.84663962913896,-2.11989719237576,
13.667295564914));
#74781=CARTESIAN_POINT('Ctrl Pts',(-7.8961195399841,-1.91598115146818,13.6590734582111));
#74782=CARTESIAN_POINT('Ctrl Pts',(-7.91781916556865,-1.82655290346206,
13.6554676183072));
#74783=CARTESIAN_POINT('Ctrl Pts',(-7.93799803372971,-1.73676157763822,
13.6518617784032));
#74784=CARTESIAN_POINT('Ctrl Pts',(-7.95664491912623,-1.64666001149077,
13.6482559384993));
#74785=CARTESIAN_POINT('Ctrl Pts',(-8.00016030884298,-1.43639407797839,
13.6398411536524));
#74786=CARTESIAN_POINT('Ctrl Pts',(-8.03534067518961,-1.22438249265304,
13.6314263688055));
#74787=CARTESIAN_POINT('Ctrl Pts',(-8.06207098145817,-1.01128584111026,
13.6230115839586));
#74788=CARTESIAN_POINT('Ctrl Pts',(-8.08879423962124,-0.798245377763173,
13.6145990178776));
#74789=CARTESIAN_POINT('Ctrl Pts',(-8.10707185453581,-0.584120681911771,
13.6061864517965));
#74790=CARTESIAN_POINT('Ctrl Pts',(-8.11684044199827,-0.369579222415569,
13.5977738857155));
#74791=CARTESIAN_POINT('Ctrl Pts',(-8.12244374199678,-0.246517401625759,
13.5929484048883));
#74792=CARTESIAN_POINT('Ctrl Pts',(-8.1252483419671,-0.12331857197614,13.588122924061));
#74793=CARTESIAN_POINT('Ctrl Pts',(-8.12524999926494,-0.000109293386091071,
13.5832974432338));
#74794=CARTESIAN_POINT('Origin',(0.,0.,24.4167025567876));
#74795=CARTESIAN_POINT('',(4.94675954817621,6.44587135576157,16.8749477411846));
#74796=CARTESIAN_POINT('',(4.94678612080823,6.44590587665303,16.7083566551695));
#74797=CARTESIAN_POINT('',(4.9467595481762,6.44587135576158,24.4167025567876));
#74798=CARTESIAN_POINT('',(-8.12525198907861,0.000116094565966279,15.4167025568297));
#74799=CARTESIAN_POINT('Ctrl Pts',(4.94678612080823,6.44590587665303,16.7083566551695));
#74800=CARTESIAN_POINT('Ctrl Pts',(5.18341558504802,6.26470660955122,16.6966804905928));
#74801=CARTESIAN_POINT('Ctrl Pts',(6.43739680606016,5.19025029452804,16.6320731255035));
#74802=CARTESIAN_POINT('Ctrl Pts',(8.07312723790633,2.56246057378528,16.5145345599018));
#74803=CARTESIAN_POINT('Ctrl Pts',(8.31518029376954,-1.61225440732664,16.3557409583643));
#74804=CARTESIAN_POINT('Ctrl Pts',(6.53042868202404,-5.39398635712584,16.1969473568268));
#74805=CARTESIAN_POINT('Ctrl Pts',(3.15390120175042,-7.86094744934625,16.0381537552892));
#74806=CARTESIAN_POINT('Ctrl Pts',(-0.991381909914889,-8.41182200837257,
15.8793601537517));
#74807=CARTESIAN_POINT('Ctrl Pts',(-4.89501812861923,-6.91233572045668,
15.7205665522142));
#74808=CARTESIAN_POINT('Ctrl Pts',(-7.52742407670693,-3.81971705372047,
15.5663473571833));
#74809=CARTESIAN_POINT('Ctrl Pts',(-8.12495145299739,-1.23397979003354,
15.4650593626648));
#74810=CARTESIAN_POINT('Ctrl Pts',(-8.12581156037035,0.000115800672715422,
15.4167025686589));
#74811=CARTESIAN_POINT('Ctrl Pts',(-8.1252499991706,0.000116095611088758,
15.4167025567876));
#74812=CARTESIAN_POINT('Ctrl Pts',(-8.12524833125246,0.116849637214079,
15.4121281542381));
#74813=CARTESIAN_POINT('Ctrl Pts',(-8.12273074956299,0.233575803540142,
15.4075537516886));
#74814=CARTESIAN_POINT('Ctrl Pts',(-8.11769993863055,0.350193187908608,
15.4029793491391));
#74815=CARTESIAN_POINT('Ctrl Pts',(-8.10865741733798,0.559804559792054,
15.3947571891316));
#74816=CARTESIAN_POINT('Ctrl Pts',(-8.09149033708956,0.769100095999624,
15.386535029124));
#74817=CARTESIAN_POINT('Ctrl Pts',(-8.06624427927133,0.977440939199128,
15.3783128691164));
#74818=CARTESIAN_POINT('Ctrl Pts',(-8.04100287504045,1.18574337908361,15.3700922246936));
#74819=CARTESIAN_POINT('Ctrl Pts',(-8.00768550094828,1.39309118433539,15.3618715802707));
#74820=CARTESIAN_POINT('Ctrl Pts',(-7.96638953334373,1.59885126435561,15.3536509358479));
#74821=CARTESIAN_POINT('Ctrl Pts',(-7.92509820506246,1.80458822861932,15.3454312149589));
#74822=CARTESIAN_POINT('Ctrl Pts',(-7.87583013080488,2.00873753449623,15.33721149407));
#74823=CARTESIAN_POINT('Ctrl Pts',(-7.81873383394003,2.21067609488622,15.3289917731811));
#74824=CARTESIAN_POINT('Ctrl Pts',(-7.76163296216609,2.41263083584496,15.3207713936772));
#74825=CARTESIAN_POINT('Ctrl Pts',(-7.69670269216183,2.61237419261429,15.3125510141733));
#74826=CARTESIAN_POINT('Ctrl Pts',(-7.62414177180475,2.80929703056155,15.3043306346694));
#74827=CARTESIAN_POINT('Ctrl Pts',(-7.55158111997556,3.00621913975188,15.2961102855869));
#74828=CARTESIAN_POINT('Ctrl Pts',(-7.47138997883233,3.20032047498142,15.2878899365044));
#74829=CARTESIAN_POINT('Ctrl Pts',(-7.38381590253885,3.39101021524773,15.2796695874218));
#74830=CARTESIAN_POINT('Ctrl Pts',(-7.29622310173865,3.58174072752639,15.2714474807189));
#74831=CARTESIAN_POINT('Ctrl Pts',(-7.2012443353129,3.7690579192871,15.263225374016));
#74832=CARTESIAN_POINT('Ctrl Pts',(-7.09917441044576,3.9523929780036,15.2550032673131));
#74833=CARTESIAN_POINT('Ctrl Pts',(-7.05441121028773,4.03279534863327,15.2513974274093));
#74834=CARTESIAN_POINT('Ctrl Pts',(-7.00828476682951,4.11243214996698,15.2477915875055));
#74835=CARTESIAN_POINT('Ctrl Pts',(-6.96082269957941,4.19125696033064,15.2441857476017));
#74836=CARTESIAN_POINT('Ctrl Pts',(-6.8525980635358,4.37099600051744,15.2359635875941));
#74837=CARTESIAN_POINT('Ctrl Pts',(-6.73739014407924,4.5465706724238,15.2277414275865));
#74838=CARTESIAN_POINT('Ctrl Pts',(-6.61554461530079,4.71744178612357,15.219519267579));
#74839=CARTESIAN_POINT('Ctrl Pts',(-6.49372154621956,4.88828140327589,15.2112986231561));
#74840=CARTESIAN_POINT('Ctrl Pts',(-6.36526348103575,5.05441895245761,15.2030779787333));
#74841=CARTESIAN_POINT('Ctrl Pts',(-6.2305588173836,5.21534508787516,15.1948573343105));
#74842=CARTESIAN_POINT('Ctrl Pts',(-6.09586928689129,5.37625314432747,15.1866376134216));
#74843=CARTESIAN_POINT('Ctrl Pts',(-5.95493474832005,5.53195072962859,15.1784178925327));
#74844=CARTESIAN_POINT('Ctrl Pts',(-5.80818372688031,5.68196175253783,15.1701981716438));
#74845=CARTESIAN_POINT('Ctrl Pts',(-5.66142094683921,5.83198479525995,15.1619777921399));
#74846=CARTESIAN_POINT('Ctrl Pts',(-5.50884095715798,5.97632015227656,15.153757412636));
#74847=CARTESIAN_POINT('Ctrl Pts',(-5.35090971124037,6.11452801323647,15.1455370331321));
#74848=CARTESIAN_POINT('Ctrl Pts',(-5.19297904978318,6.25273536272681,15.1373166840496));
#74849=CARTESIAN_POINT('Ctrl Pts',(-5.02969739556781,6.38481506916211,15.1290963349671));
#74850=CARTESIAN_POINT('Ctrl Pts',(-4.86156479830643,6.51036675421345,15.1208759858846));
#74851=CARTESIAN_POINT('Ctrl Pts',(-4.69339625205083,6.63594528389144,15.1126538791817));
#74852=CARTESIAN_POINT('Ctrl Pts',(-4.52037492716479,6.75499282706329,15.1044317724788));
#74853=CARTESIAN_POINT('Ctrl Pts',(-4.34303183798392,6.86715093883614,15.0962096657759));
#74854=CARTESIAN_POINT('Ctrl Pts',(-4.26525727110475,6.91633835631831,15.0926038258719));
#74855=CARTESIAN_POINT('Ctrl Pts',(-4.18665187507912,6.96420129217655,15.088997985968));
#74856=CARTESIAN_POINT('Ctrl Pts',(-4.10726211279737,7.01071219629499,15.0853921460641));
#74857=CARTESIAN_POINT('Ctrl Pts',(-3.9262348498468,7.11676795749043,15.0771699860565));
#74858=CARTESIAN_POINT('Ctrl Pts',(-3.74106773711732,7.21582587228796,15.068947826049));
#74859=CARTESIAN_POINT('Ctrl Pts',(-3.55232228419872,7.3075778443808,15.0607256660414));
#74860=CARTESIAN_POINT('Ctrl Pts',(-3.36361162259147,7.39931290389971,15.0525050216186));
#74861=CARTESIAN_POINT('Ctrl Pts',(-3.17132420255942,7.48374457956918,15.0442843771957));
#74862=CARTESIAN_POINT('Ctrl Pts',(-2.97604477205769,7.56061142218062,15.0360637327729));
#74863=CARTESIAN_POINT('Ctrl Pts',(-2.7807872798827,7.63746962932082,15.027844011884));
#74864=CARTESIAN_POINT('Ctrl Pts',(-2.58253872282732,7.70676459202466,15.0196242909951));
#74865=CARTESIAN_POINT('Ctrl Pts',(-2.38190317598133,7.76828326097536,15.0114045701062));
#74866=CARTESIAN_POINT('Ctrl Pts',(-2.18125155297117,7.8298068591833,15.0031841906024));
#74867=CARTESIAN_POINT('Ctrl Pts',(-1.97821283939896,7.88355282951826,14.9949638110985));
#74868=CARTESIAN_POINT('Ctrl Pts',(-1.77340661920289,7.92935788859775,14.9867434315946));
#74869=CARTESIAN_POINT('Ctrl Pts',(-1.56860115693872,7.97516277816522,14.9785230825121));
#74870=CARTESIAN_POINT('Ctrl Pts',(-1.36202848974609,8.01302675344973,14.9703027334295));
#74871=CARTESIAN_POINT('Ctrl Pts',(-1.15431927700282,8.04283747002509,14.962082384347));
#74872=CARTESIAN_POINT('Ctrl Pts',(-0.946565653256594,8.07265456052969,
14.9538602776441));
#74873=CARTESIAN_POINT('Ctrl Pts',(-0.73767529068533,8.09441491037672,14.9456381709412));
#74874=CARTESIAN_POINT('Ctrl Pts',(-0.528285977342776,8.10805781236438,
14.9374160642383));
#74875=CARTESIAN_POINT('Ctrl Pts',(-0.436457402406439,8.1140409651219,14.9338102243344));
#74876=CARTESIAN_POINT('Ctrl Pts',(-0.344532925030685,8.11846356305347,
14.9302043844305));
#74877=CARTESIAN_POINT('Ctrl Pts',(-0.252566526273103,8.12132364287413,
14.9265985445266));
#74878=CARTESIAN_POINT('Ctrl Pts',(-0.0428615848291338,8.12784529512343,
14.918376384519));
#74879=CARTESIAN_POINT('Ctrl Pts',(0.167130694596802,8.12624133064013,14.9101542245115));
#74880=CARTESIAN_POINT('Ctrl Pts',(0.376769833492397,8.11650984445101,14.9019320645039));
#74881=CARTESIAN_POINT('Ctrl Pts',(0.58637032975894,8.10678015205961,14.8937114200811));
#74882=CARTESIAN_POINT('Ctrl Pts',(0.795617520736961,8.08892594172221,14.8854907756582));
#74883=CARTESIAN_POINT('Ctrl Pts',(1.00387283902084,8.06299738841433,14.8772701312354));
#74884=CARTESIAN_POINT('Ctrl Pts',(1.21210476122435,8.03707174800452,14.8690504103465));
#74885=CARTESIAN_POINT('Ctrl Pts',(1.41934474042965,8.00307361203196,14.8608306894576));
#74886=CARTESIAN_POINT('Ctrl Pts',(1.6249603934794,7.96110490334874,14.8526109685688));
#74887=CARTESIAN_POINT('Ctrl Pts',(1.83059252173041,7.9191328318723,14.8443905890649));
#74888=CARTESIAN_POINT('Ctrl Pts',(2.03459977403428,7.86918896794758,14.836170209561));
#74889=CARTESIAN_POINT('Ctrl Pts',(2.23635995797362,7.81142635508216,14.8279498300571));
#74890=CARTESIAN_POINT('Ctrl Pts',(2.43811939525372,7.75366395598037,14.8197294809746));
#74891=CARTESIAN_POINT('Ctrl Pts',(2.6376314977942,7.68808294961918,14.8115091318921));
#74892=CARTESIAN_POINT('Ctrl Pts',(2.83428871821796,7.61488640915164,14.8032887828095));
#74893=CARTESIAN_POINT('Ctrl Pts',(3.03098798658119,7.54167421828644,14.7950666761066));
#74894=CARTESIAN_POINT('Ctrl Pts',(3.22483087668187,7.46084334325658,14.7868445694037));
#74895=CARTESIAN_POINT('Ctrl Pts',(3.41522828601163,7.37264561178184,14.7786224627008));
#74896=CARTESIAN_POINT('Ctrl Pts',(3.49872788057658,7.33396612110172,14.7750166227969));
#74897=CARTESIAN_POINT('Ctrl Pts',(3.58156507489106,7.29387038377963,14.771410782893));
#74898=CARTESIAN_POINT('Ctrl Pts',(3.66369152747975,7.25238250190743,14.7678049429891));
#74899=CARTESIAN_POINT('Ctrl Pts',(3.8509572389557,7.15778134148305,14.7595828640634));
#74900=CARTESIAN_POINT('Ctrl Pts',(4.03458781042971,7.05590753652313,14.7513607851376));
#74901=CARTESIAN_POINT('Ctrl Pts',(4.21401992606655,6.94706582847853,14.7431387062119));
#74902=CARTESIAN_POINT('Ctrl Pts',(4.39342133299661,6.83824274802512,14.7349180344446));
#74903=CARTESIAN_POINT('Ctrl Pts',(4.56862546571034,6.72245429712697,14.7266973626773));
#74904=CARTESIAN_POINT('Ctrl Pts',(4.73909558099361,6.60005004804561,14.71847669091));
#74905=CARTESIAN_POINT('Ctrl Pts',(4.8091274599213,6.54976440391581,14.7150995060647));
#74906=CARTESIAN_POINT('Ctrl Pts',(4.87836070806544,6.49836272531081,14.7117223212193));
#74907=CARTESIAN_POINT('Ctrl Pts',(4.94675954817621,6.44587135576157,14.708345136374));
#74908=CARTESIAN_POINT('',(-8.1252499975661,0.000198877198026241,15.5832974432373));
#74909=CARTESIAN_POINT('Ctrl Pts',(-8.12524999756608,0.000198877834300525,
15.5832974432124));
#74910=CARTESIAN_POINT('Ctrl Pts',(-8.12524452136295,0.223931802217315,
15.5745316392917));
#74911=CARTESIAN_POINT('Ctrl Pts',(-8.11599380670282,0.447621544553009,
15.565765835371));
#74912=CARTESIAN_POINT('Ctrl Pts',(-8.09753449887972,0.670539038351091,
15.5570000314503));
#74913=CARTESIAN_POINT('Ctrl Pts',(-8.09527362566499,0.697841697565204,
15.5559264066167));
#74914=CARTESIAN_POINT('Ctrl Pts',(-8.09287467794545,0.725132776551766,
15.5548527817831));
#74915=CARTESIAN_POINT('Ctrl Pts',(-8.09033777663931,0.752410939834638,
15.5537791569495));
#74916=CARTESIAN_POINT('Ctrl Pts',(-8.07090938060148,0.961315779042493,
15.5455569969417));
#74917=CARTESIAN_POINT('Ctrl Pts',(-8.04338209203338,1.16950218231516,15.5373348369338));
#74918=CARTESIAN_POINT('Ctrl Pts',(-8.0078331243954,1.37633433959039,15.529112676926));
#74919=CARTESIAN_POINT('Ctrl Pts',(-7.97229070947257,1.58312837164571,15.5208920325029));
#74920=CARTESIAN_POINT('Ctrl Pts',(-7.92872961659068,1.78856836519349,15.5126713880798));
#74921=CARTESIAN_POINT('Ctrl Pts',(-7.87727850438065,1.99202683890617,15.5044507436566));
#74922=CARTESIAN_POINT('Ctrl Pts',(-7.82583317235589,2.19546245543225,15.4962310227675));
#74923=CARTESIAN_POINT('Ctrl Pts',(-7.76649966294933,2.39691671052598,15.4880113018783));
#74924=CARTESIAN_POINT('Ctrl Pts',(-7.69945722266801,2.59577465100602,15.4797915809891));
#74925=CARTESIAN_POINT('Ctrl Pts',(-7.63240941053079,2.79464852521692,15.4715712014849));
#74926=CARTESIAN_POINT('Ctrl Pts',(-7.5576515250233,2.99092538858532,15.4633508219807));
#74927=CARTESIAN_POINT('Ctrl Pts',(-7.47541228327836,3.18400671442617,15.4551304424766));
#74928=CARTESIAN_POINT('Ctrl Pts',(-7.39317334587837,3.37708732572584,15.4469100933938));
#74929=CARTESIAN_POINT('Ctrl Pts',(-7.30345322573677,3.56697215266104,15.438689744311));
#74930=CARTESIAN_POINT('Ctrl Pts',(-7.20652847781618,3.75308338049189,15.4304693952282));
#74931=CARTESIAN_POINT('Ctrl Pts',(-7.10958300609048,3.93923440138795,15.422247288525));
#74932=CARTESIAN_POINT('Ctrl Pts',(-7.00542996543054,4.12160994943329,15.4140251818218));
#74933=CARTESIAN_POINT('Ctrl Pts',(-6.89439201400549,4.2996565350871,15.4058030751186));
#74934=CARTESIAN_POINT('Ctrl Pts',(-6.84569584763828,4.37773962330011,15.4021972352164));
#74935=CARTESIAN_POINT('Ctrl Pts',(-6.79567608925784,4.4549904658639,15.3985913953142));
#74936=CARTESIAN_POINT('Ctrl Pts',(-6.7443626269528,4.53136406820974,15.394985555412));
#74937=CARTESIAN_POINT('Ctrl Pts',(-6.62735590756068,4.70551377975176,15.3867633954045));
#74938=CARTESIAN_POINT('Ctrl Pts',(-6.50358105876076,4.87515786872667,15.3785412353971));
#74939=CARTESIAN_POINT('Ctrl Pts',(-6.37341007369604,5.03977495479806,15.3703190753896));
#74940=CARTESIAN_POINT('Ctrl Pts',(-6.24326308295346,5.2043616971228,15.3620984309668));
#74941=CARTESIAN_POINT('Ctrl Pts',(-6.10672249203103,5.36392305456479,15.3538777865441));
#74942=CARTESIAN_POINT('Ctrl Pts',(-5.96420148471735,5.51796957332998,15.3456571421213));
#74943=CARTESIAN_POINT('Ctrl Pts',(-5.82169648867807,5.67199878600723,15.3374374212325));
#74944=CARTESIAN_POINT('Ctrl Pts',(-5.67321261792456,5.82051418034593,15.3292177003437));
#74945=CARTESIAN_POINT('Ctrl Pts',(-5.51920148495797,5.9630615065533,15.320997979455));
#74946=CARTESIAN_POINT('Ctrl Pts',(-5.36517801166409,6.10562025453666,15.3127775999512));
#74947=CARTESIAN_POINT('Ctrl Pts',(-5.20562660599788,6.24220977640885,15.3045572204474));
#74948=CARTESIAN_POINT('Ctrl Pts',(-5.04103446300252,6.37241391509692,15.2963368409436));
#74949=CARTESIAN_POINT('Ctrl Pts',(-4.87644292911781,6.50261757193497,15.2881164918612));
#74950=CARTESIAN_POINT('Ctrl Pts',(-4.70681092834914,6.62643571184036,15.2798961427787));
#74951=CARTESIAN_POINT('Ctrl Pts',(-4.53265775419765,6.74349325244802,15.2716757936963));
#74952=CARTESIAN_POINT('Ctrl Pts',(-4.35846734377206,6.86057582152092,15.2634536869935));
#74953=CARTESIAN_POINT('Ctrl Pts',(-4.17975407371267,6.97089473877623,15.2552315802907));
#74954=CARTESIAN_POINT('Ctrl Pts',(-3.99706608407484,7.07411833955572,15.2470094735879));
#74955=CARTESIAN_POINT('Ctrl Pts',(-3.91694748832893,7.11938748920636,15.2434036336834));
#74956=CARTESIAN_POINT('Ctrl Pts',(-3.83606478217253,7.16329257730237,15.239797793779));
#74957=CARTESIAN_POINT('Ctrl Pts',(-3.75446573782737,7.20580839226109,15.2361919538745));
#74958=CARTESIAN_POINT('Ctrl Pts',(-3.56840079405644,7.30275441391065,15.2279697938669));
#74959=CARTESIAN_POINT('Ctrl Pts',(-3.378548198833,7.3925058607378,15.2197476338593));
#74960=CARTESIAN_POINT('Ctrl Pts',(-3.18548405257249,7.47478286730166,15.2115254738518));
#74961=CARTESIAN_POINT('Ctrl Pts',(-2.99245549368421,7.55704470780534,15.2033048294289));
#74962=CARTESIAN_POINT('Ctrl Pts',(-2.79621683665351,7.63183474220884,15.195084185006));
#74963=CARTESIAN_POINT('Ctrl Pts',(-2.59736507789831,7.69892084740545,15.1868635405832));
#74964=CARTESIAN_POINT('Ctrl Pts',(-2.39853565879714,7.76599941593058,15.1786438196943));
#74965=CARTESIAN_POINT('Ctrl Pts',(-2.19709400359908,7.82537568881756,15.1704240988054));
#74966=CARTESIAN_POINT('Ctrl Pts',(-1.9936540113673,7.87686684192764,15.1622043779165));
#74967=CARTESIAN_POINT('Ctrl Pts',(-1.79019771826208,7.92836212082813,15.1539839984126));
#74968=CARTESIAN_POINT('Ctrl Pts',(-1.58474305364989,7.97197094247569,15.1457636189087));
#74969=CARTESIAN_POINT('Ctrl Pts',(-1.37791693789531,8.00756095666847,15.1375432394048));
#74970=CARTESIAN_POINT('Ctrl Pts',(-1.17109158754778,8.0431508391523,15.1293228903222));
#74971=CARTESIAN_POINT('Ctrl Pts',(-0.962895087532059,8.07072192612209,
15.1211025412397));
#74972=CARTESIAN_POINT('Ctrl Pts',(-0.753962893379013,8.09019329298797,
15.1128821921572));
#74973=CARTESIAN_POINT('Ctrl Pts',(-0.544986026733049,8.10966882309208,
15.1046600854543));
#74974=CARTESIAN_POINT('Ctrl Pts',(-0.335273445622575,8.12104114584314,
15.0964379787514));
#74975=CARTESIAN_POINT('Ctrl Pts',(-0.125465164204048,8.12428126390706,
15.0882158720484));
#74976=CARTESIAN_POINT('Ctrl Pts',(-0.0334528490363855,8.12570223148023,
15.0846100321446));
#74977=CARTESIAN_POINT('Ctrl Pts',(0.0585778449112692,8.12555980823119,
15.0810041922408));
#74978=CARTESIAN_POINT('Ctrl Pts',(0.150572905645268,8.12385471082451,15.077398352337));
#74979=CARTESIAN_POINT('Ctrl Pts',(0.360343203117682,8.11996668914849,15.0691761923294));
#74980=CARTESIAN_POINT('Ctrl Pts',(0.569997443396807,8.10794880024545,15.0609540323218));
#74981=CARTESIAN_POINT('Ctrl Pts',(0.778895841848721,8.08783091008033,15.0527318723142));
#74982=CARTESIAN_POINT('Ctrl Pts',(0.98775573421209,8.06771672823114,15.0445112278914));
#74983=CARTESIAN_POINT('Ctrl Pts',(1.19585976918339,8.03950555335458,15.0362905834685));
#74984=CARTESIAN_POINT('Ctrl Pts',(1.40257265411832,8.00327917246547,15.0280699390456));
#74985=CARTESIAN_POINT('Ctrl Pts',(1.60926231625469,7.96705686136594,15.0198502181567));
#74986=CARTESIAN_POINT('Ctrl Pts',(1.81456084977107,7.92282119287479,15.0116304972678));
#74987=CARTESIAN_POINT('Ctrl Pts',(2.01784170542331,7.87070533143976,15.0034107763789));
#74988=CARTESIAN_POINT('Ctrl Pts',(2.22113884919822,7.81858529415876,14.995190396875));
#74989=CARTESIAN_POINT('Ctrl Pts',(2.42241770549352,7.75858387296805,14.9869700173711));
#74990=CARTESIAN_POINT('Ctrl Pts',(2.6210644389143,7.69088478457186,14.9787496378672));
#74991=CARTESIAN_POINT('Ctrl Pts',(2.81971043719779,7.62318594671149,14.9705292887847));
#74992=CARTESIAN_POINT('Ctrl Pts',(3.01572405358715,7.5477895963651,14.9623089397021));
#74993=CARTESIAN_POINT('Ctrl Pts',(3.20850856123859,7.46492869188706,14.9540885906196));
#74994=CARTESIAN_POINT('Ctrl Pts',(3.40133428879183,7.38205007064129,14.9458664839167));
#74995=CARTESIAN_POINT('Ctrl Pts',(3.59092925705583,7.29170382329379,14.9376443772138));
#74996=CARTESIAN_POINT('Ctrl Pts',(3.77671757964361,7.19417068786326,14.9294222705108));
#74997=CARTESIAN_POINT('Ctrl Pts',(3.85819583959006,7.15139711602993,14.925816430607));
#74998=CARTESIAN_POINT('Ctrl Pts',(3.93894226690403,7.10724189675949,14.9222105907032));
#74999=CARTESIAN_POINT('Ctrl Pts',(4.01890977511006,7.06173150027844,14.9186047507994));
#75000=CARTESIAN_POINT('Ctrl Pts',(4.20125611213359,6.95795617601265,14.9103825151302));
#75001=CARTESIAN_POINT('Ctrl Pts',(4.37961089847017,6.8470971967438,14.9021602794609));
#75002=CARTESIAN_POINT('Ctrl Pts',(4.5534265962013,6.72948688946688,14.8939380437917));
#75003=CARTESIAN_POINT('Ctrl Pts',(4.6873097519285,6.63889645782107,14.8876047903923));
#75004=CARTESIAN_POINT('Ctrl Pts',(4.81850033447646,6.54430141354479,14.8812715369928));
#75005=CARTESIAN_POINT('Ctrl Pts',(4.94675954817619,6.44587135576159,14.8749382835934));
#75006=CARTESIAN_POINT('Ctrl Pts',(4.94675954817621,6.44587135576157,16.8749477411846));
#75007=CARTESIAN_POINT('Ctrl Pts',(5.11829741941736,6.31422792765041,16.8664777791955));
#75008=CARTESIAN_POINT('Ctrl Pts',(5.28456668674438,6.17574134722785,16.8580078172063));
#75009=CARTESIAN_POINT('Ctrl Pts',(5.44503195406664,6.03086350216064,16.8495378552172));
#75010=CARTESIAN_POINT('Ctrl Pts',(5.60549722138891,5.88598565709341,16.841067893228));
#75011=CARTESIAN_POINT('Ctrl Pts',(5.7601582403538,5.73471678322235,16.8325979312388));
#75012=CARTESIAN_POINT('Ctrl Pts',(5.90851966259262,5.57755169937997,16.8241279692497));
#75013=CARTESIAN_POINT('Ctrl Pts',(6.05254053837894,5.42498472693902,16.8159058093031));
#75014=CARTESIAN_POINT('Ctrl Pts',(6.19067275391596,5.26681133952474,16.8076836493564));
#75015=CARTESIAN_POINT('Ctrl Pts',(6.32248991924454,5.10350945757438,16.7994614894098));
#75016=CARTESIAN_POINT('Ctrl Pts',(6.45428278679872,4.94023767695626,16.7912408450487));
#75017=CARTESIAN_POINT('Ctrl Pts',(6.57976274213852,4.77183951809809,16.7830202006876));
#75018=CARTESIAN_POINT('Ctrl Pts',(6.69854362780632,4.59882602724601,16.7747995563265));
#75019=CARTESIAN_POINT('Ctrl Pts',(6.81731116923496,4.42583197330407,16.7665798354999));
#75020=CARTESIAN_POINT('Ctrl Pts',(6.92938097651304,4.24822386574383,16.7583601146733));
#75021=CARTESIAN_POINT('Ctrl Pts',(7.03440971151707,4.06654245926615,16.7501403938467));
#75022=CARTESIAN_POINT('Ctrl Pts',(7.13944686206854,3.8848464953581,16.7419200144055));
#75023=CARTESIAN_POINT('Ctrl Pts',(7.23744166298733,3.69907683455894,16.7336996349644));
#75024=CARTESIAN_POINT('Ctrl Pts',(7.32809578457087,3.50980052633404,16.7254792555233));
#75025=CARTESIAN_POINT('Ctrl Pts',(7.4187495706669,3.3205249185719,16.7172589065036));
#75026=CARTESIAN_POINT('Ctrl Pts',(7.50206260668621,3.12774295668412,16.709038557484));
#75027=CARTESIAN_POINT('Ctrl Pts',(7.57778371056895,2.93204392844579,16.7008182084644));
#75028=CARTESIAN_POINT('Ctrl Pts',(7.65352100463689,2.73630305713668,16.6925961018241));
#75029=CARTESIAN_POINT('Ctrl Pts',(7.72166301709084,2.53764414874344,16.6843739951839));
#75030=CARTESIAN_POINT('Ctrl Pts',(7.78200728077188,2.33667504041822,16.6761518885436));
#75031=CARTESIAN_POINT('Ctrl Pts',(7.80847151749335,2.24853917245015,16.6725460482664));
#75032=CARTESIAN_POINT('Ctrl Pts',(7.83343665589362,2.15995919427053,16.6689402079893));
#75033=CARTESIAN_POINT('Ctrl Pts',(7.85688865322568,2.07098726536731,16.6653343677121));
#75034=CARTESIAN_POINT('Ctrl Pts',(7.91036469779007,1.8681104371108,16.6571122076708));
#75035=CARTESIAN_POINT('Ctrl Pts',(7.95598748355096,1.66312777465361,16.6488900476294));
#75036=CARTESIAN_POINT('Ctrl Pts',(7.9936112373037,1.45666294981097,16.6406678875881));
#75037=CARTESIAN_POINT('Ctrl Pts',(8.03122805589937,1.25023618246787,16.632447243131));
#75038=CARTESIAN_POINT('Ctrl Pts',(8.06084873241069,1.04232808823558,16.624226598674));
#75039=CARTESIAN_POINT('Ctrl Pts',(8.08237867119612,0.833572179174715,16.616005954217));
#75040=CARTESIAN_POINT('Ctrl Pts',(8.10390619123909,0.624839722422922,16.6077862332935));
#75041=CARTESIAN_POINT('Ctrl Pts',(8.11734475792283,0.415259934465333,16.5995665123701));
#75042=CARTESIAN_POINT('Ctrl Pts',(8.12265158977301,0.205471929123945,16.5913467914467));
#75043=CARTESIAN_POINT('Ctrl Pts',(8.12795884683955,-0.00433288573640242,
16.5831264119081));
#75044=CARTESIAN_POINT('Ctrl Pts',(8.12513305698705,-0.214345656326267,
16.5749060323695));
#75045=CARTESIAN_POINT('Ctrl Pts',(8.11418354199454,-0.423925712035658,
16.566685652831));
#75046=CARTESIAN_POINT('Ctrl Pts',(8.10323406752314,-0.633504992147367,
16.5584653037138));
#75047=CARTESIAN_POINT('Ctrl Pts',(8.08416094611475,-0.842651265979325,
16.5502449545965));
#75048=CARTESIAN_POINT('Ctrl Pts',(8.0570255405828,-1.05072689167856,16.5420246054793));
#75049=CARTESIAN_POINT('Ctrl Pts',(8.02988433313923,-1.2588470067217,16.5338024987418));
#75050=CARTESIAN_POINT('Ctrl Pts',(7.99467743588163,-1.46589572357169,16.5255803920043));
#75051=CARTESIAN_POINT('Ctrl Pts',(7.95151786401598,-1.67124241830284,16.5173582852668));
#75052=CARTESIAN_POINT('Ctrl Pts',(7.93259005116643,-1.76129808009773,16.5137524455694));
#75053=CARTESIAN_POINT('Ctrl Pts',(7.91213336603844,-1.85102651469605,16.510146605872));
#75054=CARTESIAN_POINT('Ctrl Pts',(7.8901604319332,-1.94037520105149,16.5065407661746));
#75055=CARTESIAN_POINT('Ctrl Pts',(7.84005699004637,-2.14411115606933,16.4983186061815));
#75056=CARTESIAN_POINT('Ctrl Pts',(7.78204990350035,-2.3459390725583,16.4900964461883));
#75057=CARTESIAN_POINT('Ctrl Pts',(7.71630954770293,-2.54524154581222,16.4818742861951));
#75058=CARTESIAN_POINT('Ctrl Pts',(7.65058130977847,-2.74450728178321,16.4736536417869));
#75059=CARTESIAN_POINT('Ctrl Pts',(7.57712274004723,-2.94124822347166,16.4654329973786));
#75060=CARTESIAN_POINT('Ctrl Pts',(7.49615386213667,-3.1348628100243,16.4572123529703));
#75061=CARTESIAN_POINT('Ctrl Pts',(7.41519408053462,-3.32845564528119,16.4489926320962));
#75062=CARTESIAN_POINT('Ctrl Pts',(7.32672578903245,-3.51892255441356,16.440772911222));
#75063=CARTESIAN_POINT('Ctrl Pts',(7.23101719068251,-3.70568184691482,16.4325531903478));
#75064=CARTESIAN_POINT('Ctrl Pts',(7.13530092356684,-3.89245610372739,16.4243328108586));
#75065=CARTESIAN_POINT('Ctrl Pts',(7.03234332261003,-4.07552188640379,16.4161124313695));
#75066=CARTESIAN_POINT('Ctrl Pts',(6.9224590889106,-4.25432106508888,16.4078920518804));
#75067=CARTESIAN_POINT('Ctrl Pts',(6.81257526186324,-4.43311958208618,16.3996717028126));
#75068=CARTESIAN_POINT('Ctrl Pts',(6.69576501015939,-4.60765127662146,16.3914513537449));
#75069=CARTESIAN_POINT('Ctrl Pts',(6.57238728445004,-4.77738557641095,16.3832310046772));
#75070=CARTESIAN_POINT('Ctrl Pts',(6.44898317893375,-4.94715616766256,16.375008897989));
#75071=CARTESIAN_POINT('Ctrl Pts',(6.31900896763612,-5.11212707613925,16.3667867913007));
#75072=CARTESIAN_POINT('Ctrl Pts',(6.18286560094914,-5.27179860418622,16.3585646846125));
#75073=CARTESIAN_POINT('Ctrl Pts',(6.12315934623455,-5.34182323451699,16.3549588446207));
#75074=CARTESIAN_POINT('Ctrl Pts',(6.06226710345063,-5.4108290610488,16.3513530046289));
#75075=CARTESIAN_POINT('Ctrl Pts',(6.00022508505059,-5.47877600301651,16.3477471646371));
#75076=CARTESIAN_POINT('Ctrl Pts',(5.85875474696184,-5.63371095033383,16.3395250046254));
#75077=CARTESIAN_POINT('Ctrl Pts',(5.71125687210847,-5.78318906605329,16.3313028446137));
#75078=CARTESIAN_POINT('Ctrl Pts',(5.55817645593022,-5.92674970344142,16.323080684602));
#75079=CARTESIAN_POINT('Ctrl Pts',(5.40512425695113,-6.07028387840413,16.3148600401749));
#75080=CARTESIAN_POINT('Ctrl Pts',(5.24649178561628,-6.20790255025607,16.3066393957479));
#75081=CARTESIAN_POINT('Ctrl Pts',(5.08276005461068,-6.33918273831525,16.2984187513208));
#75082=CARTESIAN_POINT('Ctrl Pts',(4.91904671776042,-6.470448177931,16.2901990304277));
#75083=CARTESIAN_POINT('Ctrl Pts',(4.75023549510396,-6.59537637082879,16.2819793095345));
#75084=CARTESIAN_POINT('Ctrl Pts',(4.57684020039286,-6.71358483543388,16.2737595886414));
#75085=CARTESIAN_POINT('Ctrl Pts',(4.40343101217637,-6.8318027716336,16.2655392091333));
#75086=CARTESIAN_POINT('Ctrl Pts',(4.2254372603307,-6.9432997351995,16.2573188296252));
#75087=CARTESIAN_POINT('Ctrl Pts',(4.04340231766253,-7.04773617979712,16.2490984501171));
#75088=CARTESIAN_POINT('Ctrl Pts',(3.86136804865659,-7.15217223790362,16.2408781010304));
#75089=CARTESIAN_POINT('Ctrl Pts',(3.67529287607674,-7.24954768475143,16.2326577519437));
#75090=CARTESIAN_POINT('Ctrl Pts',(3.48574584508091,-7.33956834330202,16.224437402857));
#75091=CARTESIAN_POINT('Ctrl Pts',(3.29615828639918,-7.42960824947129,16.21621529615));
#75092=CARTESIAN_POINT('Ctrl Pts',(3.10309765292968,-7.51229009904726,16.2079931894429));
#75093=CARTESIAN_POINT('Ctrl Pts',(2.9071550995866,-7.58736692070758,16.1997710827358));
#75094=CARTESIAN_POINT('Ctrl Pts',(2.82122365914698,-7.62029218027385,16.1961652428571));
#75095=CARTESIAN_POINT('Ctrl Pts',(2.73473819679738,-7.65175539049154,16.1925594029783));
#75096=CARTESIAN_POINT('Ctrl Pts',(2.64774968743878,-7.68173868047904,16.1889535630996));
#75097=CARTESIAN_POINT('Ctrl Pts',(2.44939549900504,-7.75010760869606,16.180731403092));
#75098=CARTESIAN_POINT('Ctrl Pts',(2.24835907894321,-7.81080100149879,16.1725092430844));
#75099=CARTESIAN_POINT('Ctrl Pts',(2.04525157618255,-7.86362725163285,16.1642870830768));
#75100=CARTESIAN_POINT('Ctrl Pts',(1.84218151207885,-7.91644376434298,16.1560664386539));
#75101=CARTESIAN_POINT('Ctrl Pts',(1.63704141271484,-7.96139595441826,16.147845794231));
#75102=CARTESIAN_POINT('Ctrl Pts',(1.43045603417608,-7.99834252184721,16.1396251498081));
#75103=CARTESIAN_POINT('Ctrl Pts',(1.22389386411197,-8.03528493857838,16.1314054289192));
#75104=CARTESIAN_POINT('Ctrl Pts',(1.01588702944717,-8.0642234762678,16.1231857080303));
#75105=CARTESIAN_POINT('Ctrl Pts',(0.80706971379653,-8.08506809121434,16.1149659871414));
#75106=CARTESIAN_POINT('Ctrl Pts',(0.598235666406607,-8.1059143763608,16.1067456076374));
#75107=CARTESIAN_POINT('Ctrl Pts',(0.388591301695215,-8.11866541089209,
16.0985252281335));
#75108=CARTESIAN_POINT('Ctrl Pts',(0.178776218394585,-8.12328299557737,
16.0903048486295));
#75109=CARTESIAN_POINT('Ctrl Pts',(-0.0310380884386643,-8.12790056317426,
16.0820844995469));
#75110=CARTESIAN_POINT('Ctrl Pts',(-0.241022817466202,-8.12438473731043,
16.0738641504643));
#75111=CARTESIAN_POINT('Ctrl Pts',(-0.450537532377986,-8.1127494411216,
16.0656438013817));
#75112=CARTESIAN_POINT('Ctrl Pts',(-0.660097044332808,-8.10111165715111,
16.0574216946787));
#75113=CARTESIAN_POINT('Ctrl Pts',(-0.869186046652183,-8.08135095093156,
16.0491995879757));
#75114=CARTESIAN_POINT('Ctrl Pts',(-1.07716727245303,-8.05353327612521,
16.0409774812727));
#75115=CARTESIAN_POINT('Ctrl Pts',(-1.16837832459194,-8.04133371639392,
16.0373716413692));
#75116=CARTESIAN_POINT('Ctrl Pts',(-1.25937639108115,-8.02758523259906,
16.0337658014656));
#75117=CARTESIAN_POINT('Ctrl Pts',(-1.35010815957349,-8.01229651972224,
16.0301599615621));
#75118=CARTESIAN_POINT('Ctrl Pts',(-1.55699785467115,-7.97743467146244,
16.0219378015556));
#75119=CARTESIAN_POINT('Ctrl Pts',(-1.76257068892938,-7.93454947677531,
16.0137156415492));
#75120=CARTESIAN_POINT('Ctrl Pts',(-1.96619832597162,-7.88376507168031,
16.0054934815427));
#75121=CARTESIAN_POINT('Ctrl Pts',(-2.16978842848168,-7.83299002763725,
15.997272837121));
#75122=CARTESIAN_POINT('Ctrl Pts',(-2.3714337631785,-7.77431875065692,15.9890521926992));
#75123=CARTESIAN_POINT('Ctrl Pts',(-2.57051811332891,-7.70792606292691,
15.9808315482774));
#75124=CARTESIAN_POINT('Ctrl Pts',(-2.76958009769652,-7.64154083396717,
15.9726118273896));
#75125=CARTESIAN_POINT('Ctrl Pts',(-2.96608139203507,-7.56743601939258,
15.9643921065017));
#75126=CARTESIAN_POINT('Ctrl Pts',(-3.15942202355638,-7.48583596130498,
15.9561723856139));
#75127=CARTESIAN_POINT('Ctrl Pts',(-3.35277814672597,-7.40422936491558,
15.9479520061111));
#75128=CARTESIAN_POINT('Ctrl Pts',(-3.54297282806777,-7.31512643727572,
15.9397316266083));
#75129=CARTESIAN_POINT('Ctrl Pts',(-3.72942614353552,-7.21879963722597,
15.9315112471055));
#75130=CARTESIAN_POINT('Ctrl Pts',(-3.91587876898924,-7.12247319365603,
15.9232908980242));
#75131=CARTESIAN_POINT('Ctrl Pts',(-4.0985897952732,-7.01892306899367,15.9150705489428));
#75132=CARTESIAN_POINT('Ctrl Pts',(-4.27700349969413,-6.90846789281851,
15.9068501998615));
#75133=CARTESIAN_POINT('Ctrl Pts',(-4.45545535134861,-6.79798909985103,
15.8986280931597));
#75134=CARTESIAN_POINT('Ctrl Pts',(-4.62960779451056,-6.68060246121653,
15.8904059864579));
#75135=CARTESIAN_POINT('Ctrl Pts',(-4.798932782557,-6.55667077951911,15.8821838797561));
#75136=CARTESIAN_POINT('Ctrl Pts',(-4.8731909771889,-6.50232001270836,15.8785780398456));
#75137=CARTESIAN_POINT('Ctrl Pts',(-4.94652109332637,-6.44671099355055,
15.874972199935));
#75138=CARTESIAN_POINT('Ctrl Pts',(-5.01888047592989,-6.38987686351073,
15.8713663600245));
#75139=CARTESIAN_POINT('Ctrl Pts',(-5.18387682536536,-6.2602817281944,15.863144200016));
#75140=CARTESIAN_POINT('Ctrl Pts',(-5.34387820306937,-6.1242711063155,15.8549220400074));
#75141=CARTESIAN_POINT('Ctrl Pts',(-5.49839224065822,-5.9822546193195,15.8466998799989));
#75142=CARTESIAN_POINT('Ctrl Pts',(-5.652877796788,-5.84026431011826,15.8384792355751));
#75143=CARTESIAN_POINT('Ctrl Pts',(-5.80187781438076,-5.69227054495628,
15.8302585911513));
#75144=CARTESIAN_POINT('Ctrl Pts',(-5.94493481736284,-5.53872165574396,
15.8220379467275));
#75145=CARTESIAN_POINT('Ctrl Pts',(-6.08797574885572,-5.38519001671346,
15.8138182258376));
#75146=CARTESIAN_POINT('Ctrl Pts',(-6.22507479755883,-5.22610471542581,
15.8055985049477));
#75147=CARTESIAN_POINT('Ctrl Pts',(-6.35581244339621,-5.06194979695274,
15.7973787840578));
#75148=CARTESIAN_POINT('Ctrl Pts',(-6.48656056474432,-4.89778172536987,
15.789158404553));
#75149=CARTESIAN_POINT('Ctrl Pts',(-6.61094607875186,-4.72854345413192,
15.7809380250481));
#75150=CARTESIAN_POINT('Ctrl Pts',(-6.7285900911127,-4.55475168898152,15.7727176455432));
#75151=CARTESIAN_POINT('Ctrl Pts',(-6.84623366810529,-4.3809605669868,15.7644972964597));
#75152=CARTESIAN_POINT('Ctrl Pts',(-6.95713563011982,-4.20261623069591,
15.7562769473762));
#75153=CARTESIAN_POINT('Ctrl Pts',(-7.06096042411412,-4.02026435095929,
15.7480565982927));
#75154=CARTESIAN_POINT('Ctrl Pts',(-7.16480741723577,-3.83787348195579,
15.7398344915888));
#75155=CARTESIAN_POINT('Ctrl Pts',(-7.26157407320873,-3.65147361419057,
15.7316123848849));
#75156=CARTESIAN_POINT('Ctrl Pts',(-7.35097027573048,-3.46163596697096,
15.723390278181));
#75157=CARTESIAN_POINT('Ctrl Pts',(-7.39017536092233,-3.3783818586093,15.719784438283));
#75158=CARTESIAN_POINT('Ctrl Pts',(-7.42796349162727,-3.29446686553102,
15.716178598385));
#75159=CARTESIAN_POINT('Ctrl Pts',(-7.46431306717456,-3.20994049753374,
15.712572758487));
#75160=CARTESIAN_POINT('Ctrl Pts',(-7.54686890659341,-3.01796727204274,
15.7043833055124));
#75161=CARTESIAN_POINT('Ctrl Pts',(-7.62203047401269,-2.82277096174243,
15.6961938525379));
#75162=CARTESIAN_POINT('Ctrl Pts',(-7.68956225568293,-2.62494188097117,
15.6880043995633));
#75163=CARTESIAN_POINT('Ctrl Pts',(-7.75708055109871,-2.4271523071292,15.6798165820416));
#75164=CARTESIAN_POINT('Ctrl Pts',(-7.81697200482374,-2.22673129573819,
15.67162876452));
#75165=CARTESIAN_POINT('Ctrl Pts',(-7.86905023528938,-2.02428653035882,
15.6634409469983));
#75166=CARTESIAN_POINT('Ctrl Pts',(-7.92112674591894,-1.82184845053327,
15.6552533998718));
#75167=CARTESIAN_POINT('Ctrl Pts',(-7.96539047091651,-1.61738703977369,
15.6470658527453));
#75168=CARTESIAN_POINT('Ctrl Pts',(-8.0017054032708,-1.41152336210451,15.6388783056189));
#75169=CARTESIAN_POINT('Ctrl Pts',(-8.03801842105186,-1.20567053785188,
15.6306911901511));
#75170=CARTESIAN_POINT('Ctrl Pts',(-8.06638343269783,-0.99841588989253,
15.6225040746834));
#75171=CARTESIAN_POINT('Ctrl Pts',(-8.08671577975118,-0.79038943567284,
15.6143169592157));
#75172=CARTESIAN_POINT('Ctrl Pts',(-8.10705089490952,-0.58233466012534,
15.6061287291302));
#75173=CARTESIAN_POINT('Ctrl Pts',(-8.11935113195728,-0.373508166877472,
15.5979404990448));
#75174=CARTESIAN_POINT('Ctrl Pts',(-8.12358372655715,-0.164544827070897,
15.5897522689593));
#75175=CARTESIAN_POINT('Ctrl Pts',(-8.12469591890351,-0.109635852984543,
15.5876006603853));
#75176=CARTESIAN_POINT('Ctrl Pts',(-8.12525134172209,-0.0547174411157915,
15.5854490518113));
#75177=CARTESIAN_POINT('Ctrl Pts',(-8.1252499975661,0.000198877198045901,
15.5832974432373));
#75178=CARTESIAN_POINT('Origin',(0.,0.,24.4167025567876));
#75179=CARTESIAN_POINT('',(4.94710325578446,6.44631862759455,18.8749389137103));
#75180=CARTESIAN_POINT('',(4.94687992157187,6.44602802604219,18.7083406766545));
#75181=CARTESIAN_POINT('',(4.9467595481762,6.44587135576158,24.4167025567876));
#75182=CARTESIAN_POINT('',(-8.12473160140278,0.000169117238404473,19.5832974432124));
#75183=CARTESIAN_POINT('Ctrl Pts',(-8.12473160140278,0.000169117238404473,
19.5832974432124));
#75184=CARTESIAN_POINT('Ctrl Pts',(-8.12504359874105,0.508019142218013,
19.5634046939374));
#75185=CARTESIAN_POINT('Ctrl Pts',(-7.95342738081474,2.36695158764184,19.49058074415));
#75186=CARTESIAN_POINT('Ctrl Pts',(-6.5521428145264,5.36767209002086,19.3648255938499));
#75187=CARTESIAN_POINT('Ctrl Pts',(-3.18555877319028,7.84813792090891,19.2060319923125));
#75188=CARTESIAN_POINT('Ctrl Pts',(0.957454270241905,8.41576578597796,19.0472383907749));
#75189=CARTESIAN_POINT('Ctrl Pts',(3.67473557222166,7.38452740613752,18.9368740312409));
#75190=CARTESIAN_POINT('Ctrl Pts',(4.85600651503698,6.5163309368714,18.8794408722194));
#75191=CARTESIAN_POINT('Ctrl Pts',(4.94710325578446,6.44631862759455,18.8749389137103));
#75192=CARTESIAN_POINT('',(-2.10208451021638,-7.84862588447228,20.));
#75193=CARTESIAN_POINT('Ctrl Pts',(-2.10208451021637,-7.84862588447229,
20.));
#75194=CARTESIAN_POINT('Ctrl Pts',(-3.4072189357264,-7.49907388645407,19.9470687994875));
#75195=CARTESIAN_POINT('Ctrl Pts',(-5.83842156753237,-6.13666000427729,
19.8412063984625));
#75196=CARTESIAN_POINT('Ctrl Pts',(-7.7841496768604,-3.03846725289262,19.7023055461999));
#75197=CARTESIAN_POINT('Ctrl Pts',(-8.12421342723266,-0.843282838764658,
19.6163358944499));
#75198=CARTESIAN_POINT('Ctrl Pts',(-8.12473160140278,0.000169117238404473,
19.5832974432124));
#75199=CARTESIAN_POINT('',(2.10231591215296,-7.84925099980569,20.));
#75200=CARTESIAN_POINT('Origin',(0.,0.,20.));
#75201=CARTESIAN_POINT('',(-8.12506026921708,0.000206357840382317,19.4167025567876));
#75202=CARTESIAN_POINT('Ctrl Pts',(2.10231591215296,-7.84925099980569,20.));
#75203=CARTESIAN_POINT('Ctrl Pts',(0.863038871999875,-8.18056558660505,
19.9497333973966));
#75204=CARTESIAN_POINT('Ctrl Pts',(-1.84558751149673,-8.24902228982473,
19.8465355942806));
#75205=CARTESIAN_POINT('Ctrl Pts',(-5.52703238734317,-6.41823528948013,
19.6904065906521));
#75206=CARTESIAN_POINT('Ctrl Pts',(-7.70327725426576,-3.30735306071981,
19.5462407121848));
#75207=CARTESIAN_POINT('Ctrl Pts',(-8.12411843531473,-0.977581626766432,
19.45500603423));
#75208=CARTESIAN_POINT('Ctrl Pts',(-8.12506026921708,0.000206357840382317,
19.4167025567876));
#75209=CARTESIAN_POINT('Ctrl Pts',(-8.12506026921708,0.000206357840382317,
19.4167025567876));
#75210=CARTESIAN_POINT('Ctrl Pts',(-8.12541994636447,0.373614017280771,
19.4020748337174));
#75211=CARTESIAN_POINT('Ctrl Pts',(-8.00870660044479,2.09799453871542,19.3345159101348));
#75212=CARTESIAN_POINT('Ctrl Pts',(-6.81029807173662,5.03601435634795,19.2140257860396));
#75213=CARTESIAN_POINT('Ctrl Pts',(-3.57092777478972,7.68049794291721,19.0552321845021));
#75214=CARTESIAN_POINT('Ctrl Pts',(0.538848536797422,8.45288346202083,18.8964385829646));
#75215=CARTESIAN_POINT('Ctrl Pts',(3.43586812217437,7.51499625442789,18.7808080803487));
#75216=CARTESIAN_POINT('Ctrl Pts',(4.74924899934986,6.59802379651327,18.7181087782453));
#75217=CARTESIAN_POINT('Ctrl Pts',(4.94687992157187,6.44602802604219,18.7083406766545));
#75218=CARTESIAN_POINT('Origin',(0.,0.,10.));
#75219=CARTESIAN_POINT('',(-6.57226796657889,2.44190915842114,0.660259531491259));
#75220=CARTESIAN_POINT('',(-6.57226803330854,2.44190897882182,0.113027768592106));
#75221=CARTESIAN_POINT('',(-6.57226799596304,2.44190907933527,10.));
#75222=CARTESIAN_POINT('',(-5.31037376991248,4.57794244025912,0.));
#75223=CARTESIAN_POINT('Ctrl Pts',(-6.57226803330854,2.44190897882183,0.113027768592105));
#75224=CARTESIAN_POINT('Ctrl Pts',(-6.48443345352562,2.67831107485938,0.101407930745955));
#75225=CARTESIAN_POINT('Ctrl Pts',(-6.38388671904456,2.90985881189943,0.0898378038016317));
#75226=CARTESIAN_POINT('Ctrl Pts',(-6.17965164134882,3.31832780391347,0.0690489203037348));
#75227=CARTESIAN_POINT('Ctrl Pts',(-6.08030470536102,3.49704022444068,0.0598108240986432));
#75228=CARTESIAN_POINT('Ctrl Pts',(-5.77692312506962,3.99066819037698,0.0337236943739866));
#75229=CARTESIAN_POINT('Ctrl Pts',(-5.55523859827604,4.29390135003466,0.0170257482840738));
#75230=CARTESIAN_POINT('Ctrl Pts',(-5.31037376991249,4.57794244025909,4.3758399681515E-15));
#75231=CARTESIAN_POINT('',(5.30568034743329,4.58338113332943,0.));
#75232=CARTESIAN_POINT('Origin',(0.,0.,0.));
#75233=CARTESIAN_POINT('Ctrl Pts',(5.30568034743329,4.58338113332944,6.94323071259717E-15));
#75234=CARTESIAN_POINT('Ctrl Pts',(4.96791334889641,4.97437714130201,0.0236067383578522));
#75235=CARTESIAN_POINT('Ctrl Pts',(4.58795008248023,5.3268511784941,0.0475070844258374));
#75236=CARTESIAN_POINT('Ctrl Pts',(3.85055355547309,5.87295169038987,0.0891721388758242));
#75237=CARTESIAN_POINT('Ctrl Pts',(3.50853732234251,6.08346078767968,0.107069906261077));
#75238=CARTESIAN_POINT('Ctrl Pts',(3.02818103051952,6.32506641310171,0.131176288252661));
#75239=CARTESIAN_POINT('Ctrl Pts',(2.90418137948066,6.38295193387525,0.137318833587793));
#75240=CARTESIAN_POINT('Ctrl Pts',(2.67245720329945,6.482974364138,0.148721669371288));
#75241=CARTESIAN_POINT('Ctrl Pts',(2.56523174226913,6.52614506999249,0.153974771223025));
#75242=CARTESIAN_POINT('Ctrl Pts',(2.17852954815138,6.67083431627747,0.172846788730674));
#75243=CARTESIAN_POINT('Ctrl Pts',(1.89372568641637,6.75720535105471,0.186569527123648));
#75244=CARTESIAN_POINT('Ctrl Pts',(1.41195725613856,6.87044711760687,0.209290931356877));
#75245=CARTESIAN_POINT('Ctrl Pts',(1.21778600242591,6.90750793300775,0.218323788242286));
#75246=CARTESIAN_POINT('Ctrl Pts',(0.569258507063312,7.00309095687257,0.248116670311023));
#75247=CARTESIAN_POINT('Ctrl Pts',(0.110757790567507,7.02531672066892,0.268505037624363));
#75248=CARTESIAN_POINT('Ctrl Pts',(-0.507914252363528,6.99469271472608,
0.296307214694604));
#75249=CARTESIAN_POINT('Ctrl Pts',(-0.668872106733601,6.981139755992,0.303577181476585));
#75250=CARTESIAN_POINT('Ctrl Pts',(-1.01378136682171,6.94005912625189,0.319374000659245));
#75251=CARTESIAN_POINT('Ctrl Pts',(-1.19739547110362,6.91074640970429,0.327908120856951));
#75252=CARTESIAN_POINT('Ctrl Pts',(-1.62259330619564,6.82541052256908,0.347855654488837));
#75253=CARTESIAN_POINT('Ctrl Pts',(-1.86280722624768,6.76379988414577,0.359263260409735));
#75254=CARTESIAN_POINT('Ctrl Pts',(-2.19577880582656,6.65931050020424,0.375227639560647));
#75255=CARTESIAN_POINT('Ctrl Pts',(-2.29163631047198,6.62693474892065,0.379842851859015));
#75256=CARTESIAN_POINT('Ctrl Pts',(-2.60973911421866,6.51176818465846,0.39523099159136));
#75257=CARTESIAN_POINT('Ctrl Pts',(-2.82848107349163,6.41977887178156,0.405927506613424));
#75258=CARTESIAN_POINT('Ctrl Pts',(-3.27268329389293,6.20585578736824,0.428068426288916));
#75259=CARTESIAN_POINT('Ctrl Pts',(-3.49697169700823,6.08229317503956,0.439487904763073));
#75260=CARTESIAN_POINT('Ctrl Pts',(-3.77417559254421,5.90916731010841,0.454174195423844));
#75261=CARTESIAN_POINT('Ctrl Pts',(-3.83377469301685,5.87067553207248,0.457367927034044));
#75262=CARTESIAN_POINT('Ctrl Pts',(-3.99875996351912,5.76053667290316,0.466326447082652));
#75263=CARTESIAN_POINT('Ctrl Pts',(-4.10278982410944,5.68691292843994,0.472119387767559));
#75264=CARTESIAN_POINT('Ctrl Pts',(-4.42553216947801,5.44503547688161,0.49056508378768));
#75265=CARTESIAN_POINT('Ctrl Pts',(-4.6363499694602,5.26668822082289,0.503293603600562));
#75266=CARTESIAN_POINT('Ctrl Pts',(-5.01970741925679,4.90147582916418,0.527613906159142));
#75267=CARTESIAN_POINT('Ctrl Pts',(-5.19368418101213,4.71673363498409,0.539197663955715));
#75268=CARTESIAN_POINT('Ctrl Pts',(-5.53830840738503,4.30854048464011,0.563415701596132));
#75269=CARTESIAN_POINT('Ctrl Pts',(-5.70630889343921,4.08343277863767,0.576006412544775));
#75270=CARTESIAN_POINT('Ctrl Pts',(-6.00100774244055,3.63471730934702,0.600055436935681));
#75271=CARTESIAN_POINT('Ctrl Pts',(-6.12980373036217,3.413028955647,0.611501325720239));
#75272=CARTESIAN_POINT('Ctrl Pts',(-6.30993120414253,3.05975397798143,0.629456560710598));
#75273=CARTESIAN_POINT('Ctrl Pts',(-6.36991585719028,2.93283080971328,0.635864537870555));
#75274=CARTESIAN_POINT('Ctrl Pts',(-6.47815530853341,2.68479101819484,0.648274547622285));
#75275=CARTESIAN_POINT('Ctrl Pts',(-6.52691228708205,2.5639815452794,0.654267302790969));
#75276=CARTESIAN_POINT('Ctrl Pts',(-6.57226796657889,2.44190915842114,0.660259531491259));
#75277=CARTESIAN_POINT('Origin',(0.,0.,10.));
#75278=CARTESIAN_POINT('',(-6.57226793021668,2.44190925628809,2.66021763119828));
#75279=CARTESIAN_POINT('',(-6.57226800353884,2.44190905894539,2.1130822547889));
#75280=CARTESIAN_POINT('',(-6.57226799596304,2.44190907933527,10.));
#75281=CARTESIAN_POINT('Ctrl Pts',(-6.57226800353884,2.44190905894539,2.1130822547889));
#75282=CARTESIAN_POINT('Ctrl Pts',(-6.49279312640791,2.65581145229596,2.10284308653732));
#75283=CARTESIAN_POINT('Ctrl Pts',(-6.40291465001429,2.86572907629688,2.09265138196384));
#75284=CARTESIAN_POINT('Ctrl Pts',(-6.25383406080689,3.17171237278575,2.07736071604314));
#75285=CARTESIAN_POINT('Ctrl Pts',(-6.20231043424039,3.27132154565605,2.07231009358979));
#75286=CARTESIAN_POINT('Ctrl Pts',(-6.08508969571202,3.48520790432581,2.06125649921506));
#75287=CARTESIAN_POINT('Ctrl Pts',(-6.01851470692794,3.5989540390872,2.0552377909509));
#75288=CARTESIAN_POINT('Ctrl Pts',(-5.80822232179475,3.93607744699537,2.03701748118551));
#75289=CARTESIAN_POINT('Ctrl Pts',(-5.65498086469982,4.15323297416772,2.02476943204738));
#75290=CARTESIAN_POINT('Ctrl Pts',(-5.36701183334432,4.51572497144245,2.00352705492179));
#75291=CARTESIAN_POINT('Ctrl Pts',(-5.23775930831982,4.66502596046627,1.99451177070619));
#75292=CARTESIAN_POINT('Ctrl Pts',(-4.82370543706551,5.10436928212147,1.9671001200107));
#75293=CARTESIAN_POINT('Ctrl Pts',(-4.51985522445697,5.37527987021319,1.94896666566469));
#75294=CARTESIAN_POINT('Ctrl Pts',(-4.04376068101001,5.73069775673144,1.92233086230248));
#75295=CARTESIAN_POINT('Ctrl Pts',(-3.88881481972275,5.83695252404356,1.91389524311176));
#75296=CARTESIAN_POINT('Ctrl Pts',(-3.5141836513171,6.07231218219803,1.89379320727144));
#75297=CARTESIAN_POINT('Ctrl Pts',(-3.29135777375622,6.19591988878065,1.88207047139596));
#75298=CARTESIAN_POINT('Ctrl Pts',(-2.79373886227124,6.43752915577014,1.85661779779701));
#75299=CARTESIAN_POINT('Ctrl Pts',(-2.51711303562919,6.55064161661477,1.84292144775973));
#75300=CARTESIAN_POINT('Ctrl Pts',(-2.00143274165636,6.7239983977605,1.81819065650761));
#75301=CARTESIAN_POINT('Ctrl Pts',(-1.76479801681821,6.78994686428469,1.8071292352449));
#75302=CARTESIAN_POINT('Ctrl Pts',(-1.30041644677844,6.8934444387163,1.78577738801826));
#75303=CARTESIAN_POINT('Ctrl Pts',(-1.07331225438102,6.93243532046221,1.77549348767729));
#75304=CARTESIAN_POINT('Ctrl Pts',(-0.694225197395039,6.97844215541894,
1.75834063160464));
#75305=CARTESIAN_POINT('Ctrl Pts',(-0.54319809609625,6.99181941615377,1.75150790838926));
#75306=CARTESIAN_POINT('Ctrl Pts',(-0.144797896936059,7.01412067457361,
1.73334900114839));
#75307=CARTESIAN_POINT('Ctrl Pts',(0.102816355217044,7.01486149949597,1.72195436564623));
#75308=CARTESIAN_POINT('Ctrl Pts',(0.643198637537469,6.98785610048713,1.69706021019252));
#75309=CARTESIAN_POINT('Ctrl Pts',(0.935243580742794,6.95479415869257,1.68359416102377));
#75310=CARTESIAN_POINT('Ctrl Pts',(1.68928804648194,6.82106240345378,1.64878674172699));
#75311=CARTESIAN_POINT('Ctrl Pts',(2.14469936525171,6.69184982170806,1.62778302068919));
#75312=CARTESIAN_POINT('Ctrl Pts',(2.7255129671203,6.46161666541025,1.59972124012996));
#75313=CARTESIAN_POINT('Ctrl Pts',(2.86549027479619,6.40077149314128,1.59284387525232));
#75314=CARTESIAN_POINT('Ctrl Pts',(3.2293496599641,6.22827984587918,1.57452009409872));
#75315=CARTESIAN_POINT('Ctrl Pts',(3.44943235845743,6.10913931908499,1.56300295340686));
#75316=CARTESIAN_POINT('Ctrl Pts',(3.92787635503417,5.81602462338885,1.53718748372424));
#75317=CARTESIAN_POINT('Ctrl Pts',(4.18197629092144,5.63608334722262,1.52293114114716));
#75318=CARTESIAN_POINT('Ctrl Pts',(4.73019815009442,5.19031032768737,1.49085352556271));
#75319=CARTESIAN_POINT('Ctrl Pts',(5.01543714730117,4.91523052639097,1.47319127530002));
#75320=CARTESIAN_POINT('Ctrl Pts',(5.4040528509735,4.47120451168982,1.44674285207172));
#75321=CARTESIAN_POINT('Ctrl Pts',(5.52600220610544,4.31957805856301,1.43801089281206));
#75322=CARTESIAN_POINT('Ctrl Pts',(5.79602963515161,3.95365756666718,1.41735159340973));
#75323=CARTESIAN_POINT('Ctrl Pts',(5.93878852624269,3.73579385192775,1.40536673500222));
#75324=CARTESIAN_POINT('Ctrl Pts',(6.217113782653,3.25461347645448,1.37979016067684));
#75325=CARTESIAN_POINT('Ctrl Pts',(6.34879583875365,2.98961688460007,1.36623096200207));
#75326=CARTESIAN_POINT('Ctrl Pts',(6.55710077293798,2.49410679385626,1.34179868138937));
#75327=CARTESIAN_POINT('Ctrl Pts',(6.6392410051092,2.2664114793094,1.33089806488089));
#75328=CARTESIAN_POINT('Ctrl Pts',(6.79873075296536,1.74054994326668,1.30623503290395));
#75329=CARTESIAN_POINT('Ctrl Pts',(6.86854119434363,1.44062215947135,1.29253162590189));
#75330=CARTESIAN_POINT('Ctrl Pts',(6.93901190680758,1.01185320266401,1.27291463982902));
#75331=CARTESIAN_POINT('Ctrl Pts',(6.95618993896126,0.88608901596617,1.26714804521847));
#75332=CARTESIAN_POINT('Ctrl Pts',(6.99997323701482,0.48451553450993,1.24867921127313));
#75333=CARTESIAN_POINT('Ctrl Pts',(7.01365072944863,0.207565591087008,1.23589750904888));
#75334=CARTESIAN_POINT('Ctrl Pts',(7.00837627413621,-0.324770476602897,
1.21144199179764));
#75335=CARTESIAN_POINT('Ctrl Pts',(6.99190294887023,-0.579750598249626,
1.19977695961132));
#75336=CARTESIAN_POINT('Ctrl Pts',(6.92380854636316,-1.14864810171334,1.17380034313954));
#75337=CARTESIAN_POINT('Ctrl Pts',(6.86467056097649,-1.46110209823195,1.15957432486484));
#75338=CARTESIAN_POINT('Ctrl Pts',(6.72514814806198,-1.99636505123688,1.13479810361725));
#75339=CARTESIAN_POINT('Ctrl Pts',(6.6543009970792,-2.221118206933,1.12425877640029));
#75340=CARTESIAN_POINT('Ctrl Pts',(6.51576150794132,-2.59399563783087,1.10621865276002));
#75341=CARTESIAN_POINT('Ctrl Pts',(6.45397931128989,-2.74410468677476,1.09878904586431));
#75342=CARTESIAN_POINT('Ctrl Pts',(6.19887618598403,-3.30751887337305,1.0703796101476));
#75343=CARTESIAN_POINT('Ctrl Pts',(5.97058761211762,-3.703761406826,1.04937976319834));
#75344=CARTESIAN_POINT('Ctrl Pts',(5.53560492813307,-4.31278069371356,1.01546062965234));
#75345=CARTESIAN_POINT('Ctrl Pts',(5.35108519743545,-4.5397015208267,1.00236202317304));
#75346=CARTESIAN_POINT('Ctrl Pts',(4.98326101475976,-4.93835500990896,0.978065917075798));
#75347=CARTESIAN_POINT('Ctrl Pts',(4.80385596417464,-5.11304262589715,0.966879410479455));
#75348=CARTESIAN_POINT('Ctrl Pts',(4.5014235621914,-5.37752532508763,0.948668903431823));
#75349=CARTESIAN_POINT('Ctrl Pts',(4.38414420895216,-5.47356103972028,0.941738102653115));
#75350=CARTESIAN_POINT('Ctrl Pts',(4.08111497310209,-5.70570903579223,0.924213992744855));
#75351=CARTESIAN_POINT('Ctrl Pts',(3.89159880535497,-5.83661494977194,0.913603035218845));
#75352=CARTESIAN_POINT('Ctrl Pts',(3.48745112933642,-6.08732565936716,0.891767238045576));
#75353=CARTESIAN_POINT('Ctrl Pts',(3.27226412748057,-6.20565386843528,0.880564244524344));
#75354=CARTESIAN_POINT('Ctrl Pts',(2.7845335893355,-6.44141293850014,0.85601515254437));
#75355=CARTESIAN_POINT('Ctrl Pts',(2.50984486143492,-6.55332817754673,0.842735694799498));
#75356=CARTESIAN_POINT('Ctrl Pts',(1.983661245951,-6.72975609073621,0.817877494194208));
#75357=CARTESIAN_POINT('Ctrl Pts',(1.73406594405275,-6.79834832786492,0.806312481595107));
#75358=CARTESIAN_POINT('Ctrl Pts',(1.28669542541168,-6.89504636326368,0.785531617432516));
#75359=CARTESIAN_POINT('Ctrl Pts',(1.0904332236139,-6.92879518929464,0.776394530482349));
#75360=CARTESIAN_POINT('Ctrl Pts',(0.52956158706368,-7.00081852693867,0.750388408331139));
#75361=CARTESIAN_POINT('Ctrl Pts',(0.163011828899802,-7.01892666715469,
0.733544461211931));
#75362=CARTESIAN_POINT('Ctrl Pts',(-0.459091340103273,-7.00088276558127,
0.70526777664876));
#75363=CARTESIAN_POINT('Ctrl Pts',(-0.714313479005114,-6.97946157114112,
0.693746958941813));
#75364=CARTESIAN_POINT('Ctrl Pts',(-1.24394001082276,-6.90564819119305,
0.669762296487304));
#75365=CARTESIAN_POINT('Ctrl Pts',(-1.51754068417451,-6.8507248734772,0.657328439064246));
#75366=CARTESIAN_POINT('Ctrl Pts',(-1.90905962857967,-6.74751918273071,
0.639061742462014));
#75367=CARTESIAN_POINT('Ctrl Pts',(-2.03008692504151,-6.71209878603812,
0.633339548630402));
#75368=CARTESIAN_POINT('Ctrl Pts',(-2.44175009212672,-6.57946629418827,
0.61357881644767));
#75369=CARTESIAN_POINT('Ctrl Pts',(-2.72693222177506,-6.46647975880543,
0.599429740775669));
#75370=CARTESIAN_POINT('Ctrl Pts',(-3.22454520072293,-6.23053887926962,
0.574142576554722));
#75371=CARTESIAN_POINT('Ctrl Pts',(-3.43966601976377,-6.11440982550656,
0.562989124960971));
#75372=CARTESIAN_POINT('Ctrl Pts',(-3.81618798289243,-5.88498028555875,
0.543006541645807));
#75373=CARTESIAN_POINT('Ctrl Pts',(-3.97971107958816,-5.7756544989867,0.534155795878401));
#75374=CARTESIAN_POINT('Ctrl Pts',(-4.3558787901782,-5.5005923601428,0.513244021840513));
#75375=CARTESIAN_POINT('Ctrl Pts',(-4.56398686139376,-5.32918554740747,
0.501228754710601));
#75376=CARTESIAN_POINT('Ctrl Pts',(-4.85889269374257,-5.05631458197018,
0.483138362108514));
#75377=CARTESIAN_POINT('Ctrl Pts',(-4.95350243808937,-4.96366482040794,
0.477147569826183));
#75378=CARTESIAN_POINT('Ctrl Pts',(-5.13437554873011,-4.77621415676932,
0.465268085802562));
#75379=CARTESIAN_POINT('Ctrl Pts',(-5.22077473879689,-4.68161772997975,
0.459393220794168));
#75380=CARTESIAN_POINT('Ctrl Pts',(-5.58263483472045,-4.26294358824424,
0.43396165710622));
#75381=CARTESIAN_POINT('Ctrl Pts',(-5.83089024532003,-3.91653328043703,
0.414399752780401));
#75382=CARTESIAN_POINT('Ctrl Pts',(-6.09739427006168,-3.46260381604466,
0.390526191683218));
#75383=CARTESIAN_POINT('Ctrl Pts',(-6.1466760514654,-3.37434672637,0.385956771612364));
#75384=CARTESIAN_POINT('Ctrl Pts',(-6.30204945332605,-3.08138722638288,
0.371003577210365));
#75385=CARTESIAN_POINT('Ctrl Pts',(-6.39995552547464,-2.8725154476415,0.360682872803395));
#75386=CARTESIAN_POINT('Ctrl Pts',(-6.57444378949163,-2.44683317023401,
0.340073643603738));
#75387=CARTESIAN_POINT('Ctrl Pts',(-6.65101183465584,-2.23032335448553,
0.329797065975353));
#75388=CARTESIAN_POINT('Ctrl Pts',(-6.76540054318372,-1.8481563762227,0.311701115082449));
#75389=CARTESIAN_POINT('Ctrl Pts',(-6.8080794005409,-1.68415538730638,0.303940974934625));
#75390=CARTESIAN_POINT('Ctrl Pts',(-6.93962976274809,-1.09128687920283,
0.276039159265955));
#75391=CARTESIAN_POINT('Ctrl Pts',(-6.99423014699099,-0.655842069030141,
0.25589408105819));
#75392=CARTESIAN_POINT('Ctrl Pts',(-7.0109706278193,-0.118077221317558,
0.231504526978879));
#75393=CARTESIAN_POINT('Ctrl Pts',(-7.01194192434386,-0.0179459306536899,
0.226980140501383));
#75394=CARTESIAN_POINT('Ctrl Pts',(-7.00804521914173,0.314512647529299,
0.211994204451907));
#75395=CARTESIAN_POINT('Ctrl Pts',(-6.99377388525388,0.546574713582783,
0.201596821116923));
#75396=CARTESIAN_POINT('Ctrl Pts',(-6.94438043931484,0.989241965167925,
0.181643537258381));
#75397=CARTESIAN_POINT('Ctrl Pts',(-6.91111505020142,1.19979400991379,0.172098775150825));
#75398=CARTESIAN_POINT('Ctrl Pts',(-6.84595513888636,1.51753526881411,0.157393470294117));
#75399=CARTESIAN_POINT('Ctrl Pts',(-6.82100244102319,1.62601963603786,0.152312659542052));
#75400=CARTESIAN_POINT('Ctrl Pts',(-6.75160255402251,1.89793664833274,0.139444578944936));
#75401=CARTESIAN_POINT('Ctrl Pts',(-6.70379667449445,2.0604392966348,0.131635618956626));
#75402=CARTESIAN_POINT('Ctrl Pts',(-6.62541859343733,2.29511491041281,0.120224315696719));
#75403=CARTESIAN_POINT('Ctrl Pts',(-6.59945212357222,2.36874444689044,0.116624014189679));
#75404=CARTESIAN_POINT('Ctrl Pts',(-6.57226803330854,2.44190897882182,0.113027768592106));
#75405=CARTESIAN_POINT('Ctrl Pts',(-6.57226796657889,2.44190915842114,0.660259531491259));
#75406=CARTESIAN_POINT('Ctrl Pts',(-6.61936822038628,2.315141343063,0.666482247053822));
#75407=CARTESIAN_POINT('Ctrl Pts',(-6.66280048077769,2.18701158570925,0.672704323074592));
#75408=CARTESIAN_POINT('Ctrl Pts',(-6.76042717422472,1.86901087077713,0.687967745466177));
#75409=CARTESIAN_POINT('Ctrl Pts',(-6.81035720103147,1.67797906830669,0.696981790108703));
#75410=CARTESIAN_POINT('Ctrl Pts',(-6.93827667256961,1.08776383334722,0.724403037241743));
#75411=CARTESIAN_POINT('Ctrl Pts',(-6.98966943009966,0.683695560157103,
0.742546829547995));
#75412=CARTESIAN_POINT('Ctrl Pts',(-7.01318344917094,0.0899608285585705,
0.769185932077584));
#75413=CARTESIAN_POINT('Ctrl Pts',(-7.01307905937192,-0.097751731837338,
0.777614190741723));
#75414=CARTESIAN_POINT('Ctrl Pts',(-6.99508835007367,-0.539614474412561,
0.79770720508367));
#75415=CARTESIAN_POINT('Ctrl Pts',(-6.97088291521988,-0.793242383565875,
0.809428378410608));
#75416=CARTESIAN_POINT('Ctrl Pts',(-6.88843545187471,-1.34023746984631,
0.834881134791783));
#75417=CARTESIAN_POINT('Ctrl Pts',(-6.82511734801832,-1.63234732784954,
0.848579118604667));
#75418=CARTESIAN_POINT('Ctrl Pts',(-6.67614967385812,-2.15567478138416,
0.873313457990113));
#75419=CARTESIAN_POINT('Ctrl Pts',(-6.59657233599127,-2.38812575784159,
0.884376783898336));
#75420=CARTESIAN_POINT('Ctrl Pts',(-6.41922320370544,-2.8291359735642,0.905708877608907));
#75421=CARTESIAN_POINT('Ctrl Pts',(-6.32305169926817,-3.03800158252752,
0.91597138101971));
#75422=CARTESIAN_POINT('Ctrl Pts',(-6.14659171595843,-3.37640232553529,
0.933113913625399));
#75423=CARTESIAN_POINT('Ctrl Pts',(-6.07203166188136,-3.50871960366765,
0.939958145794952));
#75424=CARTESIAN_POINT('Ctrl Pts',(-5.86455968270675,-3.8504604144153,0.958151611574397));
#75425=CARTESIAN_POINT('Ctrl Pts',(-5.72473384552216,-4.05543164861286,
0.969569682469305));
#75426=CARTESIAN_POINT('Ctrl Pts',(-5.38708352780995,-4.49803064641249,
0.995182915034166));
#75427=CARTESIAN_POINT('Ctrl Pts',(-5.18380813011305,-4.73086544284331,
1.00933743455038));
#75428=CARTESIAN_POINT('Ctrl Pts',(-4.67558223594547,-5.24076520041791,
1.04202846822909));
#75429=CARTESIAN_POINT('Ctrl Pts',(-4.36026230076107,-5.50588837385504,
1.06037448841543));
#75430=CARTESIAN_POINT('Ctrl Pts',(-3.87207580808598,-5.84797885991537,
1.08710191118593));
#75431=CARTESIAN_POINT('Ctrl Pts',(-3.71648496687771,-5.9480724317828,1.09541051428432));
#75432=CARTESIAN_POINT('Ctrl Pts',(-3.33988855493214,-6.16979077412279,
1.11526821476839));
#75433=CARTESIAN_POINT('Ctrl Pts',(-3.11591821679655,-6.28587501970539,
1.12687294108092));
#75434=CARTESIAN_POINT('Ctrl Pts',(-2.61291044936449,-6.51308241471437,
1.15226926876994));
#75435=CARTESIAN_POINT('Ctrl Pts',(-2.33199250240424,-6.61886393100552,
1.16602690499378));
#75436=CARTESIAN_POINT('Ctrl Pts',(-1.81089882002314,-6.77777660847228,
1.19079253406406));
#75437=CARTESIAN_POINT('Ctrl Pts',(-1.573049494107,-6.83689465731812,1.20182917749871));
#75438=CARTESIAN_POINT('Ctrl Pts',(-1.03084935256075,-6.94186122754047,
1.22661480723018));
#75439=CARTESIAN_POINT('Ctrl Pts',(-0.725595226018135,-6.98037216848192,
1.24030642864799));
#75440=CARTESIAN_POINT('Ctrl Pts',(-0.292014700059731,-7.00631766596057,
1.25991751660996));
#75441=CARTESIAN_POINT('Ctrl Pts',(-0.165045143543451,-7.01045782870972,
1.26568962695711));
#75442=CARTESIAN_POINT('Ctrl Pts',(0.238693467207839,-7.01264802599733,
1.28415035480813));
#75443=CARTESIAN_POINT('Ctrl Pts',(0.515266268549994,-6.99776443004944,
1.29691748561911));
#75444=CARTESIAN_POINT('Ctrl Pts',(1.04346536383209,-6.93784967375325,1.32133664779025));
#75445=CARTESIAN_POINT('Ctrl Pts',(1.29494606342271,-6.89533875000542,1.33298009214175));
#75446=CARTESIAN_POINT('Ctrl Pts',(1.84866222491564,-6.77036970411805,1.35871509899302));
#75447=CARTESIAN_POINT('Ctrl Pts',(2.1488205305843,-6.68116997282315,1.37272688720449));
#75448=CARTESIAN_POINT('Ctrl Pts',(2.67319084871069,-6.48633136884539,1.39778278828183));
#75449=CARTESIAN_POINT('Ctrl Pts',(2.89966422100529,-6.38830083873669,1.40881530300481));
#75450=CARTESIAN_POINT('Ctrl Pts',(3.28135669597843,-6.19859599839696,1.42816014400196));
#75451=CARTESIAN_POINT('Ctrl Pts',(3.43908184739036,-6.11249606713499,1.43639624344593));
#75452=CARTESIAN_POINT('Ctrl Pts',(3.95447280276339,-5.80488272126014,1.46398870568754));
#75453=CARTESIAN_POINT('Ctrl Pts',(4.29550328604515,-5.55726408383358,1.48333310074313));
#75454=CARTESIAN_POINT('Ctrl Pts',(4.68765706420252,-5.21474000877471,1.50694859177633));
#75455=CARTESIAN_POINT('Ctrl Pts',(4.76161352378925,-5.14729822295721,1.51147318897595));
#75456=CARTESIAN_POINT('Ctrl Pts',(5.00185371129468,-4.91861021400595,1.52642990714244));
#75457=CARTESIAN_POINT('Ctrl Pts',(5.16159132140603,-4.7507097600355,1.5367973026684));
#75458=CARTESIAN_POINT('Ctrl Pts',(5.46258012305145,-4.40120212931766,1.55745765299244));
#75459=CARTESIAN_POINT('Ctrl Pts',(5.6037917062938,-4.21993806318362,1.56773860539465));
#75460=CARTESIAN_POINT('Ctrl Pts',(5.83129670770962,-3.89629954326537,1.5856834502393));
#75461=CARTESIAN_POINT('Ctrl Pts',(5.92188903016706,-3.75717976725567,1.5932846164083));
#75462=CARTESIAN_POINT('Ctrl Pts',(6.23839646056179,-3.23120029089253,1.62148845238909));
#75463=CARTESIAN_POINT('Ctrl Pts',(6.4320345802714,-2.82616238410946,1.64210299742816));
#75464=CARTESIAN_POINT('Ctrl Pts',(6.62010692382887,-2.31124717132462,1.66695278150905));
#75465=CARTESIAN_POINT('Ctrl Pts',(6.65248120535126,-2.21634230563035,1.671483331566));
#75466=CARTESIAN_POINT('Ctrl Pts',(6.75347201079601,-1.89810855152635,1.6865316777584));
#75467=CARTESIAN_POINT('Ctrl Pts',(6.81296227369022,-1.67204857049558,1.69698455267594));
#75468=CARTESIAN_POINT('Ctrl Pts',(6.9051213163183,-1.23399207133201,1.71703715294312));
#75469=CARTESIAN_POINT('Ctrl Pts',(6.93957093184892,-1.02263856339566,1.72662554848845));
#75470=CARTESIAN_POINT('Ctrl Pts',(6.98238237215309,-0.654570222906499,
1.74342556754275));
#75471=CARTESIAN_POINT('Ctrl Pts',(6.99525443619507,-0.498537135387838,
1.75058753721644));
#75472=CARTESIAN_POINT('Ctrl Pts',(7.010322312855,-0.190189817221909,1.76476366493551));
#75473=CARTESIAN_POINT('Ctrl Pts',(7.0127989560457,-0.0379708568626089,
1.77177198096467));
#75474=CARTESIAN_POINT('Ctrl Pts',(7.00590491700599,0.385200883853832,1.79123813732939));
#75475=CARTESIAN_POINT('Ctrl Pts',(6.9857803295653,0.655713888114175,1.80365465089155));
#75476=CARTESIAN_POINT('Ctrl Pts',(6.91653182200668,1.17636325315985,1.8275194242353));
#75477=CARTESIAN_POINT('Ctrl Pts',(6.86933868967801,1.42633519478744,1.83896357813441));
#75478=CARTESIAN_POINT('Ctrl Pts',(6.74271737357749,1.94159115104607,1.8627630149837));
#75479=CARTESIAN_POINT('Ctrl Pts',(6.66094840059031,2.20585078870684,1.87508905047707));
#75480=CARTESIAN_POINT('Ctrl Pts',(6.5190987862986,2.5836303826207,1.89328823747418));
#75481=CARTESIAN_POINT('Ctrl Pts',(6.47117247103299,2.70142944935583,1.89905634554082));
#75482=CARTESIAN_POINT('Ctrl Pts',(6.29613598649128,3.10022366737014,1.91894843544529));
#75483=CARTESIAN_POINT('Ctrl Pts',(6.15370994481535,3.37410263845989,1.93318482723096));
#75484=CARTESIAN_POINT('Ctrl Pts',(5.86655379879665,3.84723856177491,1.95859309166131));
#75485=CARTESIAN_POINT('Ctrl Pts',(5.72848814684077,4.04995369789045,1.96978083621134));
#75486=CARTESIAN_POINT('Ctrl Pts',(5.39881645172317,4.48330749652224,1.99445368730968));
#75487=CARTESIAN_POINT('Ctrl Pts',(5.20246590427389,4.7097364255845,2.00786845093655));
#75488=CARTESIAN_POINT('Ctrl Pts',(4.81460842040578,5.10305536796147,2.03261045289571));
#75489=CARTESIAN_POINT('Ctrl Pts',(4.62735880958025,5.27344050435344,2.04392482673201));
#75490=CARTESIAN_POINT('Ctrl Pts',(4.28719831610805,5.55086859526103,2.06385042962107));
#75491=CARTESIAN_POINT('Ctrl Pts',(4.13846411214626,5.66262521653732,2.07238095550425));
#75492=CARTESIAN_POINT('Ctrl Pts',(3.64863908404127,6.00105580070087,2.09975642510544));
#75493=CARTESIAN_POINT('Ctrl Pts',(3.29206724194482,6.20383301847566,2.11858113930592));
#75494=CARTESIAN_POINT('Ctrl Pts',(2.82886856279303,6.4160066621223,2.14169311823062));
#75495=CARTESIAN_POINT('Ctrl Pts',(2.73701484019737,6.45572527565513,2.14621783153879));
#75496=CARTESIAN_POINT('Ctrl Pts',(2.53837369202448,6.53661816842051,2.15589114260135));
#75497=CARTESIAN_POINT('Ctrl Pts',(2.43136442889559,6.57717153160591,2.16103457980988));
#75498=CARTESIAN_POINT('Ctrl Pts',(2.06677022413769,6.70522755816935,2.17837491338701));
#75499=CARTESIAN_POINT('Ctrl Pts',(1.80510395581976,6.78035497916357,2.19050677621098));
#75500=CARTESIAN_POINT('Ctrl Pts',(1.41217581221567,6.86880504155568,2.20864697954383));
#75501=CARTESIAN_POINT('Ctrl Pts',(1.28383841713066,6.89394528751383,2.21456589966175));
#75502=CARTESIAN_POINT('Ctrl Pts',(1.02805676988242,6.93666032647216,2.22639567796045));
#75503=CARTESIAN_POINT('Ctrl Pts',(0.900683769950669,6.9543457959294,2.23229418558519));
#75504=CARTESIAN_POINT('Ctrl Pts',(0.350565115262764,7.01536098208177,2.25773672936224));
#75505=CARTESIAN_POINT('Ctrl Pts',(-0.0751629981528878,7.02371344715437,
2.27728272193942));
#75506=CARTESIAN_POINT('Ctrl Pts',(-0.80261055115844,6.97180582807092,2.31035747959763));
#75507=CARTESIAN_POINT('Ctrl Pts',(-1.10446594334541,6.93039819291771,2.32400196811033));
#75508=CARTESIAN_POINT('Ctrl Pts',(-1.64609895777159,6.81980274987345,2.34876344590875));
#75509=CARTESIAN_POINT('Ctrl Pts',(-1.88670363915619,6.75719596037491,2.35987122714874));
#75510=CARTESIAN_POINT('Ctrl Pts',(-2.26830368167821,6.63592640849457,2.37801947398393));
#75511=CARTESIAN_POINT('Ctrl Pts',(-2.41159680567609,6.58520462257227,2.3849694346356));
#75512=CARTESIAN_POINT('Ctrl Pts',(-2.76675639064031,6.44634010168383,2.40247500024569));
#75513=CARTESIAN_POINT('Ctrl Pts',(-2.9761596105,6.35237876013932,2.41304764497562));
#75514=CARTESIAN_POINT('Ctrl Pts',(-3.39946457423003,6.13690408246136,2.43485441723145));
#75515=CARTESIAN_POINT('Ctrl Pts',(-3.61234605431573,6.01405940181746,2.44606627064762));
#75516=CARTESIAN_POINT('Ctrl Pts',(-4.06844913358781,5.71789087354352,2.47070937757767));
#75517=CARTESIAN_POINT('Ctrl Pts',(-4.30793992709884,5.53969416749828,2.48407201280389));
#75518=CARTESIAN_POINT('Ctrl Pts',(-4.73004461640136,5.18164827813524,2.50886414163479));
#75519=CARTESIAN_POINT('Ctrl Pts',(-4.91556327632237,5.00599984984363,2.52028047616279));
#75520=CARTESIAN_POINT('Ctrl Pts',(-5.22069421682454,4.68374987365058,2.54042726024354));
#75521=CARTESIAN_POINT('Ctrl Pts',(-5.34472780304034,4.5417005268804,2.54907554572099));
#75522=CARTESIAN_POINT('Ctrl Pts',(-5.71684159521833,4.0791535412962,2.57637391166004));
#75523=CARTESIAN_POINT('Ctrl Pts',(-5.94296471403411,3.74205216656131,2.59500086617898));
#75524=CARTESIAN_POINT('Ctrl Pts',(-6.23407490378244,3.21448295770506,2.62233697489158));
#75525=CARTESIAN_POINT('Ctrl Pts',(-6.32210011202131,3.03770346464745,2.63123157730135));
#75526=CARTESIAN_POINT('Ctrl Pts',(-6.46356288804325,2.72073401664894,2.64681712099078));
#75527=CARTESIAN_POINT('Ctrl Pts',(-6.52016167747087,2.5821504437946,2.65351582122961));
#75528=CARTESIAN_POINT('Ctrl Pts',(-6.57226793021667,2.4419092562881,2.66021763119828));
#75529=CARTESIAN_POINT('Origin',(0.,0.,10.));
#75530=CARTESIAN_POINT('',(-6.57226799596304,2.44190907933527,4.66030144016832));
#75531=CARTESIAN_POINT('',(-6.57269630323124,2.4420685397187,4.11322495262288));
#75532=CARTESIAN_POINT('',(-6.57226799596304,2.44190907933527,10.));
#75533=CARTESIAN_POINT('',(-7.01180849524368,2.69103457778642E-5,2.22648654173946));
#75534=CARTESIAN_POINT('Ctrl Pts',(-6.57269630323124,2.4420685397187,4.11322495262288));
#75535=CARTESIAN_POINT('Ctrl Pts',(-6.20535467906786,3.42842235222112,4.0654299812279));
#75536=CARTESIAN_POINT('Ctrl Pts',(-4.95782740744273,5.33202724196766,3.96470380932042));
#75537=CARTESIAN_POINT('Ctrl Pts',(-1.91930106773404,7.05226072421662,3.81104643690041));
#75538=CARTESIAN_POINT('Ctrl Pts',(1.68861748831434,7.11102446149387,3.65225283536289));
#75539=CARTESIAN_POINT('Ctrl Pts',(4.88493970070459,5.43649354182164,3.49345923382538));
#75540=CARTESIAN_POINT('Ctrl Pts',(6.89056992096269,2.43683074440551,3.33466563228786));
#75541=CARTESIAN_POINT('Ctrl Pts',(7.21664073544971,-1.15680353300375,3.17587203075035));
#75542=CARTESIAN_POINT('Ctrl Pts',(5.78367318632997,-4.46846980083332,3.01707842921281));
#75543=CARTESIAN_POINT('Ctrl Pts',(2.94094957949722,-6.69095759537126,2.85828482767533));
#75544=CARTESIAN_POINT('Ctrl Pts',(-0.618623231225066,-7.28254097808985,
2.69949122613779));
#75545=CARTESIAN_POINT('Ctrl Pts',(-4.02740814743654,-6.09902301034318,
2.54069762460028));
#75546=CARTESIAN_POINT('Ctrl Pts',(-6.4374277342472,-3.44768939946999,2.38302243189696));
#75547=CARTESIAN_POINT('Ctrl Pts',(-7.01160457735808,-1.14092551293614,
2.27827843970617));
#75548=CARTESIAN_POINT('Ctrl Pts',(-7.0118447620046,2.59581319030052E-5,
2.22646564802786));
#75549=CARTESIAN_POINT('Ctrl Pts',(-7.01124999987674,4.1574104656346E-5,
2.22680829755206));
#75550=CARTESIAN_POINT('Ctrl Pts',(-7.01124960066053,0.0673672487642149,
2.22375897461869));
#75551=CARTESIAN_POINT('Ctrl Pts',(-7.01027946364388,0.13468844982995,2.2206980026699));
#75552=CARTESIAN_POINT('Ctrl Pts',(-6.99921204821522,0.518698384756561,
2.20317221559078));
#75553=CARTESIAN_POINT('Ctrl Pts',(-6.96862589450747,0.834427695950238,
2.18854167333345));
#75554=CARTESIAN_POINT('Ctrl Pts',(-6.88439660075787,1.34235720129083,2.16490095114753));
#75555=CARTESIAN_POINT('Ctrl Pts',(-6.84373919639515,1.53625353620252,2.15584663781379));
#75556=CARTESIAN_POINT('Ctrl Pts',(-6.74359093682043,1.93002273684355,2.1373776599019));
#75557=CARTESIAN_POINT('Ctrl Pts',(-6.6832839369519,2.12948920324959,2.12797811415362));
#75558=CARTESIAN_POINT('Ctrl Pts',(-6.60055197415375,2.36474718119154,2.11677107083992));
#75559=CARTESIAN_POINT('Ctrl Pts',(-6.58657864775301,2.40339272323902,2.11492597067985));
#75560=CARTESIAN_POINT('Ctrl Pts',(-6.57226800353884,2.44190905894539,2.1130822547889));
#75561=CARTESIAN_POINT('',(-7.01124999997673,-1.80655468318879E-5,2.77353435691037));
#75562=CARTESIAN_POINT('Ctrl Pts',(-6.57226793021667,2.4419092562881,2.66021763119828));
#75563=CARTESIAN_POINT('Ctrl Pts',(-6.63825067143893,2.26432024352436,2.66870420947979));
#75564=CARTESIAN_POINT('Ctrl Pts',(-6.69702941724246,2.08407313392669,2.67719508029717));
#75565=CARTESIAN_POINT('Ctrl Pts',(-6.78370868773811,1.77646480852692,2.69164819243435));
#75566=CARTESIAN_POINT('Ctrl Pts',(-6.81548338591757,1.65036835490453,2.69757167026797));
#75567=CARTESIAN_POINT('Ctrl Pts',(-6.88364107724175,1.34418898412278,2.71193582834949));
#75568=CARTESIAN_POINT('Ctrl Pts',(-6.91648900616039,1.16341643458372,2.72039248230661));
#75569=CARTESIAN_POINT('Ctrl Pts',(-6.97028931756841,0.782908825344512,
2.73807246531727));
#75570=CARTESIAN_POINT('Ctrl Pts',(-6.98983768873121,0.58313790210834,2.74728572145898));
#75571=CARTESIAN_POINT('Ctrl Pts',(-7.00776269506336,0.255320933964559,
2.76228116211942));
#75572=CARTESIAN_POINT('Ctrl Pts',(-7.0112500449107,0.127671648310814,2.76809066635348));
#75573=CARTESIAN_POINT('Ctrl Pts',(-7.01124999999957,-2.4663037176062E-6,
2.7738784608769));
#75574=CARTESIAN_POINT('Ctrl Pts',(-7.01124999997673,-1.80655468318879E-5,
2.77353435691037));
#75575=CARTESIAN_POINT('Ctrl Pts',(-7.01124950890869,-0.190601875733761,
2.7821841598315));
#75576=CARTESIAN_POINT('Ctrl Pts',(-7.00347383924979,-0.381166330084032,
2.79083396275264));
#75577=CARTESIAN_POINT('Ctrl Pts',(-6.98795373149948,-0.571077235514203,
2.79948376567377));
#75578=CARTESIAN_POINT('Ctrl Pts',(-6.97242834684876,-0.761052711432532,
2.80813650956344));
#75579=CARTESIAN_POINT('Ctrl Pts',(-6.94915328487888,-0.950373907584441,
2.81678925345311));
#75580=CARTESIAN_POINT('Ctrl Pts',(-6.91821124521096,-1.13841105455658,
2.82544199734278));
#75581=CARTESIAN_POINT('Ctrl Pts',(-6.88859135868876,-1.31841337551048,
2.83372500954457));
#75582=CARTESIAN_POINT('Ctrl Pts',(-6.85194608979608,-1.49723885436048,
2.84200802174635));
#75583=CARTESIAN_POINT('Ctrl Pts',(-6.80839202835472,-1.67434302063106,
2.85029103394815));
#75584=CARTESIAN_POINT('Ctrl Pts',(-6.76353436973175,-1.8567480126883,2.85882196129273));
#75585=CARTESIAN_POINT('Ctrl Pts',(-6.71133454211413,-2.03738050321834,
2.86735288863731));
#75586=CARTESIAN_POINT('Ctrl Pts',(-6.65195766392592,-2.21564568463399,
2.8758838159819));
#75587=CARTESIAN_POINT('Ctrl Pts',(-6.59259205836282,-2.39387702263074,
2.88441312374073));
#75588=CARTESIAN_POINT('Ctrl Pts',(-6.52605221807238,-2.56974165801549,
2.89294243149957));
#75589=CARTESIAN_POINT('Ctrl Pts',(-6.45255285871369,-2.74266078252594,
2.9014717392584));
#75590=CARTESIAN_POINT('Ctrl Pts',(-6.37527539811279,-2.92446850096178,
2.91043948061067));
#75591=CARTESIAN_POINT('Ctrl Pts',(-6.29030421808319,-3.10301957578802,
2.91940722196295));
#75592=CARTESIAN_POINT('Ctrl Pts',(-6.19794623826995,-3.27766517356722,
2.92837496331522));
#75593=CARTESIAN_POINT('Ctrl Pts',(-6.11010648638776,-3.4437669658245,2.93690399542397));
#75594=CARTESIAN_POINT('Ctrl Pts',(-6.01558555232828,-3.60633597361661,
2.94543302753274));
#75595=CARTESIAN_POINT('Ctrl Pts',(-5.91469479125556,-3.76483891936884,
2.95396205964149));
#75596=CARTESIAN_POINT('Ctrl Pts',(-5.81380302100902,-3.92334345056876,
2.96249117706308));
#75597=CARTESIAN_POINT('Ctrl Pts',(-5.70654146358684,-4.07778158189161,
2.97102029448466));
#75598=CARTESIAN_POINT('Ctrl Pts',(-5.59326525020323,-4.22764833014396,
2.97954941190625));
#75599=CARTESIAN_POINT('Ctrl Pts',(-5.47996611675168,-4.3775454021152,2.9880802550913));
#75600=CARTESIAN_POINT('Ctrl Pts',(-5.3606500820174,-4.52286899986246,2.99661109827635));
#75601=CARTESIAN_POINT('Ctrl Pts',(-5.23571360583634,-4.66314589093674,
3.0051419414614));
#75602=CARTESIAN_POINT('Ctrl Pts',(-5.21646633694138,-4.6847564495565,3.00645617280282));
#75603=CARTESIAN_POINT('Ctrl Pts',(-5.19708575200059,-4.70624729866498,
3.00777040414424));
#75604=CARTESIAN_POINT('Ctrl Pts',(-5.17757338267325,-4.72761678116294,
3.00908463548566));
#75605=CARTESIAN_POINT('Ctrl Pts',(-5.05091485599362,-4.86633018514231,
3.0176155628491));
#75606=CARTESIAN_POINT('Ctrl Pts',(-4.91865699422918,-4.999974402369,3.02614649021254));
#75607=CARTESIAN_POINT('Ctrl Pts',(-4.78122936540692,-5.12810611413907,
3.03467741757598));
#75608=CARTESIAN_POINT('Ctrl Pts',(-4.64382782704249,-5.25621350026916,
3.04320672535388));
#75609=CARTESIAN_POINT('Ctrl Pts',(-4.50125870411749,-5.37881026070913,
3.05173603313178));
#75610=CARTESIAN_POINT('Ctrl Pts',(-4.35398746275093,-5.49549085493805,
3.06026534090968));
#75611=CARTESIAN_POINT('Ctrl Pts',(-4.1991460108773,-5.61816920305433,3.06923308225247));
#75612=CARTESIAN_POINT('Ctrl Pts',(-4.03910657492292,-5.73430690843164,
3.07820082359527));
#75613=CARTESIAN_POINT('Ctrl Pts',(-3.87444908981545,-5.84348105267128,
3.08716856493806));
#75614=CARTESIAN_POINT('Ctrl Pts',(-3.71784678306701,-5.94731430880328,
3.0956975970661));
#75615=CARTESIAN_POINT('Ctrl Pts',(-3.55706774152558,-6.04484886281997,
3.10422662919414));
#75616=CARTESIAN_POINT('Ctrl Pts',(-3.39264050979283,-6.13576539103416,
3.11275566132219));
#75617=CARTESIAN_POINT('Ctrl Pts',(-3.22821163335349,-6.22668282865376,
3.12128477876308));
#75618=CARTESIAN_POINT('Ctrl Pts',(-3.06013476333635,-6.31098196286659,
3.12981389620397));
#75619=CARTESIAN_POINT('Ctrl Pts',(-2.88896334838836,-6.38838925975623,
3.13834301364486));
#75620=CARTESIAN_POINT('Ctrl Pts',(-2.71775729898345,-6.46581221907227,
3.14687385684908));
#75621=CARTESIAN_POINT('Ctrl Pts',(-2.54345573344074,-6.53634043054176,
3.15540470005329));
#75622=CARTESIAN_POINT('Ctrl Pts',(-2.36663320167697,-6.59974801422147,
3.16393554325751));
#75623=CARTESIAN_POINT('Ctrl Pts',(-2.33939255355957,-6.60951636024482,
3.16524977451273));
#75624=CARTESIAN_POINT('Ctrl Pts',(-2.31209210963559,-6.6191158039643,3.16656400576795));
#75625=CARTESIAN_POINT('Ctrl Pts',(-2.28473400769913,-6.62854562302796,
3.16787823702317));
#75626=CARTESIAN_POINT('Ctrl Pts',(-2.10714731632944,-6.6897563887316,3.1764091643825));
#75627=CARTESIAN_POINT('Ctrl Pts',(-1.92706894792116,-6.74383688423355,
3.18494009174182));
#75628=CARTESIAN_POINT('Ctrl Pts',(-1.74508821395569,-6.79060333755499,
3.19347101910115));
#75629=CARTESIAN_POINT('Ctrl Pts',(-1.5631420287983,-6.83736091232546,3.20200032687489));
#75630=CARTESIAN_POINT('Ctrl Pts',(-1.37929449525701,-6.87680713975774,
3.21052963464864));
#75631=CARTESIAN_POINT('Ctrl Pts',(-1.19414837369101,-6.90880859657518,
3.21905894242239));
#75632=CARTESIAN_POINT('Ctrl Pts',(-0.99948515209662,-6.94245503014401,
3.22802668376725));
#75633=CARTESIAN_POINT('Ctrl Pts',(-0.803386677535188,-6.96787108735875,
3.23699442511211));
#75634=CARTESIAN_POINT('Ctrl Pts',(-0.606564542512081,-6.98496285017087,
3.24596216645697));
#75635=CARTESIAN_POINT('Ctrl Pts',(-0.419371106869084,-7.00121847000559,
3.25449119858084));
#75636=CARTESIAN_POINT('Ctrl Pts',(-0.23152345263966,-7.00994476319048,
3.26302023070472));
#75637=CARTESIAN_POINT('Ctrl Pts',(-0.0436384824191531,-7.01111419428839,
3.27154926282859));
#75638=CARTESIAN_POINT('Ctrl Pts',(0.144248367147679,-7.0122836370837,3.28007838026534));
#75639=CARTESIAN_POINT('Ctrl Pts',(0.332172227240165,-7.00589606808603,
3.28860749770208));
#75640=CARTESIAN_POINT('Ctrl Pts',(0.519516233522091,-6.99197607587491,
3.29713661513882));
#75641=CARTESIAN_POINT('Ctrl Pts',(0.706898146589006,-6.97805326712237,
3.30566745833892));
#75642=CARTESIAN_POINT('Ctrl Pts',(0.89369966620886,-6.95659501469585,3.31419830153901));
#75643=CARTESIAN_POINT('Ctrl Pts',(1.07930819751002,-6.9276778488385,3.32272914473911));
#75644=CARTESIAN_POINT('Ctrl Pts',(1.10790238577609,-6.92322297341414,3.32404337601297));
#75645=CARTESIAN_POINT('Ctrl Pts',(1.13646827454602,-6.9185911723922,3.32535760728684));
#75646=CARTESIAN_POINT('Ctrl Pts',(1.1650036409725,-6.91378283423922,3.3266718385607));
#75647=CARTESIAN_POINT('Ctrl Pts',(1.3502321794825,-6.88257098871993,3.33520276591883));
#75648=CARTESIAN_POINT('Ctrl Pts',(1.53423739686404,-6.84390577530438,3.34373369327696));
#75649=CARTESIAN_POINT('Ctrl Pts',(1.71641388139953,-6.79790776270457,3.35226462063509));
#75650=CARTESIAN_POINT('Ctrl Pts',(1.89855577996322,-6.75191848276841,3.36079392840761));
#75651=CARTESIAN_POINT('Ctrl Pts',(2.07886934176505,-6.698599256705,3.36932323618013));
#75652=CARTESIAN_POINT('Ctrl Pts',(2.2567614335547,-6.63812130007581,3.37785254395265));
#75653=CARTESIAN_POINT('Ctrl Pts',(2.4437977451898,-6.57453458394159,3.38682028529812));
#75654=CARTESIAN_POINT('Ctrl Pts',(2.62815673930782,-6.50303389175604,3.39578802664358));
#75655=CARTESIAN_POINT('Ctrl Pts',(2.80916861474241,-6.42387719811378,3.40475576798904));
#75656=CARTESIAN_POINT('Ctrl Pts',(2.98132524155419,-6.34859291450363,3.41328480011165));
#75657=CARTESIAN_POINT('Ctrl Pts',(3.15045410658541,-6.2663839344867,3.42181383223426));
#75658=CARTESIAN_POINT('Ctrl Pts',(3.31600031773121,-6.17752122257031,3.43034286435687));
#75659=CARTESIAN_POINT('Ctrl Pts',(3.48154818477641,-6.08865762179206,3.43887198179233));
#75660=CARTESIAN_POINT('Ctrl Pts',(3.64351305807532,-5.99314030379713,3.44740109922778));
#75661=CARTESIAN_POINT('Ctrl Pts',(3.80136501676108,-5.89128598625504,3.45593021666324));
#75662=CARTESIAN_POINT('Ctrl Pts',(3.95924891487418,-5.78941105972843,3.46446105986206));
#75663=CARTESIAN_POINT('Ctrl Pts',(4.11301797942921,-5.68119673948677,3.47299190306088));
#75664=CARTESIAN_POINT('Ctrl Pts',(4.26217088908681,-5.56700331190138,3.4815227462597));
#75665=CARTESIAN_POINT('Ctrl Pts',(4.2851488544218,-5.54941107969777,3.4828369775392));
#75666=CARTESIAN_POINT('Ctrl Pts',(4.30801732288761,-5.53167702378405,3.4841512088187));
#75667=CARTESIAN_POINT('Ctrl Pts',(4.33077452839732,-5.51380254875753,3.48546544009821));
#75668=CARTESIAN_POINT('Ctrl Pts',(4.47849591515296,-5.39777590228194,3.49399636745846));
#75669=CARTESIAN_POINT('Ctrl Pts',(4.62157716411522,-5.27578953023405,3.50252729481871));
#75670=CARTESIAN_POINT('Ctrl Pts',(4.75954433094147,-5.14823895369115,3.51105822217896));
#75671=CARTESIAN_POINT('Ctrl Pts',(4.89748530487871,-5.02071259246101,3.51958752995363));
#75672=CARTESIAN_POINT('Ctrl Pts',(5.03031390947706,-4.88762434258184,3.5281168377283));
#75673=CARTESIAN_POINT('Ctrl Pts',(5.15759121336016,-4.74940832508326,3.53664614550298));
#75674=CARTESIAN_POINT('Ctrl Pts',(5.29141097580618,-4.60408756432229,3.54561388684737));
#75675=CARTESIAN_POINT('Ctrl Pts',(5.41909343978606,-4.45309823993976,3.55458162819177));
#75676=CARTESIAN_POINT('Ctrl Pts',(5.54017385785379,-4.29698733850281,3.56354936953617));
#75677=CARTESIAN_POINT('Ctrl Pts',(5.6553309231308,-4.14851350966971,3.57207840166097));
#75678=CARTESIAN_POINT('Ctrl Pts',(5.76451625571569,-3.99540749232178,3.58060743378577));
#75679=CARTESIAN_POINT('Ctrl Pts',(5.86737222757443,-3.83817270398146,3.58913646591057));
#75680=CARTESIAN_POINT('Ctrl Pts',(5.97022922826458,-3.68093634287791,3.59766558334822));
#75681=CARTESIAN_POINT('Ctrl Pts',(6.06675657681249,-3.51957138627459,3.60619470078588));
#75682=CARTESIAN_POINT('Ctrl Pts',(6.15664046272336,-3.35460948178137,3.61472381822353));
#75683=CARTESIAN_POINT('Ctrl Pts',(6.24654253554728,-3.18961419924956,3.62325466142454));
#75684=CARTESIAN_POINT('Ctrl Pts',(6.32979831521891,-3.0210207845251,3.63178550462556));
#75685=CARTESIAN_POINT('Ctrl Pts',(6.40613994976964,-2.84938546119429,3.64031634782657));
#75686=CARTESIAN_POINT('Ctrl Pts',(6.41790086963932,-2.82294393559193,3.64163057909629));
#75687=CARTESIAN_POINT('Ctrl Pts',(6.42949778486097,-2.79643025734872,3.64294481036601));
#75688=CARTESIAN_POINT('Ctrl Pts',(6.44092981658747,-2.76984650482558,3.64425904163573));
#75689=CARTESIAN_POINT('Ctrl Pts',(6.51513732820881,-2.59728626606002,3.65278996899439));
#75690=CARTESIAN_POINT('Ctrl Pts',(6.58241890750733,-2.42171261244503,3.66132089635305));
#75691=CARTESIAN_POINT('Ctrl Pts',(6.64254760027904,-2.24369961013662,3.66985182371172));
#75692=CARTESIAN_POINT('Ctrl Pts',(6.70266487769571,-2.06572040336788,3.67838113148479));
#75693=CARTESIAN_POINT('Ctrl Pts',(6.75563188060559,-1.88530306205903,3.68691043925785));
#75694=CARTESIAN_POINT('Ctrl Pts',(6.80127086794582,-1.70303879677815,3.69543974703092));
#75695=CARTESIAN_POINT('Ctrl Pts',(6.84925584452457,-1.51140556803342,3.70440748837612));
#75696=CARTESIAN_POINT('Ctrl Pts',(6.88913949303587,-1.31773088648166,3.71337522972131));
#75697=CARTESIAN_POINT('Ctrl Pts',(6.92077540079595,-1.1227174240376,3.7223429710665));
#75698=CARTESIAN_POINT('Ctrl Pts',(6.95086365414147,-0.937244179258234,
3.73087200318967));
#75699=CARTESIAN_POINT('Ctrl Pts',(6.97349179898842,-0.750560338373692,
3.73940103531284));
#75700=CARTESIAN_POINT('Ctrl Pts',(6.98858664232417,-0.563279065142881,
3.747930067436));
#75701=CARTESIAN_POINT('Ctrl Pts',(7.00368163664823,-0.375995918604626,
3.75645918487202));
#75702=CARTESIAN_POINT('Ctrl Pts',(7.01124315752175,-0.188115633246701,
3.76498830230804));
#75703=CARTESIAN_POINT('Ctrl Pts',(7.01124999535558,-0.000255198826522087,
3.77351741974405));
#75704=CARTESIAN_POINT('Ctrl Pts',(7.01125683457296,0.187643246871896,3.78204826294344));
#75705=CARTESIAN_POINT('Ctrl Pts',(7.00370593859617,0.375521527399259,3.79057910614282));
#75706=CARTESIAN_POINT('Ctrl Pts',(6.98862821308365,0.562763060080633,3.79910994934221));
#75707=CARTESIAN_POINT('Ctrl Pts',(6.98630539246772,0.591608822785914,3.80042418061922));
#75708=CARTESIAN_POINT('Ctrl Pts',(6.98380403514938,0.620439480036657,3.80173841189623));
#75709=CARTESIAN_POINT('Ctrl Pts',(6.98112436373805,0.649252786303629,3.80305264317324));
#75710=CARTESIAN_POINT('Ctrl Pts',(6.96373010250155,0.836285485229273,3.81158357053279));
#75711=CARTESIAN_POINT('Ctrl Pts',(6.93881229331357,1.02265077585319,3.82011449789233));
#75712=CARTESIAN_POINT('Ctrl Pts',(6.90644629163563,1.20773597414851,3.82864542525188));
#75713=CARTESIAN_POINT('Ctrl Pts',(6.87408643460146,1.3927860342571,3.83717473302585));
#75714=CARTESIAN_POINT('Ctrl Pts',(6.83428125964678,1.57655618552337,3.84570404079981));
#75715=CARTESIAN_POINT('Ctrl Pts',(6.78715753996745,1.75844223395679,3.85423334857377));
#75716=CARTESIAN_POINT('Ctrl Pts',(6.73761151108847,1.9496778042745,3.86320108991852));
#75717=CARTESIAN_POINT('Ctrl Pts',(6.67997480325776,2.13883011750153,3.87216883126327));
#75718=CARTESIAN_POINT('Ctrl Pts',(6.6144550262843,2.32521209092039,3.88113657260802));
#75719=CARTESIAN_POINT('Ctrl Pts',(6.55214053023832,2.50247610618643,3.88966560473209));
#75720=CARTESIAN_POINT('Ctrl Pts',(6.48269593291204,2.67723404533696,3.89819463685616));
#75721=CARTESIAN_POINT('Ctrl Pts',(6.40635031693033,2.84891245552871,3.90672366898024));
#75722=CARTESIAN_POINT('Ctrl Pts',(6.33000393729078,3.02059258295811,3.91525278641716));
#75723=CARTESIAN_POINT('Ctrl Pts',(6.24675652844298,3.18919284141453,3.92378190385409));
#75724=CARTESIAN_POINT('Ctrl Pts',(6.15688465148839,3.35416128872282,3.93231102129102));
#75725=CARTESIAN_POINT('Ctrl Pts',(6.0669945900506,3.5191631153936,3.94084186449131));
#75726=CARTESIAN_POINT('Ctrl Pts',(5.97047753066743,3.68053139474048,3.9493727076916));
#75727=CARTESIAN_POINT('Ctrl Pts',(5.86765560344639,3.83773947550433,3.95790355089189));
#75728=CARTESIAN_POINT('Ctrl Pts',(5.85181522411612,3.86195839164787,3.95921778216485));
#75729=CARTESIAN_POINT('Ctrl Pts',(5.83582529391221,3.88607862615853,3.9605320134378));
#75730=CARTESIAN_POINT('Ctrl Pts',(5.81968708264017,3.91009831368102,3.96184624471076));
#75731=CARTESIAN_POINT('Ctrl Pts',(5.71493085677523,4.06601471413551,3.97037717206993));
#75732=CARTESIAN_POINT('Ctrl Pts',(5.60388731357084,4.217745562263,3.97890809942909));
#75733=CARTESIAN_POINT('Ctrl Pts',(5.48691575044627,4.36478889638487,3.98743902678826));
#75734=CARTESIAN_POINT('Ctrl Pts',(5.36996639422247,4.51180431451893,3.99596833456184));
#75735=CARTESIAN_POINT('Ctrl Pts',(5.24709145452818,4.65413375504888,4.00449764233543));
#75736=CARTESIAN_POINT('Ctrl Pts',(5.11869131816443,4.79130731135545,4.01302695010901));
#75737=CARTESIAN_POINT('Ctrl Pts',(4.98369100604868,4.93553202512795,4.02199469145395));
#75738=CARTESIAN_POINT('Ctrl Pts',(4.84258274711559,5.07405656068499,4.03096243279889));
#75739=CARTESIAN_POINT('Ctrl Pts',(4.69587756928842,5.20637689922213,4.03993017414383));
#75740=CARTESIAN_POINT('Ctrl Pts',(4.55634932842262,5.33222401886917,4.04845920626751));
#75741=CARTESIAN_POINT('Ctrl Pts',(4.41175893808063,5.45245924004647,4.0569882383912));
#75742=CARTESIAN_POINT('Ctrl Pts',(4.26258191820052,5.56668859854133,4.06551727051488));
#75743=CARTESIAN_POINT('Ctrl Pts',(4.1134034061561,5.68091909963155,4.07404638795142));
#75744=CARTESIAN_POINT('Ctrl Pts',(3.95963841797951,5.78914343441517,4.08257550538796));
#75745=CARTESIAN_POINT('Ctrl Pts',(3.80179387437706,5.89100924284193,4.0911046228245));
#75746=CARTESIAN_POINT('Ctrl Pts',(3.64391739284751,5.99289566257834,4.09963546602441));
#75747=CARTESIAN_POINT('Ctrl Pts',(3.48195996501132,6.08842082102823,4.10816630922431));
#75748=CARTESIAN_POINT('Ctrl Pts',(3.3164564270066,6.17727636829264,4.11669715242422));
#75749=CARTESIAN_POINT('Ctrl Pts',(3.29095954227667,6.19096513696506,4.1180113836989));
#75750=CARTESIAN_POINT('Ctrl Pts',(3.2653785451568,6.20449570123017,4.11932561497359));
#75751=CARTESIAN_POINT('Ctrl Pts',(3.23971544313659,6.2178670305823,4.12063984624828));
#75752=CARTESIAN_POINT('Ctrl Pts',(3.07313132406655,6.30466289490009,4.12917077360755));
#75753=CARTESIAN_POINT('Ctrl Pts',(2.90302863634734,6.38477528091143,4.13770170096682));
#75754=CARTESIAN_POINT('Ctrl Pts',(2.72996304149713,6.45793530120578,4.14623262832609));
#75755=CARTESIAN_POINT('Ctrl Pts',(2.55693030292749,6.53108143216437,4.15476193609977));
#75756=CARTESIAN_POINT('Ctrl Pts',(2.38093606167818,6.59727771222868,4.16329124387345));
#75757=CARTESIAN_POINT('Ctrl Pts',(2.20255672486121,6.65630306072888,4.17182055164714));
#75758=CARTESIAN_POINT('Ctrl Pts',(2.01500812229077,6.71836250003942,4.18078829299203));
#75759=CARTESIAN_POINT('Ctrl Pts',(1.82482310199486,6.77249424437683,4.18975603433691));
#75760=CARTESIAN_POINT('Ctrl Pts',(1.6326915482164,6.8185001921891,4.1987237756818));
#75761=CARTESIAN_POINT('Ctrl Pts',(1.44995922676027,6.86225549150978,4.20725280780559));
#75762=CARTESIAN_POINT('Ctrl Pts',(1.2654665940685,6.89866095640306,4.21578183992937));
#75763=CARTESIAN_POINT('Ctrl Pts',(1.07981970058149,6.92759813909093,4.22431087205316));
#75764=CARTESIAN_POINT('Ctrl Pts',(0.894170950134817,6.95653561122712,4.23283998948981));
#75765=CARTESIAN_POINT('Ctrl Pts',(0.707368218865288,6.9780046079314,4.24136910692647));
#75766=CARTESIAN_POINT('Ctrl Pts',(0.520025226413481,6.9919382381707,4.24989822436312));
#75767=CARTESIAN_POINT('Ctrl Pts',(0.33264432738187,7.0058746877109,4.25842906756313));
#75768=CARTESIAN_POINT('Ctrl Pts',(0.144723254268758,7.01227270373496,4.26695991076313));
#75769=CARTESIAN_POINT('Ctrl Pts',(-0.0431208157453261,7.01111739723059,
4.27549075396314));
#75770=CARTESIAN_POINT('Ctrl Pts',(-0.0720594031394497,7.01093941483146,
4.27680498523736));
#75771=CARTESIAN_POINT('Ctrl Pts',(-0.100996162252054,7.01058226718464,
4.27811921651158));
#75772=CARTESIAN_POINT('Ctrl Pts',(-0.129928837230052,7.01004600981734,
4.27943344778579));
#75773=CARTESIAN_POINT('Ctrl Pts',(-0.317736381753391,7.00656506035585,
4.28796437514507));
#75774=CARTESIAN_POINT('Ctrl Pts',(-0.505436103814094,6.99553178794519,
4.29649530250434));
#75775=CARTESIAN_POINT('Ctrl Pts',(-0.692411418918306,6.9769759200854,4.30502622986361));
#75776=CARTESIAN_POINT('Ctrl Pts',(-0.87935123699947,6.95842357503326,4.31355553763729));
#75777=CARTESIAN_POINT('Ctrl Pts',(-1.06556661800272,6.93235151479403,4.32208484541098));
#75778=CARTESIAN_POINT('Ctrl Pts',(-1.25044563231558,6.89884137251487,4.33061415318467));
#75779=CARTESIAN_POINT('Ctrl Pts',(-1.44482801649572,6.8636087022486,4.33958189452955));
#75780=CARTESIAN_POINT('Ctrl Pts',(-1.6377326689979,6.82015317632885,4.34854963587444));
#75781=CARTESIAN_POINT('Ctrl Pts',(-1.82845900684053,6.76863089722019,4.35751737721933));
#75782=CARTESIAN_POINT('Ctrl Pts',(-2.00985485667058,6.7196291300295,4.36604640934311));
#75783=CARTESIAN_POINT('Ctrl Pts',(-2.18928010797788,6.66333109644986,4.3745754414669));
#75784=CARTESIAN_POINT('Ctrl Pts',(-2.3661459031183,6.59992273649143,4.38310447359068));
#75785=CARTESIAN_POINT('Ctrl Pts',(-2.54301346738409,6.53651374228183,4.39163359102733));
#75786=CARTESIAN_POINT('Ctrl Pts',(-2.71732123718675,6.4659943859631,4.40016270846398));
#75787=CARTESIAN_POINT('Ctrl Pts',(-2.88849828659866,6.38859955004355,4.40869182590062));
#75788=CARTESIAN_POINT('Ctrl Pts',(-3.05970997160829,6.31118905421859,4.41722266910063));
#75789=CARTESIAN_POINT('Ctrl Pts',(-3.22778939237545,6.22690042720623,4.42575351230064));
#75790=CARTESIAN_POINT('Ctrl Pts',(-3.39218746609123,6.13601587004089,4.43428435550065));
#75791=CARTESIAN_POINT('Ctrl Pts',(-3.4175140469265,6.12201451934559,4.43559858677487));
#75792=CARTESIAN_POINT('Ctrl Pts',(-3.44275330444796,6.10785671364891,4.43691281804908));
#75793=CARTESIAN_POINT('Ctrl Pts',(-3.46790328429765,6.09354358097631,4.4382270493233));
#75794=CARTESIAN_POINT('Ctrl Pts',(-3.63115662896687,6.00063429057287,4.44675797668256));
#75795=CARTESIAN_POINT('Ctrl Pts',(-3.79070204152074,5.90114469265081,4.45528890404183));
#75796=CARTESIAN_POINT('Ctrl Pts',(-3.94601230543783,5.795395883616,4.46381983140109));
#75797=CARTESIAN_POINT('Ctrl Pts',(-4.10129308390098,5.68966715085663,4.47234913917476));
#75798=CARTESIAN_POINT('Ctrl Pts',(-4.25234006527787,5.57768175062914,4.48087844694843));
#75799=CARTESIAN_POINT('Ctrl Pts',(-4.39865495378781,5.45980413201957,4.4894077547221));
#75800=CARTESIAN_POINT('Ctrl Pts',(-4.55249089333668,5.33586722856935,4.498375496067));
#75801=CARTESIAN_POINT('Ctrl Pts',(-4.70109514525235,5.20541660954974,4.50734323741189));
#75802=CARTESIAN_POINT('Ctrl Pts',(-4.84392719318669,5.06892453185156,4.51631097875679));
#75803=CARTESIAN_POINT('Ctrl Pts',(-4.97977178083524,4.93910975792403,4.52484001088056));
#75804=CARTESIAN_POINT('Ctrl Pts',(-5.11039518872745,4.80383073256485,4.53336904300433));
#75805=CARTESIAN_POINT('Ctrl Pts',(-5.23536928461244,4.66353246115396,4.5418980751281));
#75806=CARTESIAN_POINT('Ctrl Pts',(-5.36034463056847,4.52323278638979,4.55042719256472));
#75807=CARTESIAN_POINT('Ctrl Pts',(-5.47967035035606,4.3779139960489,4.55895631000134));
#75808=CARTESIAN_POINT('Ctrl Pts',(-5.59295747354586,4.22805549414947,4.56748542743796));
#75809=CARTESIAN_POINT('Ctrl Pts',(-5.70626751901026,4.07816667020076,4.57601627063799));
#75810=CARTESIAN_POINT('Ctrl Pts',(-5.81353634358416,3.92373654488918,4.58454711383802));
#75811=CARTESIAN_POINT('Ctrl Pts',(-5.91441679640935,3.7652756234904,4.59307795703805));
#75812=CARTESIAN_POINT('Ctrl Pts',(-5.92995807913555,3.74086369916269,4.59439218831231));
#75813=CARTESIAN_POINT('Ctrl Pts',(-5.94534782835778,3.71635616560023,4.59570641958657));
#75814=CARTESIAN_POINT('Ctrl Pts',(-5.96058486758315,3.69175494837331,4.59702065086083));
#75815=CARTESIAN_POINT('Ctrl Pts',(-6.05949047898495,3.53206523470464,4.60555149768623));
#75816=CARTESIAN_POINT('Ctrl Pts',(-6.15199196890276,3.36837123830459,4.61408234451163));
#75817=CARTESIAN_POINT('Ctrl Pts',(-6.23778000506086,3.20120714277645,4.62261319133703));
#75818=CARTESIAN_POINT('Ctrl Pts',(-6.32355367648331,3.03407103795832,4.63114260971897));
#75819=CARTESIAN_POINT('Ctrl Pts',(-6.40261599694051,2.86346626546418,4.6396720281009));
#75820=CARTESIAN_POINT('Ctrl Pts',(-6.4747037524723,2.68995127841028,4.64820144648284));
#75821=CARTESIAN_POINT('Ctrl Pts',(-6.50879210205942,2.60790073468528,4.65223477771133));
#75822=CARTESIAN_POINT('Ctrl Pts',(-6.54132155604487,2.52519977118959,4.65626810893982));
#75823=CARTESIAN_POINT('Ctrl Pts',(-6.57226799596304,2.44190907933527,4.66030144016832));
#75824=CARTESIAN_POINT('Origin',(0.,0.,10.));
#75825=CARTESIAN_POINT('',(-6.57226799589878,2.4419090795082,6.65995074817407));
#75826=CARTESIAN_POINT('',(-6.57226799596303,2.44190907933528,6.1132300454328));
#75827=CARTESIAN_POINT('',(-6.57226799596304,2.44190907933527,10.));
#75828=CARTESIAN_POINT('',(-7.01124999902813,-0.000116739559371617,4.22646564308964));
#75829=CARTESIAN_POINT('Ctrl Pts',(-6.57226799596304,2.44190907933527,6.1132300454328));
#75830=CARTESIAN_POINT('Ctrl Pts',(-6.50682618162574,2.61804223089546,6.10470102768527));
#75831=CARTESIAN_POINT('Ctrl Pts',(-6.43429998856149,2.79154289620592,6.09617200993773));
#75832=CARTESIAN_POINT('Ctrl Pts',(-6.35492875623202,2.96184183671502,6.0876429921902));
#75833=CARTESIAN_POINT('Ctrl Pts',(-6.2719715608649,3.13983482062113,6.07872863656278));
#75834=CARTESIAN_POINT('Ctrl Pts',(-6.18153660119697,3.31432972798643,6.06981428093535));
#75835=CARTESIAN_POINT('Ctrl Pts',(-6.08395206666282,3.48470282994824,6.06089992530793));
#75836=CARTESIAN_POINT('Ctrl Pts',(-5.98636753212867,3.65507593191004,6.05198556968051));
#75837=CARTESIAN_POINT('Ctrl Pts',(-5.88163362047875,3.82132690206206,6.04307121405308));
#75838=CARTESIAN_POINT('Ctrl Pts',(-5.77013196163399,3.98286375712626,6.03415685842566));
#75839=CARTESIAN_POINT('Ctrl Pts',(-5.66342626222106,4.13745251642524,6.02562593106641));
#75840=CARTESIAN_POINT('Ctrl Pts',(-5.55048629613543,4.28777710796666,6.01709500370717));
#75841=CARTESIAN_POINT('Ctrl Pts',(-5.43167763524909,4.43334012108645,6.00856407634793));
#75842=CARTESIAN_POINT('Ctrl Pts',(-5.31289153003419,4.57887549925546,6.00003476857427));
#75843=CARTESIAN_POINT('Ctrl Pts',(-5.18823914698469,4.71965086587602,5.99150546080061));
#75844=CARTESIAN_POINT('Ctrl Pts',(-5.05812674162247,4.85520137874668,5.98297615302695));
#75845=CARTESIAN_POINT('Ctrl Pts',(-4.92132614443279,4.99771961948207,5.97400841168205));
#75846=CARTESIAN_POINT('Ctrl Pts',(-4.77848965503702,5.13446143820321,5.96504067033714));
#75847=CARTESIAN_POINT('Ctrl Pts',(-4.63013458967959,5.26492927245492,5.95607292899224));
#75848=CARTESIAN_POINT('Ctrl Pts',(-4.48903717512546,5.38901451383876,5.94754389686848));
#75849=CARTESIAN_POINT('Ctrl Pts',(-4.3429484747963,5.50742473733119,5.93901486474473));
#75850=CARTESIAN_POINT('Ctrl Pts',(-4.19234891787301,5.61977198054414,5.93048583262097));
#75851=CARTESIAN_POINT('Ctrl Pts',(-4.04174785455652,5.73212034752616,5.92195671518437));
#75852=CARTESIAN_POINT('Ctrl Pts',(-3.88663609185215,5.8384054325547,5.91342759774777));
#75853=CARTESIAN_POINT('Ctrl Pts',(-3.72752493483961,5.93828126840157,5.90489848031117));
#75854=CARTESIAN_POINT('Ctrl Pts',(-3.56838158361615,6.03817731291128,5.89636763711121));
#75855=CARTESIAN_POINT('Ctrl Pts',(-3.40523748165395,6.13166135606096,5.88783679391125));
#75856=CARTESIAN_POINT('Ctrl Pts',(-3.23863129465954,6.21843178781852,5.87930595071128));
#75857=CARTESIAN_POINT('Ctrl Pts',(-3.2129645397654,6.2317993310302,5.8779917194369));
#75858=CARTESIAN_POINT('Ctrl Pts',(-3.18721566557292,6.24500762616669,5.87667748816252));
#75859=CARTESIAN_POINT('Ctrl Pts',(-3.16138669235278,6.25805566801021,5.87536325688813));
#75860=CARTESIAN_POINT('Ctrl Pts',(-2.99372587146071,6.34275301110139,5.86683232952888));
#75861=CARTESIAN_POINT('Ctrl Pts',(-2.82263067900426,6.42072322259215,5.85830140216962));
#75862=CARTESIAN_POINT('Ctrl Pts',(-2.64866010892576,6.49170441331746,5.84977047481036));
#75863=CARTESIAN_POINT('Ctrl Pts',(-2.47472256693643,6.56267212835492,5.8412411670367));
#75864=CARTESIAN_POINT('Ctrl Pts',(-2.29791102008881,6.62665335488609,5.83271185926305));
#75865=CARTESIAN_POINT('Ctrl Pts',(-2.11880460600824,6.68343426720562,5.82418255148939));
#75866=CARTESIAN_POINT('Ctrl Pts',(-1.93049155208761,6.74313389917122,5.81521481014449));
#75867=CARTESIAN_POINT('Ctrl Pts',(-1.739641830731,6.79487335749993,5.80624706879959));
#75868=CARTESIAN_POINT('Ctrl Pts',(-1.54694775921635,6.83846321864463,5.7972793274547));
#75869=CARTESIAN_POINT('Ctrl Pts',(-1.36368043885101,6.87992062822809,5.78875029533093));
#75870=CARTESIAN_POINT('Ctrl Pts',(-1.17874523268746,6.91400667981452,5.78022126320716));
#75871=CARTESIAN_POINT('Ctrl Pts',(-0.992749630653989,6.94061054470977,
5.77169223108339));
#75872=CARTESIAN_POINT('Ctrl Pts',(-0.806752168172955,6.96721467571397,
5.76316311364676));
#75873=CARTESIAN_POINT('Ctrl Pts',(-0.619694592198527,6.98633643033115,
5.75463399621012));
#75874=CARTESIAN_POINT('Ctrl Pts',(-0.432191413893036,6.99791662884441,
5.74610487877349));
#75875=CARTESIAN_POINT('Ctrl Pts',(-0.244650296596127,7.00949917047024,
5.73757403557351));
#75876=CARTESIAN_POINT('Ctrl Pts',(-0.0566637025728533,7.01353709027643,
5.72904319237352));
#75877=CARTESIAN_POINT('Ctrl Pts',(0.131151052699608,7.01002324988126,5.72051234917354));
#75878=CARTESIAN_POINT('Ctrl Pts',(0.160085123971154,7.00948192016367,5.71919811789924));
#75879=CARTESIAN_POINT('Ctrl Pts',(0.189015117454169,7.008761462279,5.71788388662494));
#75880=CARTESIAN_POINT('Ctrl Pts',(0.217938778170615,7.00786196007524,5.71656965535063));
#75881=CARTESIAN_POINT('Ctrl Pts',(0.405687809380714,7.0020231186857,5.70803872799135));
#75882=CARTESIAN_POINT('Ctrl Pts',(0.593234197456993,6.98863390357214,5.69950780063207));
#75883=CARTESIAN_POINT('Ctrl Pts',(0.779961779780187,6.96773178190594,5.69097687327279));
#75884=CARTESIAN_POINT('Ctrl Pts',(0.966653912111869,6.94683362848067,5.68244756549911));
#75885=CARTESIAN_POINT('Ctrl Pts',(1.15252724473683,6.91842544891597,5.67391825772542));
#75886=CARTESIAN_POINT('Ctrl Pts',(1.33697092129266,6.8825965534904,5.66538894995174));
#75887=CARTESIAN_POINT('Ctrl Pts',(1.53089558996927,6.8449259387846,5.65642120860685));
#75888=CARTESIAN_POINT('Ctrl Pts',(1.72323939488692,6.79905167149075,5.64745346726196));
#75889=CARTESIAN_POINT('Ctrl Pts',(1.91330376836143,6.74513863849172,5.63848572591708));
#75890=CARTESIAN_POINT('Ctrl Pts',(2.09407003766044,6.69386307504092,5.62995669379328));
#75891=CARTESIAN_POINT('Ctrl Pts',(2.27277424973527,6.63531656380038,5.62142766166948));
#75892=CARTESIAN_POINT('Ctrl Pts',(2.44882992808045,6.56969242399045,5.61289862954568));
#75893=CARTESIAN_POINT('Ctrl Pts',(2.62488736744776,6.50406762776567,5.60436951210902));
#75894=CARTESIAN_POINT('Ctrl Pts',(2.7982959343672,6.43136517149171,5.59584039467236));
#75895=CARTESIAN_POINT('Ctrl Pts',(2.96848769717246,6.35182708787289,5.58731127723569));
#75896=CARTESIAN_POINT('Ctrl Pts',(3.13871389621424,6.2722729106887,5.57878043403569));
#75897=CARTESIAN_POINT('Ctrl Pts',(3.30572171411774,6.1858804741672,5.57024959083568));
#75898=CARTESIAN_POINT('Ctrl Pts',(3.46896565475864,6.09293885153995,5.56171874763568));
#75899=CARTESIAN_POINT('Ctrl Pts',(3.49411443396873,6.0786205966773,5.56040451636149));
#75900=CARTESIAN_POINT('Ctrl Pts',(3.51917393225434,6.06414699560415,5.55909028508729));
#75901=CARTESIAN_POINT('Ctrl Pts',(3.54414220957539,6.04951920079655,5.5577760538131));
#75902=CARTESIAN_POINT('Ctrl Pts',(3.70621608827091,5.95456737809983,5.54924512645385));
#75903=CARTESIAN_POINT('Ctrl Pts',(3.86449970289803,5.85308232450999,5.5407141990946));
#75904=CARTESIAN_POINT('Ctrl Pts',(4.01846991027773,5.7453917310043,5.53218327173535));
#75905=CARTESIAN_POINT('Ctrl Pts',(4.17241088661168,5.63772158241921,5.52365396396169));
#75906=CARTESIAN_POINT('Ctrl Pts',(4.32203983908092,5.5238484203919,5.51512465618802));
#75907=CARTESIAN_POINT('Ctrl Pts',(4.46686308731619,5.40414292202492,5.50659534841436));
#75908=CARTESIAN_POINT('Ctrl Pts',(4.61913071153202,5.2782841799789,5.49762760706946));
#75909=CARTESIAN_POINT('Ctrl Pts',(4.76608527243226,5.14597792645828,5.48865986572457));
#75910=CARTESIAN_POINT('Ctrl Pts',(4.90719222607484,5.00770316800534,5.47969212437967));
#75911=CARTESIAN_POINT('Ctrl Pts',(5.04139611245137,4.87619292351969,5.4711630922559));
#75912=CARTESIAN_POINT('Ctrl Pts',(5.17031061993882,4.73928441702447,5.46263406013213));
#75913=CARTESIAN_POINT('Ctrl Pts',(5.29351323765484,4.59742799457186,5.45410502800836));
#75914=CARTESIAN_POINT('Ctrl Pts',(5.41671708772249,4.45557015318029,5.44557591057174));
#75915=CARTESIAN_POINT('Ctrl Pts',(5.53420873552052,4.30876453024073,5.43704679313512));
#75916=CARTESIAN_POINT('Ctrl Pts',(5.64560526082019,4.15749537600457,5.4285176756985));
#75917=CARTESIAN_POINT('Ctrl Pts',(5.7570243258543,4.00619561429161,5.41998683249852));
#75918=CARTESIAN_POINT('Ctrl Pts',(5.86234562434225,3.85043076455449,5.41145598929854));
#75919=CARTESIAN_POINT('Ctrl Pts',(5.96122844284613,3.69071565075153,5.40292514609856));
#75920=CARTESIAN_POINT('Ctrl Pts',(5.97646197715504,3.66611051001443,5.40161091482424));
#75921=CARTESIAN_POINT('Ctrl Pts',(5.9915427894084,3.64141167027867,5.40029668354992));
#75922=CARTESIAN_POINT('Ctrl Pts',(6.0064697273841,3.61662107173511,5.3989824522756));
#75923=CARTESIAN_POINT('Ctrl Pts',(6.10336334577159,3.45570054009038,5.39045152491632));
#75924=CARTESIAN_POINT('Ctrl Pts',(6.19380294666506,3.29085637928391,5.38192059755705));
#75925=CARTESIAN_POINT('Ctrl Pts',(6.27748592118411,3.1226266302322,5.37338967019778));
#75926=CARTESIAN_POINT('Ctrl Pts',(6.36115300859805,2.95442881938204,5.36486036242409));
#75927=CARTESIAN_POINT('Ctrl Pts',(6.43806589316049,2.78284697699901,5.35633105465041));
#75928=CARTESIAN_POINT('Ctrl Pts',(6.5079684038665,2.60844279538106,5.34780174687673));
#75929=CARTESIAN_POINT('Ctrl Pts',(6.58146412614586,2.42507368364114,5.33883400553184));
#75930=CARTESIAN_POINT('Ctrl Pts',(6.64720963161899,2.23858476654406,5.32986626418695));
#75931=CARTESIAN_POINT('Ctrl Pts',(6.7049646938521,2.04965241362939,5.32089852284206));
#75932=CARTESIAN_POINT('Ctrl Pts',(6.75989433133306,1.86996278552131,5.31236949071827));
#75933=CARTESIAN_POINT('Ctrl Pts',(6.80759654130547,1.68806339422104,5.30384045859448));
#75934=CARTESIAN_POINT('Ctrl Pts',(6.84791576449454,1.50455184187423,5.29531142647069));
#75935=CARTESIAN_POINT('Ctrl Pts',(6.88823539098236,1.3210384539271,5.28678230903405));
#75936=CARTESIAN_POINT('Ctrl Pts',(6.92117182057933,1.13591317247005,5.27825319159741));
#75937=CARTESIAN_POINT('Ctrl Pts',(6.94662048035468,0.949784430498304,5.26972407416076));
#75938=CARTESIAN_POINT('Ctrl Pts',(6.97207428935737,0.76361802763528,5.26119323096075));
#75939=CARTESIAN_POINT('Ctrl Pts',(6.99003726194707,0.576448062243412,5.25266238776075));
#75940=CARTESIAN_POINT('Ctrl Pts',(7.00045651543156,0.388889621938999,5.24413154456074));
#75941=CARTESIAN_POINT('Ctrl Pts',(7.00206166845832,0.359995037639062,5.24281731328651));
#75942=CARTESIAN_POINT('Ctrl Pts',(7.00348788392251,0.33109124045191,5.24150308201229));
#75943=CARTESIAN_POINT('Ctrl Pts',(7.00473507827124,0.302180485366532,5.24018885073807));
#75944=CARTESIAN_POINT('Ctrl Pts',(7.01283085608495,0.114515227073064,5.23165792337883));
#75945=CARTESIAN_POINT('Ctrl Pts',(7.01338201380923,-0.073507683729425,
5.22312699601959));
#75946=CARTESIAN_POINT('Ctrl Pts',(7.00638023702977,-0.261271002330286,
5.21459606866036));
#75947=CARTESIAN_POINT('Ctrl Pts',(6.99937978952862,-0.448998674306648,
5.2060667608867));
#75948=CARTESIAN_POINT('Ctrl Pts',(6.98482928045914,-0.636466546575077,
5.19753745311305));
#75949=CARTESIAN_POINT('Ctrl Pts',(6.96277248923073,-0.823058822753118,
5.1890081453394));
#75950=CARTESIAN_POINT('Ctrl Pts',(6.93958190871891,-1.01924253591332,5.18004040399449));
#75951=CARTESIAN_POINT('Ctrl Pts',(6.90809305412251,-1.2144579034598,5.17107266264959));
#75952=CARTESIAN_POINT('Ctrl Pts',(6.86841857111615,-1.40799605626111,5.16210492130469));
#75953=CARTESIAN_POINT('Ctrl Pts',(6.83068499617901,-1.59206616476769,5.15357588918093));
#75954=CARTESIAN_POINT('Ctrl Pts',(6.78554761272565,-1.77461891332654,5.14504685705717));
#75955=CARTESIAN_POINT('Ctrl Pts',(6.73315573027801,-1.95505510774619,5.13651782493341));
#75956=CARTESIAN_POINT('Ctrl Pts',(6.68076332377311,-2.13549310700452,5.1279887074968));
#75957=CARTESIAN_POINT('Ctrl Pts',(6.6211163617703,-2.3138142166712,5.11945959006018));
#75958=CARTESIAN_POINT('Ctrl Pts',(6.55441410803044,-2.48943412504762,5.11093047262357));
#75959=CARTESIAN_POINT('Ctrl Pts',(6.48769835789936,-2.6650895679803,5.10239962942359));
#75960=CARTESIAN_POINT('Ctrl Pts',(6.41392457437037,-2.83804243205775,5.09386878622361));
#75961=CARTESIAN_POINT('Ctrl Pts',(6.33334059552266,-3.0077272920936,5.08533794302364));
#75962=CARTESIAN_POINT('Ctrl Pts',(6.32092611517982,-3.03386833637455,5.08402371174928));
#75963=CARTESIAN_POINT('Ctrl Pts',(6.30835009735642,-3.05993186181274,5.08270948047492));
#75964=CARTESIAN_POINT('Ctrl Pts',(6.29561354753464,-3.08591584826908,5.08139524920056));
#75965=CARTESIAN_POINT('Ctrl Pts',(6.21293815891969,-3.25458288982304,5.07286432184127));
#75966=CARTESIAN_POINT('Ctrl Pts',(6.12346653013996,-3.4199544303172,5.06433339448198));
#75967=CARTESIAN_POINT('Ctrl Pts',(6.02748666786519,-3.58148447312109,5.05580246712268));
#75968=CARTESIAN_POINT('Ctrl Pts',(5.93152502724389,-3.742983849654,5.04727315934899));
#75969=CARTESIAN_POINT('Ctrl Pts',(5.82905777520455,-3.90064292077555,5.03874385157529));
#75970=CARTESIAN_POINT('Ctrl Pts',(5.72041797044794,-4.05394188486667,5.03021454380159));
#75971=CARTESIAN_POINT('Ctrl Pts',(5.60619373389035,-4.21512090371347,5.02124680245671));
#75972=CARTESIAN_POINT('Ctrl Pts',(5.48514584979072,-4.37147945782832,5.01227906111183));
#75973=CARTESIAN_POINT('Ctrl Pts',(5.35771237882704,-4.52244896358859,5.00331131976695));
#75974=CARTESIAN_POINT('Ctrl Pts',(5.23651305720318,-4.66603291798977,4.99478228764314));
#75975=CARTESIAN_POINT('Ctrl Pts',(5.10953820610217,-4.80474224204438,4.98625325551933));
#75976=CARTESIAN_POINT('Ctrl Pts',(4.97720561001534,-4.93812220161995,4.97772422339552));
#75977=CARTESIAN_POINT('Ctrl Pts',(4.84487169025308,-5.07150349534734,4.96919510595887));
#75978=CARTESIAN_POINT('Ctrl Pts',(4.70718013637788,-5.19955510299314,4.96066598852221));
#75979=CARTESIAN_POINT('Ctrl Pts',(4.56458547879249,-5.32185925868927,4.95213687108556));
#75980=CARTESIAN_POINT('Ctrl Pts',(4.42196196890907,-5.44418816114669,4.94360602788553));
#75981=CARTESIAN_POINT('Ctrl Pts',(4.27443360685816,-5.56076709028839,4.93507518468549));
#75982=CARTESIAN_POINT('Ctrl Pts',(4.12248854157041,-5.67121810435119,4.92654434148546));
#75983=CARTESIAN_POINT('Ctrl Pts',(4.09908042679551,-5.68823379360236,4.92523011021132));
#75984=CARTESIAN_POINT('Ctrl Pts',(4.07556754898422,-5.70510412730741,4.92391587893717));
#75985=CARTESIAN_POINT('Ctrl Pts',(4.05195175756997,-5.72182781258101,4.92260164766303));
#75986=CARTESIAN_POINT('Ctrl Pts',(3.89865712438774,-5.83038446243039,4.91407072030376));
#75987=CARTESIAN_POINT('Ctrl Pts',(3.7409711977267,-5.93279572789841,4.90553979294449));
#75988=CARTESIAN_POINT('Ctrl Pts',(3.57940810442595,-6.02871994576543,4.89700886558523));
#75989=CARTESIAN_POINT('Ctrl Pts',(3.41787568367046,-6.12462595254317,4.88847955781154));
#75990=CARTESIAN_POINT('Ctrl Pts',(3.25246782836903,-6.214047213169,4.87995025003785));
#75991=CARTESIAN_POINT('Ctrl Pts',(3.08372569427774,-6.29668662114856,4.87142094226416));
#75992=CARTESIAN_POINT('Ctrl Pts',(2.90630967733171,-6.38357395776705,4.86245320091927));
#75993=CARTESIAN_POINT('Ctrl Pts',(2.7252078866279,-6.46296368691272,4.85348545957438));
#75994=CARTESIAN_POINT('Ctrl Pts',(2.54107702163888,-6.534566101326,4.8445177182295));
#75995=CARTESIAN_POINT('Ctrl Pts',(2.36595398875084,-6.60266566722391,4.83598868610571));
#75996=CARTESIAN_POINT('Ctrl Pts',(2.18809147647589,-6.66372151148867,4.82745965398192));
#75997=CARTESIAN_POINT('Ctrl Pts',(2.00807391033646,-6.71753420036892,4.81893062185814));
#75998=CARTESIAN_POINT('Ctrl Pts',(1.8280545435459,-6.77134742751818,4.8104015044215));
#75999=CARTESIAN_POINT('Ctrl Pts',(1.64588037411524,-6.81791726992009,4.80187238698487));
#76000=CARTESIAN_POINT('Ctrl Pts',(1.46215040842561,-6.85709433693608,4.79334326954823));
#76001=CARTESIAN_POINT('Ctrl Pts',(1.27838326720818,-6.89627933095591,4.78481242634824));
#76002=CARTESIAN_POINT('Ctrl Pts',(1.09306000066022,-6.9280684989995,4.77628158314825));
#76003=CARTESIAN_POINT('Ctrl Pts',(0.906790083467169,-6.95236350509851,
4.76775073994825));
#76004=CARTESIAN_POINT('Ctrl Pts',(0.878094004441076,-6.9561063070789,4.76643650867401));
#76005=CARTESIAN_POINT('Ctrl Pts',(0.849375472554175,-6.95967134686522,
4.76512227739976));
#76006=CARTESIAN_POINT('Ctrl Pts',(0.820636730396319,-6.96305837396359,
4.76380804612552));
#76007=CARTESIAN_POINT('Ctrl Pts',(0.634088041024268,-6.9850442167189,4.75527711876636));
#76008=CARTESIAN_POINT('Ctrl Pts',(0.446623371803321,-6.99953271404231,
4.7467461914072));
#76009=CARTESIAN_POINT('Ctrl Pts',(0.258857652594177,-7.00646981569131,
4.73821526404804));
#76010=CARTESIAN_POINT('Ctrl Pts',(0.0711275804650675,-7.0134056003405,
4.72968595627446));
#76011=CARTESIAN_POINT('Ctrl Pts',(-0.116903121735255,-7.01279283896199,
4.72115664850088));
#76012=CARTESIAN_POINT('Ctrl Pts',(-0.304617106574892,-7.00462953916065,
4.7126273407273));
#76013=CARTESIAN_POINT('Ctrl Pts',(-0.50198018779514,-6.99604661976286,
4.70365959938236));
#76014=CARTESIAN_POINT('Ctrl Pts',(-0.698992770735132,-6.97911647346224,
4.69469185803742));
#76015=CARTESIAN_POINT('Ctrl Pts',(-0.894939586002808,-6.95389888479155,
4.68572411669248));
#76016=CARTESIAN_POINT('Ctrl Pts',(-1.08130052324056,-6.92991496112774,
4.67719508456881));
#76017=CARTESIAN_POINT('Ctrl Pts',(-1.26669714843785,-6.8984351143025,4.66866605244514));
#76018=CARTESIAN_POINT('Ctrl Pts',(-1.45052084731942,-6.85956382243009,
4.66013702032147));
#76019=CARTESIAN_POINT('Ctrl Pts',(-1.6343463849235,-6.8206921417421,4.65160790288495));
#76020=CARTESIAN_POINT('Ctrl Pts',(-1.8165986658713,-6.77442893479044,4.64307878544843));
#76021=CARTESIAN_POINT('Ctrl Pts',(-1.99668021412985,-6.72092959976538,
4.63454966801191));
#76022=CARTESIAN_POINT('Ctrl Pts',(-2.17679819970371,-6.66741943979929,
4.62601882481201));
#76023=CARTESIAN_POINT('Ctrl Pts',(-2.35474428206376,-6.60667031551898,
4.61748798161212));
#76024=CARTESIAN_POINT('Ctrl Pts',(-2.52993621871967,-6.53888746590048,
4.60895713841222));
#76025=CARTESIAN_POINT('Ctrl Pts',(-2.55692566358928,-6.5284450818627,4.60764290713748));
#76026=CARTESIAN_POINT('Ctrl Pts',(-2.58384977831466,-6.51783585807876,
4.60632867586275));
#76027=CARTESIAN_POINT('Ctrl Pts',(-2.61070647377527,-6.50706064750344,
4.60501444458801));
#76028=CARTESIAN_POINT('Ctrl Pts',(-2.78503843687542,-6.43711668827108,
4.59648351722844));
#76029=CARTESIAN_POINT('Ctrl Pts',(-2.95658779836757,-6.36015088199461,
4.58795258986888));
#76030=CARTESIAN_POINT('Ctrl Pts',(-3.12478871300473,-6.27640996602184,
4.57942166250931));
#76031=CARTESIAN_POINT('Ctrl Pts',(-3.2929576949143,-6.19268494815441,4.57089235473535));
#76032=CARTESIAN_POINT('Ctrl Pts',(-3.45777922458243,-6.10218752384071,
4.56236304696138));
#76033=CARTESIAN_POINT('Ctrl Pts',(-3.61871023981373,-6.00521130042626,
4.55383373918742));
#76034=CARTESIAN_POINT('Ctrl Pts',(-3.78791362151685,-5.90325019042556,
4.54486599784267));
#76035=CARTESIAN_POINT('Ctrl Pts',(-3.95281566599222,-5.79412685004191,
4.53589825649793));
#76036=CARTESIAN_POINT('Ctrl Pts',(-4.1128168790768,-5.67823598326813,4.52693051515319));
#76037=CARTESIAN_POINT('Ctrl Pts',(-4.26499070232032,-5.56801459221749,
4.51840148302911));
#76038=CARTESIAN_POINT('Ctrl Pts',(-4.41273147077478,-5.45167218924061,
4.50987245090504));
#76039=CARTESIAN_POINT('Ctrl Pts',(-4.55555472963901,-5.32959169803501,
4.50134341878097));
#76040=CARTESIAN_POINT('Ctrl Pts',(-4.69837941711351,-5.20750998570166,
4.49281430134402));
#76041=CARTESIAN_POINT('Ctrl Pts',(-4.83628626606072,-5.07969027186573,
4.48428518390708));
#76042=CARTESIAN_POINT('Ctrl Pts',(-4.96882496410373,-4.94655486562108,
4.47575606647013));
#76043=CARTESIAN_POINT('Ctrl Pts',(-5.10139047974261,-4.8133925210439,4.46722522326986));
#76044=CARTESIAN_POINT('Ctrl Pts',(-5.22858545966915,-4.67491255349351,
4.45869438006958));
#76045=CARTESIAN_POINT('Ctrl Pts',(-5.34999681375759,-4.53157375039661,
4.45016353686931));
#76046=CARTESIAN_POINT('Ctrl Pts',(-5.36870101388029,-4.50949148569738,
4.44884930559637));
#76047=CARTESIAN_POINT('Ctrl Pts',(-5.38726802491544,-4.48729397047657,
4.44753507432342));
#76048=CARTESIAN_POINT('Ctrl Pts',(-5.40569642042982,-4.46498295323199,
4.44622084305048));
#76049=CARTESIAN_POINT('Ctrl Pts',(-5.52531867163167,-4.32015785940772,
4.43768991569185));
#76050=CARTESIAN_POINT('Ctrl Pts',(-5.63913799204207,-4.17049797480983,
4.42915898833322));
#76051=CARTESIAN_POINT('Ctrl Pts',(-5.7467755444098,-4.01649068275696,4.42062806097458));
#76052=CARTESIAN_POINT('Ctrl Pts',(-5.85439266192656,-3.86251262879054,
4.41209875320155));
#76053=CARTESIAN_POINT('Ctrl Pts',(-5.95583017811012,-3.70418906531192,
4.40356944542851));
#76054=CARTESIAN_POINT('Ctrl Pts',(-6.05075168607111,-3.54203763334153,
4.39504013765547));
#76055=CARTESIAN_POINT('Ctrl Pts',(-6.1505524617193,-3.37155110156666,4.38607239631026));
#76056=CARTESIAN_POINT('Ctrl Pts',(-6.24314950152146,-3.19683311190102,
4.37710465496506));
#76057=CARTESIAN_POINT('Ctrl Pts',(-6.32820521176558,-3.01851707967388,
4.36813691361985));
#76058=CARTESIAN_POINT('Ctrl Pts',(-6.40909992728024,-2.84892441320487,
4.3596078814967));
#76059=CARTESIAN_POINT('Ctrl Pts',(-6.48317339141903,-2.67607762759124,
4.35107884937354));
#76060=CARTESIAN_POINT('Ctrl Pts',(-6.55018339351676,-2.50054475540777,
4.34254981725039));
#76061=CARTESIAN_POINT('Ctrl Pts',(-6.61719406589158,-2.32501012743174,
4.33402069981438));
#76062=CARTESIAN_POINT('Ctrl Pts',(-6.67714102886938,-2.14678964641539,
4.32549158237837));
#76063=CARTESIAN_POINT('Ctrl Pts',(-6.72983089625954,-1.96646959555711,
4.31696246494236));
#76064=CARTESIAN_POINT('Ctrl Pts',(-6.78253142480478,-1.78611305912537,
4.30843162174297));
#76065=CARTESIAN_POINT('Ctrl Pts',(-6.82797183996164,-1.60365639853373,
4.29990077854357));
#76066=CARTESIAN_POINT('Ctrl Pts',(-6.86600889366736,-1.41970012135687,
4.29136993534418));
#76067=CARTESIAN_POINT('Ctrl Pts',(-6.87186874649775,-1.39136047339615,
4.29005570406711));
#76068=CARTESIAN_POINT('Ctrl Pts',(-6.87755299079739,-1.36298525616782,
4.28874147279004));
#76069=CARTESIAN_POINT('Ctrl Pts',(-6.88306121050991,-1.33457668752077,
4.28742724151297));
#76070=CARTESIAN_POINT('Ctrl Pts',(-6.91978280158916,-1.14518557833293,
4.2786656695244));
#76071=CARTESIAN_POINT('Ctrl Pts',(-6.94868659776524,-0.954261181418948,
4.26990409753583));
#76072=CARTESIAN_POINT('Ctrl Pts',(-6.96967016874586,-0.762446261315601,
4.26114252554726));
#76073=CARTESIAN_POINT('Ctrl Pts',(-6.99064763812959,-0.570687117100848,
4.25238350124613));
#76074=CARTESIAN_POINT('Ctrl Pts',(-7.00370945223445,-0.37803823423764,
4.24362447694499));
#76075=CARTESIAN_POINT('Ctrl Pts',(-7.00880493496689,-0.185148443374064,
4.23486545264386));
#76076=CARTESIAN_POINT('Ctrl Pts',(-7.0104337725736,-0.123488702421782,
4.23206551612579));
#76077=CARTESIAN_POINT('Ctrl Pts',(-7.01124897190917,-0.0618043785464321,
4.22926557960772));
#76078=CARTESIAN_POINT('Ctrl Pts',(-7.01124999902813,-0.000116739559371617,
4.22646564308964));
#76079=CARTESIAN_POINT('Ctrl Pts',(-7.01077745316898,-0.000116731691330088,
4.22646564308964));
#76080=CARTESIAN_POINT('Ctrl Pts',(-7.01035168527277,0.718306532755159,
4.19385497538491));
#76081=CARTESIAN_POINT('Ctrl Pts',(-6.88322317671624,1.55002980981697,4.15610807856266));
#76082=CARTESIAN_POINT('Ctrl Pts',(-6.6121722290669,2.33607121355468,4.11836118174041));
#76083=CARTESIAN_POINT('Ctrl Pts',(-6.57269630323124,2.4420685397187,4.11322495262288));
#76084=CARTESIAN_POINT('',(-7.01124999890438,0.000123949001866673,4.77353435691037));
#76085=CARTESIAN_POINT('Ctrl Pts',(-6.57226799596304,2.44190907933527,4.66030144016832));
#76086=CARTESIAN_POINT('Ctrl Pts',(-6.63771043057231,2.26577425834615,4.66883072547144));
#76087=CARTESIAN_POINT('Ctrl Pts',(-6.69607048136911,2.08700116691844,4.67736001077457));
#76088=CARTESIAN_POINT('Ctrl Pts',(-6.74715618316126,1.90617680253662,4.68588929607769));
#76089=CARTESIAN_POINT('Ctrl Pts',(-6.79824010009948,1.7253587558732,4.69441828338103));
#76090=CARTESIAN_POINT('Ctrl Pts',(-6.84205009466234,1.54248987476095,4.70294727068437));
#76091=CARTESIAN_POINT('Ctrl Pts',(-6.87844442865365,1.35817112486742,4.7114762579877));
#76092=CARTESIAN_POINT('Ctrl Pts',(-6.91484744362043,1.17380841025816,4.72000727967171));
#76093=CARTESIAN_POINT('Ctrl Pts',(-6.94383120347836,0.987995436261786,
4.72853830135572));
#76094=CARTESIAN_POINT('Ctrl Pts',(-6.96530514058173,0.801343160628309,
4.73706932303973));
#76095=CARTESIAN_POINT('Ctrl Pts',(-6.98103312913002,0.664634887732377,
4.74331763282593));
#76096=CARTESIAN_POINT('Ctrl Pts',(-6.99273359566149,0.52747659570593,4.74956594261214));
#76097=CARTESIAN_POINT('Ctrl Pts',(-7.00038860523991,0.390110161527862,
4.75581425239835));
#76098=CARTESIAN_POINT('Ctrl Pts',(-7.00762509928983,0.260253840199072,
4.76172095390235));
#76099=CARTESIAN_POINT('Ctrl Pts',(-7.01124769942693,0.130195277014969,
4.76762765540636));
#76100=CARTESIAN_POINT('Ctrl Pts',(-7.01124999890438,0.000123949001866673,
4.77353435691037));
#76101=CARTESIAN_POINT('Ctrl Pts',(-7.01124999909022,0.000112948703611393,
4.77329468133506));
#76102=CARTESIAN_POINT('Ctrl Pts',(-7.01125679909962,-0.421995179608593,
4.79266801673904));
#76103=CARTESIAN_POINT('Ctrl Pts',(-6.97314410821326,-0.8432534060986,4.81213169562656));
#76104=CARTESIAN_POINT('Ctrl Pts',(-6.88164419495031,-1.34472218830463,
4.83531049418384));
#76105=CARTESIAN_POINT('Ctrl Pts',(-6.86430093479642,-1.43062134470753,
4.83928390680739));
#76106=CARTESIAN_POINT('Ctrl Pts',(-6.75240376876267,-1.93582448205209,
4.86268916910286));
#76107=CARTESIAN_POINT('Ctrl Pts',(-6.62106364394987,-2.34603645146997,
4.88177993626495));
#76108=CARTESIAN_POINT('Ctrl Pts',(-6.41003474131369,-2.84273608613219,
4.9060725872766));
#76109=CARTESIAN_POINT('Ctrl Pts',(-6.3647098019935,-2.94281543766909,4.91103505537233));
#76110=CARTESIAN_POINT('Ctrl Pts',(-6.20739139014251,-3.26952732963385,
4.92752792430019));
#76111=CARTESIAN_POINT('Ctrl Pts',(-6.08549654383899,-3.49116688776528,
4.9391679889615));
#76112=CARTESIAN_POINT('Ctrl Pts',(-5.78797482262491,-3.96902597464448,
4.96506755660791));
#76113=CARTESIAN_POINT('Ctrl Pts',(-5.6067552475093,-4.22115166241315,4.97928627065715));
#76114=CARTESIAN_POINT('Ctrl Pts',(-5.15084960484008,-4.7740536520115,5.01182502581467));
#76115=CARTESIAN_POINT('Ctrl Pts',(-4.86548153778363,-5.06457642353853,
5.02996494644311));
#76116=CARTESIAN_POINT('Ctrl Pts',(-4.41388272609466,-5.45073422911981,
5.05660352002761));
#76117=CARTESIAN_POINT('Ctrl Pts',(-4.26637231559178,-5.56694978148892,
5.06503526396739));
#76118=CARTESIAN_POINT('Ctrl Pts',(-3.90823318420276,-5.82650464906067,
5.08513167971144));
#76119=CARTESIAN_POINT('Ctrl Pts',(-3.69410520199835,-5.96456428372902,
5.09685270424898));
#76120=CARTESIAN_POINT('Ctrl Pts',(-3.21358206001639,-6.23856225368875,
5.12230448629601));
#76121=CARTESIAN_POINT('Ctrl Pts',(-2.94503149337547,-6.36973808840384,
5.13600165082681));
#76122=CARTESIAN_POINT('Ctrl Pts',(-2.44196155883025,-6.57683034191199,
5.16073197124822));
#76123=CARTESIAN_POINT('Ctrl Pts',(-2.2102359956425,-6.65828306934746,5.17179214836363));
#76124=CARTESIAN_POINT('Ctrl Pts',(-1.75342406793481,-6.79237212488537,
5.19315794123468));
#76125=CARTESIAN_POINT('Ctrl Pts',(-1.5290646716379,-6.84636953226539,5.20345684828559));
#76126=CARTESIAN_POINT('Ctrl Pts',(-1.15368175683848,-6.91733830065786,
5.22061732016552));
#76127=CARTESIAN_POINT('Ctrl Pts',(-1.00404072754944,-6.94063774890685,
5.22744235307077));
#76128=CARTESIAN_POINT('Ctrl Pts',(-0.608744709303136,-6.9891339614576,
5.24556671140942));
#76129=CARTESIAN_POINT('Ctrl Pts',(-0.36231299776361,-7.0062322788189,5.25693394089039));
#76130=CARTESIAN_POINT('Ctrl Pts',(0.191738457234614,-7.01536042568755,
5.28242948160838));
#76131=CARTESIAN_POINT('Ctrl Pts',(0.498978774929529,-7.00021939269596,
5.29651798161029));
#76132=CARTESIAN_POINT('Ctrl Pts',(1.22071726182776,-6.91688113884293,5.32951377679443));
#76133=CARTESIAN_POINT('Ctrl Pts',(1.6320460236115,-6.83153174664252,5.34821330112677));
#76134=CARTESIAN_POINT('Ctrl Pts',(2.1580545733809,-6.67213793202217,5.37286078239703));
#76135=CARTESIAN_POINT('Ctrl Pts',(2.28174665464909,-6.63085633682415,5.37871746682301));
#76136=CARTESIAN_POINT('Ctrl Pts',(2.52624737793925,-6.54160356431424,5.39048317998939));
#76137=CARTESIAN_POINT('Ctrl Pts',(2.64701557281996,-6.493674639887,5.39639814990493));
#76138=CARTESIAN_POINT('Ctrl Pts',(3.02401957130557,-6.33178876439205,5.4151804945424));
#76139=CARTESIAN_POINT('Ctrl Pts',(3.27478963052073,-6.20580343161588,5.42811728053557));
#76140=CARTESIAN_POINT('Ctrl Pts',(3.68829303968288,-5.96600154655731,5.45006060240372));
#76141=CARTESIAN_POINT('Ctrl Pts',(3.85497915505517,-5.85967724610324,5.4590932145682));
#76142=CARTESIAN_POINT('Ctrl Pts',(4.3829150375993,-5.49063334076114,5.48836234204885));
#76143=CARTESIAN_POINT('Ctrl Pts',(4.72360355932173,-5.20043964978641,5.5082534046618));
#76144=CARTESIAN_POINT('Ctrl Pts',(5.15033679390985,-4.76019070077597,5.53576602263396));
#76145=CARTESIAN_POINT('Ctrl Pts',(5.26199334869462,-4.63646520330071,5.54326332769117));
#76146=CARTESIAN_POINT('Ctrl Pts',(5.5174107115067,-4.33231651263527,5.56132251036776));
#76147=CARTESIAN_POINT('Ctrl Pts',(5.65688475498112,-4.14854673141831,5.57192926731237));
#76148=CARTESIAN_POINT('Ctrl Pts',(5.9171127704807,-3.76808686898075,5.59313905822258));
#76149=CARTESIAN_POINT('Ctrl Pts',(6.03772568284979,-3.57163444464497,5.60372898481114));
#76150=CARTESIAN_POINT('Ctrl Pts',(6.19654863945421,-3.28183305172802,5.61882606002129));
#76151=CARTESIAN_POINT('Ctrl Pts',(6.24276404825244,-3.19304564660264,5.62338513109736));
#76152=CARTESIAN_POINT('Ctrl Pts',(6.47405621673876,-2.72446413139617,5.64711856109728));
#76153=CARTESIAN_POINT('Ctrl Pts',(6.62642664102905,-2.32950285230411,5.6659591119782));
#76154=CARTESIAN_POINT('Ctrl Pts',(6.79130883108704,-1.75147155130558,5.69291614749831));
#76155=CARTESIAN_POINT('Ctrl Pts',(6.8337210897994,-1.57790458700881,5.70094476091029));
#76156=CARTESIAN_POINT('Ctrl Pts',(6.91857734053677,-1.16239933069317,5.72021849451929));
#76157=CARTESIAN_POINT('Ctrl Pts',(6.95503008523638,-0.919477357552379,
5.73151644756159));
#76158=CARTESIAN_POINT('Ctrl Pts',(7.00029356200322,-0.451611455313158,
5.75314509896803));
#76159=CARTESIAN_POINT('Ctrl Pts',(7.01116692644202,-0.227162863482876,
5.76346453614652));
#76160=CARTESIAN_POINT('Ctrl Pts',(7.01128632737948,0.0974833021738531,
5.77829163797521));
#76161=CARTESIAN_POINT('Ctrl Pts',(7.00918105544768,0.197535147302001,5.78284839017917));
#76162=CARTESIAN_POINT('Ctrl Pts',(6.98775276409793,0.702071791296174,5.80577727127322));
#76163=CARTESIAN_POINT('Ctrl Pts',(6.93555523761715,1.10438764393122,5.82384990722907));
#76164=CARTESIAN_POINT('Ctrl Pts',(6.80856887317956,1.68422154293215,5.85046025067915));
#76165=CARTESIAN_POINT('Ctrl Pts',(6.76079180215199,1.86678995278535,5.8589329155193));
#76166=CARTESIAN_POINT('Ctrl Pts',(6.63113405065837,2.29148941048707,5.87910821630758));
#76167=CARTESIAN_POINT('Ctrl Pts',(6.54326422017995,2.53151202546576,5.89086742973181));
#76168=CARTESIAN_POINT('Ctrl Pts',(6.32486766552816,3.04015866555996,5.91633746879359));
#76169=CARTESIAN_POINT('Ctrl Pts',(6.1898827228241,3.30633826493007,5.93001483632165));
#76170=CARTESIAN_POINT('Ctrl Pts',(5.91352839167062,3.77467177635828,5.95473407009145));
#76171=CARTESIAN_POINT('Ctrl Pts',(5.77766201619294,3.97952128726904,5.96580241558632));
#76172=CARTESIAN_POINT('Ctrl Pts',(5.43098270746449,4.44692559060206,5.99191841812494));
#76173=CARTESIAN_POINT('Ctrl Pts',(5.21147100502431,4.70226371963072,6.0068840772248));
#76174=CARTESIAN_POINT('Ctrl Pts',(4.8754280415691,5.0405940508303,6.02847610270383));
#76175=CARTESIAN_POINT('Ctrl Pts',(4.77339167016613,5.13732589108303,6.03489417321059));
#76176=CARTESIAN_POINT('Ctrl Pts',(4.47046904835554,5.40767968635405,6.05351321583316));
#76177=CARTESIAN_POINT('Ctrl Pts',(4.26254070274911,5.57304587974599,6.06575605996636));
#76178=CARTESIAN_POINT('Ctrl Pts',(3.88452279988924,5.84012612300974,6.08699336517462));
#76179=CARTESIAN_POINT('Ctrl Pts',(3.71856830581541,5.9471709255966,6.09600876968458));
#76180=CARTESIAN_POINT('Ctrl Pts',(3.19889281292691,6.25210750204974,6.1233666735894));
#76181=CARTESIAN_POINT('Ctrl Pts',(2.83235371138637,6.42647188805495,6.14144849944093));
#76182=CARTESIAN_POINT('Ctrl Pts',(2.27620785654595,6.63415723920077,6.16806267351317));
#76183=CARTESIAN_POINT('Ctrl Pts',(2.09701923295155,6.69295697248118,6.1765297257224));
#76184=CARTESIAN_POINT('Ctrl Pts',(1.67009496807675,6.81421956123695,6.19669425328008));
#76185=CARTESIAN_POINT('Ctrl Pts',(1.42088376594601,6.87050886259863,6.20844827668929));
#76186=CARTESIAN_POINT('Ctrl Pts',(0.875137031947884,6.96280728062533,6.23391583473576));
#76187=CARTESIAN_POINT('Ctrl Pts',(0.578234595829499,6.99372575616231,6.24759589254961));
#76188=CARTESIAN_POINT('Ctrl Pts',(0.0348466737759841,7.01546422384793,
6.27231662754573));
#76189=CARTESIAN_POINT('Ctrl Pts',(-0.210919380432283,7.01237966542289,
6.28338385771086));
#76190=CARTESIAN_POINT('Ctrl Pts',(-0.68490445812741,6.98148577307377,6.30470031306995));
#76191=CARTESIAN_POINT('Ctrl Pts',(-0.912919308510342,6.95534438888378,
6.31494352266387));
#76192=CARTESIAN_POINT('Ctrl Pts',(-1.28919125067015,6.89338140761715,6.33207208481146));
#76193=CARTESIAN_POINT('Ctrl Pts',(-1.43829576788489,6.8638200709508,6.33892195019952));
#76194=CARTESIAN_POINT('Ctrl Pts',(-1.82833172178249,6.77322360981884,6.35714387876324));
#76195=CARTESIAN_POINT('Ctrl Pts',(-2.06717972324997,6.70418680535927,6.36858525574703));
#76196=CARTESIAN_POINT('Ctrl Pts',(-2.59423413122072,6.52099594917694,6.39425799756116));
#76197=CARTESIAN_POINT('Ctrl Pts',(-2.87956637883259,6.40012049589865,6.40844827520084));
#76198=CARTESIAN_POINT('Ctrl Pts',(-3.51914294893291,6.07771839486986,6.44096974458012));
#76199=CARTESIAN_POINT('Ctrl Pts',(-3.86569120837204,5.86340041979019,6.4591197941867));
#76200=CARTESIAN_POINT('Ctrl Pts',(-4.34206960367874,5.50810711352361,6.48576265428615));
#76201=CARTESIAN_POINT('Ctrl Pts',(-4.48787096327097,5.38997447936336,6.4941882725242));
#76202=CARTESIAN_POINT('Ctrl Pts',(-4.8198869149895,5.09814375303654,6.51427281140552));
#76203=CARTESIAN_POINT('Ctrl Pts',(-5.0017265330871,4.919868756499,6.52598804908439));
#76204=CARTESIAN_POINT('Ctrl Pts',(-5.37502510657105,4.5117526659675,6.55143706435205));
#76205=CARTESIAN_POINT('Ctrl Pts',(-5.5622990345381,4.27874299650751,6.56513722909619));
#76206=CARTESIAN_POINT('Ctrl Pts',(-5.87537128270766,3.8337803959583,6.58986923763532));
#76207=CARTESIAN_POINT('Ctrl Pts',(-6.0059615065987,3.62578118502098,6.60092818467359));
#76208=CARTESIAN_POINT('Ctrl Pts',(-6.23777964980658,3.20953274361292,6.62231029130177));
#76209=CARTESIAN_POINT('Ctrl Pts',(-6.34013794114365,3.00227343359751,6.63262653190011));
#76210=CARTESIAN_POINT('Ctrl Pts',(-6.48191316875309,2.67546416034317,6.64862854258803));
#76211=CARTESIAN_POINT('Ctrl Pts',(-6.52865946284866,2.55927911941613,6.65426924392862));
#76212=CARTESIAN_POINT('Ctrl Pts',(-6.57226799589878,2.4419090795082,6.65995074817407));
#76213=CARTESIAN_POINT('Origin',(0.,0.,10.));
#76214=CARTESIAN_POINT('',(-6.57226798695174,2.4419091035887,8.66059774113391));
#76215=CARTESIAN_POINT('',(-6.57226800401825,2.44190905765509,8.11350492783088));
#76216=CARTESIAN_POINT('',(-6.57226799596304,2.44190907933527,10.));
#76217=CARTESIAN_POINT('',(-7.01124999771048,0.000179177963096134,6.22646564308964));
#76218=CARTESIAN_POINT('Ctrl Pts',(-6.57226800401825,2.44190905765509,8.11350492783088));
#76219=CARTESIAN_POINT('Ctrl Pts',(-6.55743799171866,2.48182324488917,8.11158964032659));
#76220=CARTESIAN_POINT('Ctrl Pts',(-6.5422430036516,2.52160602315529,8.10967167924349));
#76221=CARTESIAN_POINT('Ctrl Pts',(-6.4803660331804,2.67928337028087,8.10202931630123));
#76222=CARTESIAN_POINT('Ctrl Pts',(-6.43085534038898,2.79603327768028,8.0962737171796));
#76223=CARTESIAN_POINT('Ctrl Pts',(-6.2501010499617,3.1920274850446,8.07638364749166));
#76224=CARTESIAN_POINT('Ctrl Pts',(-6.10361224707174,3.46391684443965,8.06214069269033));
#76225=CARTESIAN_POINT('Ctrl Pts',(-5.81073924316456,3.93088299834635,8.03684019739495));
#76226=CARTESIAN_POINT('Ctrl Pts',(-5.67119309610008,4.12966147061864,8.02576427414835));
#76227=CARTESIAN_POINT('Ctrl Pts',(-5.45957965384424,4.40008531075991,8.01020713756199));
#76228=CARTESIAN_POINT('Ctrl Pts',(-5.39584023614814,4.47802066956506,8.00566073656017));
#76229=CARTESIAN_POINT('Ctrl Pts',(-5.17382484179504,4.73785729996587,7.9902641067623));
#76230=CARTESIAN_POINT('Ctrl Pts',(-5.00785430304868,4.91295751313342,7.97948278038044));
#76231=CARTESIAN_POINT('Ctrl Pts',(-4.68900500442983,5.21636601734565,7.95976237792332));
#76232=CARTESIAN_POINT('Ctrl Pts',(-4.53904117168727,5.34736809059905,7.95083737907751));
#76233=CARTESIAN_POINT('Ctrl Pts',(-4.25854004546789,5.57208997865151,7.93453846180782));
#76234=CARTESIAN_POINT('Ctrl Pts',(-4.12996819005442,5.66804295151848,7.92719677564156));
#76235=CARTESIAN_POINT('Ctrl Pts',(-3.6324499729222,6.01341807435682,7.8993789797547));
#76236=CARTESIAN_POINT('Ctrl Pts',(-3.24331000222098,6.2319215416855,7.87887419765568));
#76237=CARTESIAN_POINT('Ctrl Pts',(-2.55366060353697,6.53695715410225,7.84466811319653));
#76238=CARTESIAN_POINT('Ctrl Pts',(-2.26329460062408,6.64307857538963,7.83082448585817));
#76239=CARTESIAN_POINT('Ctrl Pts',(-1.72998530629469,6.79894760719639,7.8059372115454));
#76240=CARTESIAN_POINT('Ctrl Pts',(-1.48960655813323,6.8556259112,7.79490207189863));
#76241=CARTESIAN_POINT('Ctrl Pts',(-1.09776743482913,6.92643141625173,7.77685522302357));
#76242=CARTESIAN_POINT('Ctrl Pts',(-0.947960251614167,6.94851891099159,
7.76993219269087));
#76243=CARTESIAN_POINT('Ctrl Pts',(-0.568394476943045,6.99197819336942,
7.75239508717265));
#76244=CARTESIAN_POINT('Ctrl Pts',(-0.338074809094541,7.00689211214926,
7.74176312764431));
#76245=CARTESIAN_POINT('Ctrl Pts',(0.137981144539973,7.01418799745145,7.71990514651528));
#76246=CARTESIAN_POINT('Ctrl Pts',(0.383433248609888,7.00505919989913,7.70870081730449));
#76247=CARTESIAN_POINT('Ctrl Pts',(0.925277745823956,6.9563376951143,7.68404864538288));
#76248=CARTESIAN_POINT('Ctrl Pts',(1.22064235856468,6.91063012757235,7.67066995300729));
#76249=CARTESIAN_POINT('Ctrl Pts',(1.76078477099419,6.79132354169578,7.64589328183402));
#76250=CARTESIAN_POINT('Ctrl Pts',(2.00619572181711,6.72291700716577,7.6345083647682));
#76251=CARTESIAN_POINT('Ctrl Pts',(2.425141450439,6.58115109824151,7.61443049309929));
#76252=CARTESIAN_POINT('Ctrl Pts',(2.60045505571314,6.51386922787786,7.60581926436072));
#76253=CARTESIAN_POINT('Ctrl Pts',(3.1461899633329,6.27888022055778,7.57849719911343));
#76254=CARTESIAN_POINT('Ctrl Pts',(3.50484782594696,6.08595945740171,7.55980860075223));
#76255=CARTESIAN_POINT('Ctrl Pts',(4.10429799392953,5.6928625669429,7.52728829737601));
#76256=CARTESIAN_POINT('Ctrl Pts',(4.35224237910438,5.50562772812465,7.51337495393488));
#76257=CARTESIAN_POINT('Ctrl Pts',(4.77412475970954,5.1406807790236,7.48838878419116));
#76258=CARTESIAN_POINT('Ctrl Pts',(4.95257714444692,4.96898805618932,7.47732426678287));
#76259=CARTESIAN_POINT('Ctrl Pts',(5.22512418692035,4.67746654960826,7.45923645188895));
#76260=CARTESIAN_POINT('Ctrl Pts',(5.32505063162602,4.5633814271053,7.45230257026397));
#76261=CARTESIAN_POINT('Ctrl Pts',(5.56718418754557,4.26814753012032,7.43477520138407));
#76262=CARTESIAN_POINT('Ctrl Pts',(5.70431522031333,4.08306395911104,7.42416415263037));
#76263=CARTESIAN_POINT('Ctrl Pts',(5.9683466003706,3.68737396183035,7.40232538388935));
#76264=CARTESIAN_POINT('Ctrl Pts',(6.09378402112142,3.47615988872294,7.39111954873523));
#76265=CARTESIAN_POINT('Ctrl Pts',(6.34662788481562,2.9945022179251,7.36646920714207));
#76266=CARTESIAN_POINT('Ctrl Pts',(6.4683505287011,2.72161238445936,7.35309374409657));
#76267=CARTESIAN_POINT('Ctrl Pts',(6.66102318643904,2.20301642554055,7.32831396595407));
#76268=CARTESIAN_POINT('Ctrl Pts',(6.73665588446388,1.95958532626026,7.31692273169131));
#76269=CARTESIAN_POINT('Ctrl Pts',(6.84476244024639,1.53040771121768,7.29683105917654));
#76270=CARTESIAN_POINT('Ctrl Pts',(6.88330997576356,1.34646291639651,7.28821243578745));
#76271=CARTESIAN_POINT('Ctrl Pts',(6.98169930849974,0.760596471026311,7.26089514120011));
#76272=CARTESIAN_POINT('Ctrl Pts',(7.01403534692144,0.354898640283086,7.24221888701904));
#76273=CARTESIAN_POINT('Ctrl Pts',(7.0103298676516,-0.151373695439597,7.21925066148355));
#76274=CARTESIAN_POINT('Ctrl Pts',(7.00745561476455,-0.251405832416107,
7.21472571493635));
#76275=CARTESIAN_POINT('Ctrl Pts',(6.99672086768851,-0.465354874216318,
7.20506380305275));
#76276=CARTESIAN_POINT('Ctrl Pts',(6.98821673433173,-0.579210838011116,
7.1999319245512));
#76277=CARTESIAN_POINT('Ctrl Pts',(6.95009629580528,-0.963102972505531,
7.18262007458876));
#76278=CARTESIAN_POINT('Ctrl Pts',(6.90757179907468,-1.23160704678244,7.17050530862667));
#76279=CARTESIAN_POINT('Ctrl Pts',(6.82156504401769,-1.62514358855543,7.15236410297419));
#76280=CARTESIAN_POINT('Ctrl Pts',(6.78995984234394,-1.752508536021,7.1464257570538));
#76281=CARTESIAN_POINT('Ctrl Pts',(6.72057170037631,-2.00196290508527,7.13461531624808));
#76282=CARTESIAN_POINT('Ctrl Pts',(6.68298837135976,-2.12405399667506,7.12875634265293));
#76283=CARTESIAN_POINT('Ctrl Pts',(6.50651377443913,-2.64616301204923,7.10342390529694));
#76284=CARTESIAN_POINT('Ctrl Pts',(6.33487610871482,-3.03418177473879,7.08394471886494));
#76285=CARTESIAN_POINT('Ctrl Pts',(5.98020890095359,-3.67273545297891,7.05081139597953));
#76286=CARTESIAN_POINT('Ctrl Pts',(5.81366792564436,-3.93104992642798,7.0370469422111));
#76287=CARTESIAN_POINT('Ctrl Pts',(5.48211435815663,-4.37792873893386,7.01212261396588));
#76288=CARTESIAN_POINT('Ctrl Pts',(5.32291652827791,-4.57016345622703,7.00097162699666));
#76289=CARTESIAN_POINT('Ctrl Pts',(5.05055109649184,-4.86546605050667,6.98276295231262));
#76290=CARTESIAN_POINT('Ctrl Pts',(4.94366555649898,-4.97403209793866,6.97579686226693));
#76291=CARTESIAN_POINT('Ctrl Pts',(4.48971091255839,-5.40602676156326,6.9470295041862));
#76292=CARTESIAN_POINT('Ctrl Pts',(4.11378047428365,-5.69732039118457,6.92517891382745));
#76293=CARTESIAN_POINT('Ctrl Pts',(3.45902305259344,-6.10583499038029,6.89020694535978));
#76294=CARTESIAN_POINT('Ctrl Pts',(3.19696155546038,-6.24703943541135,6.87688058968884));
#76295=CARTESIAN_POINT('Ctrl Pts',(2.69327891564335,-6.47841586711455,6.85205354450293));
#76296=CARTESIAN_POINT('Ctrl Pts',(2.45411924910366,-6.57274052199594,6.84056625555677));
#76297=CARTESIAN_POINT('Ctrl Pts',(2.02967220752053,-6.71373930813828,6.82026128866536));
#76298=CARTESIAN_POINT('Ctrl Pts',(1.84664925498781,-6.76636898724402,6.81152672305988));
#76299=CARTESIAN_POINT('Ctrl Pts',(1.27106942842937,-6.90678617362863,6.78428161912001));
#76300=CARTESIAN_POINT('Ctrl Pts',(0.87294010245506,-6.96830686883063,6.76579619228501));
#76301=CARTESIAN_POINT('Ctrl Pts',(0.161859247530876,-7.01625876510001,
6.73346188776163));
#76302=CARTESIAN_POINT('Ctrl Pts',(-0.149063728130618,-7.01654257392534,
6.7195377353665));
#76303=CARTESIAN_POINT('Ctrl Pts',(-0.707083092720185,-6.97993401271807,
6.6944891229262));
#76304=CARTESIAN_POINT('Ctrl Pts',(-0.954138696093317,-6.9504720131852,
6.68337298133156));
#76305=CARTESIAN_POINT('Ctrl Pts',(-1.34889721563537,-6.88194866636739,
6.66521305977248));
#76306=CARTESIAN_POINT('Ctrl Pts',(-1.49780368827869,-6.8510819173672,6.65825999598243));
#76307=CARTESIAN_POINT('Ctrl Pts',(-1.86832894631033,-6.76161818534322,
6.6407621070194));
#76308=CARTESIAN_POINT('Ctrl Pts',(-2.08830171764772,-6.69694928891135,
6.63020036457347));
#76309=CARTESIAN_POINT('Ctrl Pts',(-2.53673320352266,-6.54086893825623,
6.60840144941294));
#76310=CARTESIAN_POINT('Ctrl Pts',(-2.76435195785374,-6.4479720427829,6.59718667471982));
#76311=CARTESIAN_POINT('Ctrl Pts',(-3.25629743072108,-6.2163491577006,6.57254707004008));
#76312=CARTESIAN_POINT('Ctrl Pts',(-3.51759857248614,-6.07231204571228,
6.55919065236748));
#76313=CARTESIAN_POINT('Ctrl Pts',(-3.98444287679584,-5.77469968391117,
6.53439254664884));
#76314=CARTESIAN_POINT('Ctrl Pts',(-4.19226868448282,-5.62563957349027,
6.52296405691939));
#76315=CARTESIAN_POINT('Ctrl Pts',(-4.53868033199722,-5.34730396741956,
6.50279043877826));
#76316=CARTESIAN_POINT('Ctrl Pts',(-4.68103265499013,-5.22314178804768,
6.49412764123343));
#76317=CARTESIAN_POINT('Ctrl Pts',(-5.11214575074516,-4.81532127200719,
6.46683842532445));
#76318=CARTESIAN_POINT('Ctrl Pts',(-5.3814778365187,-4.51232334275096,6.4482354747848));
#76319=CARTESIAN_POINT('Ctrl Pts',(-5.74107478481165,-4.02947288138569,
6.42092249097817));
#76320=CARTESIAN_POINT('Ctrl Pts',(-5.85224059235256,-3.86624792410868,
6.41202772809416));
#76321=CARTESIAN_POINT('Ctrl Pts',(-6.1352284528919,-3.4105067316652,6.38793998648474));
#76322=CARTESIAN_POINT('Ctrl Pts',(-6.29295321481477,-3.10987437749404,
6.37285457546544));
#76323=CARTESIAN_POINT('Ctrl Pts',(-6.48033931322618,-2.67951797885644,
6.35162781671172));
#76324=CARTESIAN_POINT('Ctrl Pts',(-6.529028545093,-2.55859320303073,6.34568988560134));
#76325=CARTESIAN_POINT('Ctrl Pts',(-6.73087075116901,-2.01394377636797,
6.31909105740829));
#76326=CARTESIAN_POINT('Ctrl Pts',(-6.84634643856867,-1.57738522833334,
6.29827911901619));
#76327=CARTESIAN_POINT('Ctrl Pts',(-6.94246099196424,-0.990304786190284,
6.27121013842236));
#76328=CARTESIAN_POINT('Ctrl Pts',(-6.9613798781732,-0.847147631325589,
6.26467194045431));
#76329=CARTESIAN_POINT('Ctrl Pts',(-6.99944632495622,-0.469686896284264,
6.24755607764817));
#76330=CARTESIAN_POINT('Ctrl Pts',(-7.0112560665116,-0.234827899798161,
6.23703396468846));
#76331=CARTESIAN_POINT('Ctrl Pts',(-7.01124999766219,0.000181057866101147,
6.2265076133824));
#76332=CARTESIAN_POINT('Ctrl Pts',(-7.01124999771049,0.000179177963096134,
6.22646564308964));
#76333=CARTESIAN_POINT('Ctrl Pts',(-7.01124490821585,0.199331566167948,
6.21742360468036));
#76334=CARTESIAN_POINT('Ctrl Pts',(-7.00275018852882,0.39844265281681,6.20838156627109));
#76335=CARTESIAN_POINT('Ctrl Pts',(-6.98580233730263,0.596818453666757,
6.19933952786181));
#76336=CARTESIAN_POINT('Ctrl Pts',(-6.98181057617832,0.643542300794496,
6.19720983856227));
#76337=CARTESIAN_POINT('Ctrl Pts',(-6.97735010198673,0.69022537353174,6.19508014926272));
#76338=CARTESIAN_POINT('Ctrl Pts',(-6.97242181091054,0.73685863857258,6.19295045996318));
#76339=CARTESIAN_POINT('Ctrl Pts',(-6.95268047751938,0.923658244776018,
6.1844195299041));
#76340=CARTESIAN_POINT('Ctrl Pts',(-6.92542456469802,1.1096960269454,6.17588859984501));
#76341=CARTESIAN_POINT('Ctrl Pts',(-6.89073711509391,1.29436029495933,6.16735766978593));
#76342=CARTESIAN_POINT('Ctrl Pts',(-6.85605668170207,1.47898721102849,6.1588284652736));
#76343=CARTESIAN_POINT('Ctrl Pts',(-6.81394776824682,1.66224086665267,6.15029926076127));
#76344=CARTESIAN_POINT('Ctrl Pts',(-6.76454471919494,1.84351872909168,6.14177005624894));
#76345=CARTESIAN_POINT('Ctrl Pts',(-6.71514635696827,2.02477939385422,6.13324166089499));
#76346=CARTESIAN_POINT('Ctrl Pts',(-6.65845532044975,2.20406434413078,6.12471326554103));
#76347=CARTESIAN_POINT('Ctrl Pts',(-6.59465630396905,2.38078449151143,6.11618487018707));
#76348=CARTESIAN_POINT('Ctrl Pts',(-6.58728817646199,2.40119384342299,6.11519992860232));
#76349=CARTESIAN_POINT('Ctrl Pts',(-6.57982529813203,2.42156900377658,6.11421498701756));
#76350=CARTESIAN_POINT('Ctrl Pts',(-6.57226799596304,2.44190907933527,6.1132300454328));
#76351=CARTESIAN_POINT('Ctrl Pts',(-6.57226799589878,2.4419090795082,6.65995074817407));
#76352=CARTESIAN_POINT('Ctrl Pts',(-6.58131771308462,2.41755224856329,6.66112978362918));
#76353=CARTESIAN_POINT('Ctrl Pts',(-6.59023229898885,2.39314438829913,6.66231065902376));
#76354=CARTESIAN_POINT('Ctrl Pts',(-6.68221482357477,2.13688688044955,6.67470135157294));
#76355=CARTESIAN_POINT('Ctrl Pts',(-6.75314634805076,1.90086630247217,6.68604193313713));
#76356=CARTESIAN_POINT('Ctrl Pts',(-6.88314653638676,1.36794965318498,6.71128068282838));
#76357=CARTESIAN_POINT('Ctrl Pts',(-6.93571747621243,1.06996312059661,6.72514149733374));
#76358=CARTESIAN_POINT('Ctrl Pts',(-6.99711562074584,0.513926255681263,
6.75055596579651));
#76359=CARTESIAN_POINT('Ctrl Pts',(-7.01125611619881,0.256978822438064,
6.76212942280701));
#76360=CARTESIAN_POINT('Ctrl Pts',(-7.011243385311,-0.278097192768184,6.78612673913558));
#76361=CARTESIAN_POINT('Ctrl Pts',(-6.99471080565663,-0.555778604460915,
6.79852182034323));
#76362=CARTESIAN_POINT('Ctrl Pts',(-6.94670341357092,-0.95760418852317,
6.81678288974097));
#76363=CARTESIAN_POINT('Ctrl Pts',(-6.92825614545814,-1.08303280228687,
6.82253801863334));
#76364=CARTESIAN_POINT('Ctrl Pts',(-6.88098492762266,-1.35331757087629,
6.8350771712644));
#76365=CARTESIAN_POINT('Ctrl Pts',(-6.8509641279571,-1.49790252529874,6.84186181752672));
#76366=CARTESIAN_POINT('Ctrl Pts',(-6.73191371868191,-1.99228551530236,
6.86525578795537));
#76367=CARTESIAN_POINT('Ctrl Pts',(-6.62046125839425,-2.33610047252772,
6.88183668462479));
#76368=CARTESIAN_POINT('Ctrl Pts',(-6.38270144433937,-2.91344748834885,
6.91019572887894));
#76369=CARTESIAN_POINT('Ctrl Pts',(-6.26871147363916,-3.15124004571073,
6.92204860411966));
#76370=CARTESIAN_POINT('Ctrl Pts',(-5.98440861800993,-3.66751690392067,
6.94847414748757));
#76371=CARTESIAN_POINT('Ctrl Pts',(-5.80750188670883,-3.94166734281123,
6.96298892029673));
#76372=CARTESIAN_POINT('Ctrl Pts',(-5.50457485250056,-4.34620613502314,
6.98592598315164));
#76373=CARTESIAN_POINT('Ctrl Pts',(-5.39149719422794,-4.48571154734406,
6.99415664389733));
#76374=CARTESIAN_POINT('Ctrl Pts',(-4.99586713817197,-4.93720677967955,
7.02175348051643));
#76375=CARTESIAN_POINT('Ctrl Pts',(-4.69060481405529,-5.22809140792073,
7.04110785646335));
#76376=CARTESIAN_POINT('Ctrl Pts',(-4.1191372564352,-5.68206207282254,7.07420965234174));
#76377=CARTESIAN_POINT('Ctrl Pts',(-3.86472648733112,-5.85807258089696,
7.0880609931667));
#76378=CARTESIAN_POINT('Ctrl Pts',(-3.37583837714098,-6.15055204011379,
7.11357863093797));
#76379=CARTESIAN_POINT('Ctrl Pts',(-3.14485841685916,-6.27179689551686,
7.12523247441315));
#76380=CARTESIAN_POINT('Ctrl Pts',(-2.73016450371685,-6.46079569246422,
7.14592460237187));
#76381=CARTESIAN_POINT('Ctrl Pts',(-2.54936288906152,-6.53425022622116,
7.1548778221625));
#76382=CARTESIAN_POINT('Ctrl Pts',(-1.9942397389208,-6.73322925932852,7.18199947573059));
#76383=CARTESIAN_POINT('Ctrl Pts',(-1.61215418065476,-6.83478887391636,
7.20013825169232));
#76384=CARTESIAN_POINT('Ctrl Pts',(-0.916971275615275,-6.9579979662812,
7.23217303126062));
#76385=CARTESIAN_POINT('Ctrl Pts',(-0.607107129938149,-6.99185220284239,
7.24613318124684));
#76386=CARTESIAN_POINT('Ctrl Pts',(-0.0462832116005817,-7.01555150281003,
7.2712762249153));
#76387=CARTESIAN_POINT('Ctrl Pts',(0.203833041020188,-7.01274223104484,
7.28245086030312));
#76388=CARTESIAN_POINT('Ctrl Pts',(0.605446245084778,-6.98672450007237,
7.30069266450485));
#76389=CARTESIAN_POINT('Ctrl Pts',(0.757267235247652,-6.97190281822153,
7.30766763574173));
#76390=CARTESIAN_POINT('Ctrl Pts',(1.3773468909258,-6.89087305560463,7.33637564536627));
#76391=CARTESIAN_POINT('Ctrl Pts',(1.83882822546788,-6.78232603573567,7.35815762439493));
#76392=CARTESIAN_POINT('Ctrl Pts',(2.56456417919663,-6.53204021135923,7.39294790552744));
#76393=CARTESIAN_POINT('Ctrl Pts',(2.83692688928799,-6.41844124762686,7.40616154980519));
#76394=CARTESIAN_POINT('Ctrl Pts',(3.33620385675422,-6.17219206857562,7.43109711662841));
#76395=CARTESIAN_POINT('Ctrl Pts',(3.56439790951083,-6.04328339588388,7.4428046961773));
#76396=CARTESIAN_POINT('Ctrl Pts',(3.9504264567158,-5.79572703475529,7.46362718872269));
#76397=CARTESIAN_POINT('Ctrl Pts',(4.11146756786985,-5.68261853786531,7.47265650678087));
#76398=CARTESIAN_POINT('Ctrl Pts',(4.57865974646798,-5.32421495768197,7.4997388599903));
#76399=CARTESIAN_POINT('Ctrl Pts',(4.86921806764402,-5.05985344130576,7.51776080969534));
#76400=CARTESIAN_POINT('Ctrl Pts',(5.35568038768731,-4.53633367375472,7.55018824509851));
#76401=CARTESIAN_POINT('Ctrl Pts',(5.55864972726014,-4.28521333430483,7.56464027532156));
#76402=CARTESIAN_POINT('Ctrl Pts',(5.88852487292474,-3.81401976693936,7.59040346364981));
#76403=CARTESIAN_POINT('Ctrl Pts',(6.02213921942784,-3.59934815944039,7.60170416789714));
#76404=CARTESIAN_POINT('Ctrl Pts',(6.23331121314428,-3.21526362284056,7.62160056012623));
#76405=CARTESIAN_POINT('Ctrl Pts',(6.31625313436411,-3.04910366744836,7.63011574732553));
#76406=CARTESIAN_POINT('Ctrl Pts',(6.56089479887711,-2.50606439460331,7.65750165480046));
#76407=CARTESIAN_POINT('Ctrl Pts',(6.69618263606603,-2.118218691752,7.67635253919336));
#76408=CARTESIAN_POINT('Ctrl Pts',(6.84524754917262,-1.5294347366303,7.70390446373839));
#76409=CARTESIAN_POINT('Ctrl Pts',(6.88558914207132,-1.33613186397445,7.71279771792521));
#76410=CARTESIAN_POINT('Ctrl Pts',(6.9610115280969,-0.879010034295987,7.73359977736443));
#76411=CARTESIAN_POINT('Ctrl Pts',(6.98933947644396,-0.61438809336215,7.74546272815319));
#76412=CARTESIAN_POINT('Ctrl Pts',(7.00952034532501,-0.209232550461513,
7.76370591127279));
#76413=CARTESIAN_POINT('Ctrl Pts',(7.01229805977016,-0.0694924325936259,
7.77001672636569));
#76414=CARTESIAN_POINT('Ctrl Pts',(7.01029982261131,0.129962593846073,7.77910349082552));
#76415=CARTESIAN_POINT('Ctrl Pts',(7.00893834569618,0.189676226231698,7.78183244713181));
#76416=CARTESIAN_POINT('Ctrl Pts',(7.00042140818598,0.428990637080506,7.79279647660735));
#76417=CARTESIAN_POINT('Ctrl Pts',(6.98712381965537,0.608303410428246,7.80107123281553));
#76418=CARTESIAN_POINT('Ctrl Pts',(6.93365284225106,1.08171419301939,7.82299107288664));
#76419=CARTESIAN_POINT('Ctrl Pts',(6.88167545139285,1.37411626381108,7.83659514747978));
#76420=CARTESIAN_POINT('Ctrl Pts',(6.75117296819582,1.9088391551483,7.86160471530203));
#76421=CARTESIAN_POINT('Ctrl Pts',(6.67767890774314,2.15188543722486,7.87302814017459));
#76422=CARTESIAN_POINT('Ctrl Pts',(6.49703095281132,2.64999206931696,7.89679526319872));
#76423=CARTESIAN_POINT('Ctrl Pts',(6.38763928098552,2.90377877040218,7.90910964409462));
#76424=CARTESIAN_POINT('Ctrl Pts',(6.20637761806247,3.2641542419812,7.92730094855199));
#76425=CARTESIAN_POINT('Ctrl Pts',(6.14610252911692,3.37627739555295,7.93307379655572));
#76426=CARTESIAN_POINT('Ctrl Pts',(5.92886033544775,3.75527286890485,7.95302480427029));
#76427=CARTESIAN_POINT('Ctrl Pts',(5.75729366458968,4.01335625066513,7.96731717573306));
#76428=CARTESIAN_POINT('Ctrl Pts',(5.42040930044206,4.45385306682423,7.99277546588871));
#76429=CARTESIAN_POINT('Ctrl Pts',(5.26148481795813,4.6405199072907,8.00395806909183));
#76430=CARTESIAN_POINT('Ctrl Pts',(4.88717717047649,5.0361610307667,8.02863737452834));
#76431=CARTESIAN_POINT('Ctrl Pts',(4.66749604956386,5.24041055144013,8.0420633623407));
#76432=CARTESIAN_POINT('Ctrl Pts',(4.23987599336553,5.58970738788746,8.06679456450268));
#76433=CARTESIAN_POINT('Ctrl Pts',(4.03584946575664,5.73875354140848,8.0780869697612));
#76434=CARTESIAN_POINT('Ctrl Pts',(3.66880549544993,5.97761502678099,8.09796571718949));
#76435=CARTESIAN_POINT('Ctrl Pts',(3.5094283338005,6.07255514015831,8.10647168292543));
#76436=CARTESIAN_POINT('Ctrl Pts',(2.98592573999628,6.35690374683526,8.13386390638225));
#76437=CARTESIAN_POINT('Ctrl Pts',(2.60886892619951,6.52072033891968,8.15273056674295));
#76438=CARTESIAN_POINT('Ctrl Pts',(2.03242699627514,6.71310843254059,8.18029770391176));
#76439=CARTESIAN_POINT('Ctrl Pts',(1.84264530607353,6.76766164683866,8.1891908756156));
#76440=CARTESIAN_POINT('Ctrl Pts',(1.39233669253338,6.87675479006558,8.20999433195249));
#76441=CARTESIAN_POINT('Ctrl Pts',(1.13050781126064,6.92461615575911,8.22185875462551));
#76442=CARTESIAN_POINT('Ctrl Pts',(0.727986095596016,6.9747525724049,8.24010091576521));
#76443=CARTESIAN_POINT('Ctrl Pts',(0.588894825797756,6.98787089403302,8.24640913248971));
#76444=CARTESIAN_POINT('Ctrl Pts',(0.389876360918287,7.00065661448197,8.25549430367158));
#76445=CARTESIAN_POINT('Ctrl Pts',(0.330203171120092,7.00372489481785,8.25822432272138));
#76446=CARTESIAN_POINT('Ctrl Pts',(0.0907604269257031,7.01296962793811,
8.26919552532952));
#76447=CARTESIAN_POINT('Ctrl Pts',(-0.0891772435494388,7.01298989936746,
8.27747641923897));
#76448=CARTESIAN_POINT('Ctrl Pts',(-0.565150720725934,6.99472057798788,
8.29939175734012));
#76449=CARTESIAN_POINT('Ctrl Pts',(-0.860371252053511,6.96457305164982,
8.31298521294926));
#76450=CARTESIAN_POINT('Ctrl Pts',(-1.40306090347226,6.87411216238591,8.33798388463364));
#76451=CARTESIAN_POINT('Ctrl Pts',(-1.65087661835399,6.81884209186505,8.34940683779166));
#76452=CARTESIAN_POINT('Ctrl Pts',(-2.16098979917076,6.67562648324292,8.37317322354868));
#76453=CARTESIAN_POINT('Ctrl Pts',(-2.42218295046466,6.58535444555105,8.38548733732131));
#76454=CARTESIAN_POINT('Ctrl Pts',(-2.79500325541901,6.43131274398579,8.40367846873569));
#76455=CARTESIAN_POINT('Ctrl Pts',(-2.91128953968702,6.37951560245342,8.40945143295155));
#76456=CARTESIAN_POINT('Ctrl Pts',(-3.30537631453778,6.19095821204386,8.4294037898352));
#76457=CARTESIAN_POINT('Ctrl Pts',(-3.5754929362007,6.03898385200246,8.44369743533632));
#76458=CARTESIAN_POINT('Ctrl Pts',(-4.03977230878579,5.73566757881892,8.46915686226971));
#76459=CARTESIAN_POINT('Ctrl Pts',(-4.23770488292853,5.59101990526327,8.48033934681214));
#76460=CARTESIAN_POINT('Ctrl Pts',(-4.66000845447045,5.24706998311381,8.50501880401818));
#76461=CARTESIAN_POINT('Ctrl Pts',(-4.87998564735673,5.04313055372814,8.51844505361271));
#76462=CARTESIAN_POINT('Ctrl Pts',(-5.26001709833127,4.64258456003735,8.54317600423241));
#76463=CARTESIAN_POINT('Ctrl Pts',(-5.42377063276552,4.45017745640206,8.55446789742397));
#76464=CARTESIAN_POINT('Ctrl Pts',(-5.68917123286956,4.10187046636537,8.57434555749507));
#76465=CARTESIAN_POINT('Ctrl Pts',(-5.79565890491001,3.94998056782896,8.58285095563357));
#76466=CARTESIAN_POINT('Ctrl Pts',(-6.1146255396035,3.45430278126104,8.60995325151693));
#76467=CARTESIAN_POINT('Ctrl Pts',(-6.303482117885,3.09628465607241,8.62853280010782));
#76468=CARTESIAN_POINT('Ctrl Pts',(-6.49976039695399,2.63077489275526,8.65145887612565));
#76469=CARTESIAN_POINT('Ctrl Pts',(-6.53703987495371,2.53672368632034,8.65603465619411));
#76470=CARTESIAN_POINT('Ctrl Pts',(-6.57226798695174,2.4419091035887,8.66059774113391));
#76471=CARTESIAN_POINT('Origin',(0.,0.,10.));
#76472=CARTESIAN_POINT('',(-6.57243166141306,2.44196984210433,10.6603064506077));
#76473=CARTESIAN_POINT('',(-6.5722680052526,2.44190905433291,10.1130597871067));
#76474=CARTESIAN_POINT('',(-6.57226799596304,2.44190907933527,10.));
#76475=CARTESIAN_POINT('Ctrl Pts',(-6.5722680052526,2.44190905433291,10.1130597871067));
#76476=CARTESIAN_POINT('Ctrl Pts',(-6.52306249854838,2.57434305175004,10.1065737603578));
#76477=CARTESIAN_POINT('Ctrl Pts',(-6.46985951358318,2.70527517963783,10.1001055101174));
#76478=CARTESIAN_POINT('Ctrl Pts',(-6.32488472488106,3.03326103144295,10.0837545771268));
#76479=CARTESIAN_POINT('Ctrl Pts',(-6.22784833295103,3.22780835883114,10.0739189085502));
#76480=CARTESIAN_POINT('Ctrl Pts',(-5.9748362847281,3.68103613936886,10.0505463449007));
#76481=CARTESIAN_POINT('Ctrl Pts',(-5.81088110802064,3.93476256014785,10.03708876919));
#76482=CARTESIAN_POINT('Ctrl Pts',(-5.53767751847233,4.30306143336315,10.016498894731));
#76483=CARTESIAN_POINT('Ctrl Pts',(-5.44006918617429,4.42581704400765,10.0094359335946));
#76484=CARTESIAN_POINT('Ctrl Pts',(-5.19933764260226,4.70856117751045,9.9925424234154));
#76485=CARTESIAN_POINT('Ctrl Pts',(-5.05282373972641,4.86545277012714,9.98267705736606));
#76486=CARTESIAN_POINT('Ctrl Pts',(-4.73235369833136,5.17850889803249,9.96206347538926));
#76487=CARTESIAN_POINT('Ctrl Pts',(-4.55731367266609,5.33319977309406,9.95132800918116));
#76488=CARTESIAN_POINT('Ctrl Pts',(-4.29653885739566,5.54142866301973,9.93607606030169));
#76489=CARTESIAN_POINT('Ctrl Pts',(-4.21686177588699,5.60229906250303,9.93150689483303));
#76490=CARTESIAN_POINT('Ctrl Pts',(-3.77470075403087,5.92531520321396,9.90662465693136));
#76491=CARTESIAN_POINT('Ctrl Pts',(-3.38907093348138,6.15401727778345,9.88669807223162));
#76492=CARTESIAN_POINT('Ctrl Pts',(-2.83386247311823,6.41517605053325,9.85916513346686));
#76493=CARTESIAN_POINT('Ctrl Pts',(-2.68097131019242,6.48055955191551,9.85168435875302));
#76494=CARTESIAN_POINT('Ctrl Pts',(-2.31131340663199,6.62332043371386,9.83366594610008));
#76495=CARTESIAN_POINT('Ctrl Pts',(-2.09277764516773,6.69558233159228,9.82308374159923));
#76496=CARTESIAN_POINT('Ctrl Pts',(-1.64838554617929,6.81864000392244,9.80186601458179));
#76497=CARTESIAN_POINT('Ctrl Pts',(-1.42276758996983,6.86926201646625,9.79124371790561));
#76498=CARTESIAN_POINT('Ctrl Pts',(-1.0964457643642,6.92570929457335,9.77611496619395));
#76499=CARTESIAN_POINT('Ctrl Pts',(-0.997475895118887,6.9406544812964,9.77155613742358));
#76500=CARTESIAN_POINT('Ctrl Pts',(-0.480303663538549,7.00746051789475,
9.74787252662963));
#76501=CARTESIAN_POINT('Ctrl Pts',(-0.0583710251337542,7.02365946094005,
9.72907936535576));
#76502=CARTESIAN_POINT('Ctrl Pts',(0.541417106205394,6.99261079667883,9.70214524135545));
#76503=CARTESIAN_POINT('Ctrl Pts',(0.719951963275518,6.97648951629683,9.69409064615829));
#76504=CARTESIAN_POINT('Ctrl Pts',(1.14176797158952,6.92203503604771,9.67476117077906));
#76505=CARTESIAN_POINT('Ctrl Pts',(1.38403433580727,6.87769216829246,9.66343315709252));
#76506=CARTESIAN_POINT('Ctrl Pts',(1.84176431974649,6.76874329954472,9.64178304383793));
#76507=CARTESIAN_POINT('Ctrl Pts',(2.05744675854432,6.70633255035689,9.63147209869686));
#76508=CARTESIAN_POINT('Ctrl Pts',(2.36443991445152,6.60129252397757,9.61665346488913));
#76509=CARTESIAN_POINT('Ctrl Pts',(2.45841029581005,6.56687582930091,9.61209676286884));
#76510=CARTESIAN_POINT('Ctrl Pts',(2.92769925970198,6.38351300008897,9.58922060570921));
#76511=CARTESIAN_POINT('Ctrl Pts',(3.29039064335857,6.20435295804079,9.5711984704639));
#76512=CARTESIAN_POINT('Ctrl Pts',(3.79754115590281,5.89679217765715,9.54460903757734));
#76513=CARTESIAN_POINT('Ctrl Pts',(3.9553922990875,5.79209346990283,9.53610539920755));
#76514=CARTESIAN_POINT('Ctrl Pts',(4.31626357768206,5.53109788925574,9.51587089656991));
#76515=CARTESIAN_POINT('Ctrl Pts',(4.51534124354985,5.36981059708608,9.50408330018529));
#76516=CARTESIAN_POINT('Ctrl Pts',(4.9259522138198,4.99813192077069,9.47859969769539));
#76517=CARTESIAN_POINT('Ctrl Pts',(5.13379949899486,4.78439502432016,9.46493704518687));
#76518=CARTESIAN_POINT('Ctrl Pts',(5.48720921341611,4.37133488637111,9.44022600139232));
#76519=CARTESIAN_POINT('Ctrl Pts',(5.63706364942304,4.17630818388459,9.42915153440589));
#76520=CARTESIAN_POINT('Ctrl Pts',(5.90602258953739,3.78534718926906,9.40785548819564));
#76521=CARTESIAN_POINT('Ctrl Pts',(6.02637480900709,3.59064929418081,9.39763956176396));
#76522=CARTESIAN_POINT('Ctrl Pts',(6.21056442729317,3.25724776568287,9.38053113053101));
#76523=CARTESIAN_POINT('Ctrl Pts',(6.27977959979397,3.12172084876334,9.37367368227847));
#76524=CARTESIAN_POINT('Ctrl Pts',(6.45048108308314,2.75878414798111,9.35542208953705));
#76525=CARTESIAN_POINT('Ctrl Pts',(6.54435752457093,2.52803847623592,9.34395820172231));
#76526=CARTESIAN_POINT('Ctrl Pts',(6.72735503274035,1.99920825489445,9.31821125602443));
#76527=CARTESIAN_POINT('Ctrl Pts',(6.80932402937067,1.69919149110987,9.30396990429992));
#76528=CARTESIAN_POINT('Ctrl Pts',(6.9508579923896,1.00192342681966,9.27166721102043));
#76529=CARTESIAN_POINT('Ctrl Pts',(6.99676109633989,0.603006297637533,9.25377487970263));
#76530=CARTESIAN_POINT('Ctrl Pts',(7.01384654298695,0.0112696508311266,
9.22723807018616));
#76531=CARTESIAN_POINT('Ctrl Pts',(7.01154643762042,-0.179958336348825,
9.2186537642296));
#76532=CARTESIAN_POINT('Ctrl Pts',(6.98781153254607,-0.628059652340506,
9.19826715697476));
#76533=CARTESIAN_POINT('Ctrl Pts',(6.96002468049761,-0.884320427785898,
9.18640778524028));
#76534=CARTESIAN_POINT('Ctrl Pts',(6.86997095384255,-1.43155621023386,9.16088988512966));
#76535=CARTESIAN_POINT('Ctrl Pts',(6.8031628425897,-1.72128862521069,9.14726442991084));
#76536=CARTESIAN_POINT('Ctrl Pts',(6.58252384264637,-2.460250458762,9.11220892700226));
#76537=CARTESIAN_POINT('Ctrl Pts',(6.40112923711657,-2.8996551433947,9.09111831115912));
#76538=CARTESIAN_POINT('Ctrl Pts',(6.10470015985463,-3.45158941117204,9.06297879121011));
#76539=CARTESIAN_POINT('Ctrl Pts',(6.02826775626454,-3.58340909283533,9.05611263840986));
#76540=CARTESIAN_POINT('Ctrl Pts',(5.81548979845143,-3.9242771284782,9.03782709248574));
#76541=CARTESIAN_POINT('Ctrl Pts',(5.67217631503019,-4.12871483491063,9.02633746418278));
#76542=CARTESIAN_POINT('Ctrl Pts',(5.3265045558147,-4.56975016447565,9.00055562000652));
#76543=CARTESIAN_POINT('Ctrl Pts',(5.11867186270924,-4.80140310835969,8.9863052672367));
#76544=CARTESIAN_POINT('Ctrl Pts',(4.61111094785965,-5.29658982754405,8.95411204565464));
#76545=CARTESIAN_POINT('Ctrl Pts',(4.30289684196993,-5.5498911523295,8.93633320629322));
#76546=CARTESIAN_POINT('Ctrl Pts',(3.81603612646447,-5.88495211316567,8.90984107205694));
#76547=CARTESIAN_POINT('Ctrl Pts',(3.65278628473325,-5.98764924688596,8.90118498275196));
#76548=CARTESIAN_POINT('Ctrl Pts',(3.26088112457885,-6.21219008742089,8.88066544492403));
#76549=CARTESIAN_POINT('Ctrl Pts',(3.02929355460453,-6.32835121935764,8.86874470152901));
#76550=CARTESIAN_POINT('Ctrl Pts',(2.51997388677688,-6.54944131925157,8.84319749054508));
#76551=CARTESIAN_POINT('Ctrl Pts',(2.24091891656945,-6.65009304239442,8.82960383781908));
#76552=CARTESIAN_POINT('Ctrl Pts',(1.50138084998935,-6.86497899366382,8.79459775666959));
#76553=CARTESIAN_POINT('Ctrl Pts',(1.03420446707213,-6.95071975838244,8.77352440681931));
#76554=CARTESIAN_POINT('Ctrl Pts',(0.410061592315048,-7.00090695148839,
8.74540036509224));
#76555=CARTESIAN_POINT('Ctrl Pts',(0.257809106965031,-7.0081654146418,8.73853201614708));
#76556=CARTESIAN_POINT('Ctrl Pts',(-0.144162428614273,-7.01421124997964,
8.72023791696903));
#76557=CARTESIAN_POINT('Ctrl Pts',(-0.393785461806843,-7.00463225536466,
8.70874180757832));
#76558=CARTESIAN_POINT('Ctrl Pts',(-0.949724728195507,-6.95348264739962,
8.68305525776462));
#76559=CARTESIAN_POINT('Ctrl Pts',(-1.25488927211388,-6.90493713606302,
8.66890556627461));
#76560=CARTESIAN_POINT('Ctrl Pts',(-1.95229047918078,-6.74621986211733,
8.63642989490286));
#76561=CARTESIAN_POINT('Ctrl Pts',(-2.34011993582507,-6.62168892721861,
8.6182856313818));
#76562=CARTESIAN_POINT('Ctrl Pts',(-2.88798771241883,-6.39158579860027,
8.59164522398319));
#76563=CARTESIAN_POINT('Ctrl Pts',(-3.05801587784929,-6.31200278752193,
8.58321611055528));
#76564=CARTESIAN_POINT('Ctrl Pts',(-3.45066283957357,-6.1086284815956,8.56312478075359));
#76565=CARTESIAN_POINT('Ctrl Pts',(-3.67013647425846,-5.97934039092137,
8.55140622656641));
#76566=CARTESIAN_POINT('Ctrl Pts',(-4.13073579231001,-5.67307736553466,
8.52595562911345));
#76567=CARTESIAN_POINT('Ctrl Pts',(-4.368569225362,-5.49202995873933,8.5122571872988));
#76568=CARTESIAN_POINT('Ctrl Pts',(-4.77954508892193,-5.13554440964608,
8.48752615733592));
#76569=CARTESIAN_POINT('Ctrl Pts',(-4.95638245587944,-4.96509250449275,
8.47646651286933));
#76570=CARTESIAN_POINT('Ctrl Pts',(-5.28145399943499,-4.61704846891906,
8.45509367418528));
#76571=CARTESIAN_POINT('Ctrl Pts',(-5.43056447597842,-4.44070511060848,
8.44478727944677));
#76572=CARTESIAN_POINT('Ctrl Pts',(-5.66258984337376,-4.13710052436134,
8.42762300383097));
#76573=CARTESIAN_POINT('Ctrl Pts',(-5.75055568861366,-4.01392988718079,
8.42080180513171));
#76574=CARTESIAN_POINT('Ctrl Pts',(-5.97122053793642,-3.68279332144224,
8.40269256413441));
#76575=CARTESIAN_POINT('Ctrl Pts',(-6.09704987474239,-3.47050745435505,
8.39133683572029));
#76576=CARTESIAN_POINT('Ctrl Pts',(-6.35313379357093,-2.98138391713033,
8.36593423935645));
#76577=CARTESIAN_POINT('Ctrl Pts',(-6.47699679207328,-2.70175448959318,
8.35192629616431));
#76578=CARTESIAN_POINT('Ctrl Pts',(-6.73998857089557,-1.98493568398216,
8.3172457257361));
#76579=CARTESIAN_POINT('Ctrl Pts',(-6.8552346756514,-1.54051160563081,8.29686619026766));
#76580=CARTESIAN_POINT('Ctrl Pts',(-6.9502696003491,-0.935526679806157,
8.26936414495472));
#76581=CARTESIAN_POINT('Ctrl Pts',(-6.96918215409512,-0.782276873447443,
8.26240806471864));
#76582=CARTESIAN_POINT('Ctrl Pts',(-7.00182587171905,-0.419600882761046,
8.24583967508274));
#76583=CARTESIAN_POINT('Ctrl Pts',(-7.01124487977592,-0.209937821647998,
8.23619565108158));
#76584=CARTESIAN_POINT('Ctrl Pts',(-7.01125830046331,0.34010878522083,8.2108872257868));
#76585=CARTESIAN_POINT('Ctrl Pts',(-6.98649416202547,0.679943913064139,
8.19526116620574));
#76586=CARTESIAN_POINT('Ctrl Pts',(-6.89996407488868,1.27039215559498,8.16814954332841));
#76587=CARTESIAN_POINT('Ctrl Pts',(-6.84888113152541,1.52191686087706,8.15660574827463));
#76588=CARTESIAN_POINT('Ctrl Pts',(-6.72480522780128,1.99745896547295,8.13456370998852));
#76589=CARTESIAN_POINT('Ctrl Pts',(-6.65409201294924,2.22168410121299,8.12407245122135));
#76590=CARTESIAN_POINT('Ctrl Pts',(-6.57226800401825,2.44190905765509,8.11350492783088));
#76591=CARTESIAN_POINT('',(-7.01100200678231,0.000169534895841095,8.77353435691038));
#76592=CARTESIAN_POINT('Ctrl Pts',(-6.57226798695174,2.4419091035887,8.66059774113391));
#76593=CARTESIAN_POINT('Ctrl Pts',(-6.60582227508257,2.35159952843576,8.66494401625771));
#76594=CARTESIAN_POINT('Ctrl Pts',(-6.63751550112601,2.26059739590921,8.66927879456213));
#76595=CARTESIAN_POINT('Ctrl Pts',(-6.78113365131024,1.8191190086922,8.6901281620384));
#76596=CARTESIAN_POINT('Ctrl Pts',(-6.8672279976668,1.4608691468603,8.70647653024955));
#76597=CARTESIAN_POINT('Ctrl Pts',(-6.93320891013727,1.04456516083428,8.72558511308945));
#76598=CARTESIAN_POINT('Ctrl Pts',(-6.94099522164981,0.991507640171676,
8.72802374985079));
#76599=CARTESIAN_POINT('Ctrl Pts',(-6.99016893737213,0.62739884410733,8.74477747392914));
#76600=CARTESIAN_POINT('Ctrl Pts',(-7.01124211628482,0.313964344255776,
8.75926542393631));
#76601=CARTESIAN_POINT('Ctrl Pts',(-7.01124999778838,0.000176103450165235,
8.77367723833414));
#76602=CARTESIAN_POINT('Ctrl Pts',(-7.01100200678231,0.000169534895841095,
8.77353435691038));
#76603=CARTESIAN_POINT('Ctrl Pts',(-7.01026859459823,-0.814242395437865,
8.81050553539818));
#76604=CARTESIAN_POINT('Ctrl Pts',(-6.66540157732887,-2.79524324339015,
8.90040791439849));
#76605=CARTESIAN_POINT('Ctrl Pts',(-4.83841745661552,-5.47793893682926,
9.0432414939113));
#76606=CARTESIAN_POINT('Ctrl Pts',(-1.62793640627636,-7.12516115868475,
9.20203509544883));
#76607=CARTESIAN_POINT('Ctrl Pts',(1.97935012394701,-7.03564293913092,9.36082869698635));
#76608=CARTESIAN_POINT('Ctrl Pts',(5.10417494819451,-5.23120412317588,9.51962229852384));
#76609=CARTESIAN_POINT('Ctrl Pts',(6.98486973030968,-2.15167221730337,9.67841590006139));
#76610=CARTESIAN_POINT('Ctrl Pts',(7.16301976032167,1.45232447936148,9.83720950159888));
#76611=CARTESIAN_POINT('Ctrl Pts',(5.59520140824282,4.70232066976576,9.99600310313642));
#76612=CARTESIAN_POINT('Ctrl Pts',(2.66356652666938,6.80613780628324,10.1547967046739));
#76613=CARTESIAN_POINT('Ctrl Pts',(-0.917306119809289,7.25097565591498,
10.3135903062114));
#76614=CARTESIAN_POINT('Ctrl Pts',(-4.27458766428332,5.92840609105567,10.472383907749));
#76615=CARTESIAN_POINT('Ctrl Pts',(-5.95973776688883,3.91410797347048,10.5879559558811));
#76616=CARTESIAN_POINT('Ctrl Pts',(-6.49815987240321,2.64250790562492,10.6505968035006));
#76617=CARTESIAN_POINT('Ctrl Pts',(-6.57243166141306,2.44196984210433,10.6603064506077));
#76618=CARTESIAN_POINT('Origin',(0.,0.,10.));
#76619=CARTESIAN_POINT('',(-6.57226799596304,2.44190907933527,12.6602932967));
#76620=CARTESIAN_POINT('',(-6.57226802086842,2.44190901230376,12.1131304899038));
#76621=CARTESIAN_POINT('',(-6.57226799596304,2.44190907933527,10.));
#76622=CARTESIAN_POINT('',(-7.01124982808863,8.84455196530982E-5,10.2261740575975));
#76623=CARTESIAN_POINT('Ctrl Pts',(-6.57226802086842,2.44190901230376,12.1131304899038));
#76624=CARTESIAN_POINT('Ctrl Pts',(-6.54688037716058,2.510238502889,12.1098623793163));
#76625=CARTESIAN_POINT('Ctrl Pts',(-6.52042381490871,2.57818101884485,12.1065967925351));
#76626=CARTESIAN_POINT('Ctrl Pts',(-6.39754489276982,2.87974127567772,12.0920113248996));
#76627=CARTESIAN_POINT('Ctrl Pts',(-6.28960118708034,3.10844066455065,12.0807090018542));
#76628=CARTESIAN_POINT('Ctrl Pts',(-6.08133977191838,3.49419657965324,12.0608091758205));
#76629=CARTESIAN_POINT('Ctrl Pts',(-5.98667559978145,3.65401373965553,12.0522921980193));
#76630=CARTESIAN_POINT('Ctrl Pts',(-5.66304324527052,4.15398440660527,12.0249075181839));
#76631=CARTESIAN_POINT('Ctrl Pts',(-5.41055224263107,4.47789936037004,12.0060596981926));
#76632=CARTESIAN_POINT('Ctrl Pts',(-4.99670412879478,4.92235030328896,11.9785107312699));
#76633=CARTESIAN_POINT('Ctrl Pts',(-4.85615757561548,5.06105916070442,11.969617463602));
#76634=CARTESIAN_POINT('Ctrl Pts',(-4.51296656268245,5.37228717321997,11.9488156792853));
#76635=CARTESIAN_POINT('Ctrl Pts',(-4.30598638440878,5.53956828976701,11.9369530156526));
#76636=CARTESIAN_POINT('Ctrl Pts',(-3.97649833014791,5.7762113863267,11.9187096344546));
#76637=CARTESIAN_POINT('Ctrl Pts',(-3.860579971078,5.85432137669194,11.9123983137699));
#76638=CARTESIAN_POINT('Ctrl Pts',(-3.69190062837516,5.96079383079722,11.9033112408894));
#76639=CARTESIAN_POINT('Ctrl Pts',(-3.64099253422944,5.99202525316997,11.9005824929819));
#76640=CARTESIAN_POINT('Ctrl Pts',(-3.43531952709893,6.11461391166622,11.8896198684564));
#76641=CARTESIAN_POINT('Ctrl Pts',(-3.27746717410528,6.20065576499953,11.8813463141605));
#76642=CARTESIAN_POINT('Ctrl Pts',(-2.85068187444628,6.41243220611299,11.8594255952862));
#76643=CARTESIAN_POINT('Ctrl Pts',(-2.57677013962033,6.52732217601357,11.8458194439498));
#76644=CARTESIAN_POINT('Ctrl Pts',(-2.05666919306168,6.70761628081339,11.8208077533866));
#76645=CARTESIAN_POINT('Ctrl Pts',(-1.8126002273792,6.7776461931263,11.8093842442754));
#76646=CARTESIAN_POINT('Ctrl Pts',(-1.29611754215166,6.89593714449807,11.7856169877211));
#76647=CARTESIAN_POINT('Ctrl Pts',(-1.0235606759597,6.9416273948252,11.7733025572706));
#76648=CARTESIAN_POINT('Ctrl Pts',(-0.622475285271074,6.98472264459883,
11.7551112226141));
#76649=CARTESIAN_POINT('Ctrl Pts',(-0.495583421257757,6.99487114048289,
11.7493383980851));
#76650=CARTESIAN_POINT('Ctrl Pts',(-0.0593498600627373,7.01782969787626,
11.7293876408584));
#76651=CARTESIAN_POINT('Ctrl Pts',(0.250523006141232,7.0136077617466,11.715095503905));
#76652=CARTESIAN_POINT('Ctrl Pts',(0.803304932241008,6.96938630858188,11.6896374249949));
#76653=CARTESIAN_POINT('Ctrl Pts',(1.04632136718118,6.93706417033835,11.6784548019303));
#76654=CARTESIAN_POINT('Ctrl Pts',(1.58170857792281,6.83707654822773,11.6537755424015));
#76655=CARTESIAN_POINT('Ctrl Pts',(1.87243985733845,6.76323814672692,11.6403496183861));
#76656=CARTESIAN_POINT('Ctrl Pts',(2.39779553592898,6.59332655335917,11.6156183615674));
#76657=CARTESIAN_POINT('Ctrl Pts',(2.63365842278843,6.50270849579327,11.604325838146));
#76658=CARTESIAN_POINT('Ctrl Pts',(3.03338002602547,6.32381385964298,11.5844468525831));
#76659=CARTESIAN_POINT('Ctrl Pts',(3.19957102729586,6.24137479594769,11.5759407688705));
#76660=CARTESIAN_POINT('Ctrl Pts',(3.72233968819918,5.95568311434478,11.548548631502));
#76661=CARTESIAN_POINT('Ctrl Pts',(4.06442595428536,5.72768965777138,11.5296821782738));
#76662=CARTESIAN_POINT('Ctrl Pts',(4.53862858620379,5.34765695030548,11.5021152436343));
#76663=CARTESIAN_POINT('Ctrl Pts',(4.68736831651953,5.21777386773328,11.4932220736018));
#76664=CARTESIAN_POINT('Ctrl Pts',(5.02319521206397,4.89855769729015,11.4724186402161));
#76665=CARTESIAN_POINT('Ctrl Pts',(5.20537674174289,4.70450948948079,11.4605542387343));
#76666=CARTESIAN_POINT('Ctrl Pts',(5.46575576958667,4.39347826842278,11.4423120647569));
#76667=CARTESIAN_POINT('Ctrl Pts',(5.55219576982442,4.28372024148265,11.4360038125229));
#76668=CARTESIAN_POINT('Ctrl Pts',(5.67084927962669,4.12342879355375,11.4269186217153));
#76669=CARTESIAN_POINT('Ctrl Pts',(5.70578267369711,4.07495283090559,11.4241886193547));
#76670=CARTESIAN_POINT('Ctrl Pts',(5.84337779263442,3.87877760274942,11.4132175281794));
#76671=CARTESIAN_POINT('Ctrl Pts',(5.9409581141614,3.72759920816807,11.4049367294474));
#76672=CARTESIAN_POINT('Ctrl Pts',(6.1836870029801,3.31775954576857,11.3830213258525));
#76673=CARTESIAN_POINT('Ctrl Pts',(6.31842947375525,3.05335348781755,11.3694277098683));
#76674=CARTESIAN_POINT('Ctrl Pts',(6.53667426233892,2.54831071221083,11.3444288829191));
#76675=CARTESIAN_POINT('Ctrl Pts',(6.6246024980283,2.31011748703655,11.3330059317448));
#76676=CARTESIAN_POINT('Ctrl Pts',(6.78085586132641,1.80384579524083,11.3092395472092));
#76677=CARTESIAN_POINT('Ctrl Pts',(6.84662738764625,1.53543376379101,11.2969254326983));
#76678=CARTESIAN_POINT('Ctrl Pts',(6.9193424539647,1.1386513077578,11.2787343027459));
#76679=CARTESIAN_POINT('Ctrl Pts',(6.93887204987628,1.01285772368272,11.2729613408046));
#76680=CARTESIAN_POINT('Ctrl Pts',(6.99411650599425,0.579491538137023,11.2530089878428));
#76681=CARTESIAN_POINT('Ctrl Pts',(7.01288154990812,0.270125983085059,11.2387153439766));
#76682=CARTESIAN_POINT('Ctrl Pts',(7.00976000242406,-0.284442560050966,
11.2132559204942));
#76683=CARTESIAN_POINT('Ctrl Pts',(6.99554223374986,-0.529183419687476,
11.2020734377709));
#76684=CARTESIAN_POINT('Ctrl Pts',(6.93551887943285,-1.07051382935617,11.177393998748));
#76685=CARTESIAN_POINT('Ctrl Pts',(6.88343461022993,-1.36592585795191,11.1639677651249));
#76686=CARTESIAN_POINT('Ctrl Pts',(6.7529364207787,-1.90242509710265,11.1392368058035));
#76687=CARTESIAN_POINT('Ctrl Pts',(6.68005675044703,-2.1443435737848,11.1279448879996));
#76688=CARTESIAN_POINT('Ctrl Pts',(6.53129745292929,-2.55620115303456,11.1080671884675));
#76689=CARTESIAN_POINT('Ctrl Pts',(6.46141185244808,-2.72803328700361,11.0995617760702));
#76690=CARTESIAN_POINT('Ctrl Pts',(6.21526106737558,-3.27055412443705,11.0721691776359));
#76691=CARTESIAN_POINT('Ctrl Pts',(6.01324377531958,-3.6286232593302,11.0533015746088));
#76692=CARTESIAN_POINT('Ctrl Pts',(5.6693958452331,-4.12971367414453,11.0257335311834));
#76693=CARTESIAN_POINT('Ctrl Pts',(5.55089638603365,-4.28767246413541,11.0168403670962));
#76694=CARTESIAN_POINT('Ctrl Pts',(5.25745219872648,-4.6462409890206,10.9960368316422));
#76695=CARTESIAN_POINT('Ctrl Pts',(5.07744145015366,-4.84230793918049,10.9841723226927));
#76696=CARTESIAN_POINT('Ctrl Pts',(4.78656922893734,-5.12502597446008,10.9659302231568));
#76697=CARTESIAN_POINT('Ctrl Pts',(4.68352425510897,-5.21936167744688,10.9596221604644));
#76698=CARTESIAN_POINT('Ctrl Pts',(4.53247185432463,-5.3495696702889,10.950537085712));
#76699=CARTESIAN_POINT('Ctrl Pts',(4.48671765610269,-5.38800161170629,10.947807005657));
#76700=CARTESIAN_POINT('Ctrl Pts',(4.30127349055091,-5.53976800604108,10.9368353899342));
#76701=CARTESIAN_POINT('Ctrl Pts',(4.15773684077934,-5.64829239824263,10.9285541423525));
#76702=CARTESIAN_POINT('Ctrl Pts',(3.76702328059213,-5.92072960200588,10.9066390675196));
#76703=CARTESIAN_POINT('Ctrl Pts',(3.513347622996,-6.07469316738086,10.8930462276176));
#76704=CARTESIAN_POINT('Ctrl Pts',(3.02588949854575,-6.32977015746142,10.8680481966715));
#76705=CARTESIAN_POINT('Ctrl Pts',(2.79487091834758,-6.43511439030879,10.8566252796366));
#76706=CARTESIAN_POINT('Ctrl Pts',(2.30157723395587,-6.62846949614994,10.8328589484629));
#76707=CARTESIAN_POINT('Ctrl Pts',(2.03878015831692,-6.71395849365647,10.8205448532881));
#76708=CARTESIAN_POINT('Ctrl Pts',(1.64848046451444,-6.81588871745719,10.8023537358482));
#76709=CARTESIAN_POINT('Ctrl Pts',(1.52448064134744,-6.84469027216798,10.7965807654815));
#76710=CARTESIAN_POINT('Ctrl Pts',(1.09640033669328,-6.93191053547969,10.7766283148612));
#76711=CARTESIAN_POINT('Ctrl Pts',(0.789275225705136,-6.97355874183667,
10.7623345787885));
#76712=CARTESIAN_POINT('Ctrl Pts',(0.235999473876122,-7.01155810215142,
10.7368750730369));
#76713=CARTESIAN_POINT('Ctrl Pts',(-0.00912176680378921,-7.01552299826439,
10.7256925989047));
#76714=CARTESIAN_POINT('Ctrl Pts',(-0.553412606382337,-6.99579564682385,
10.7010131488923));
#76715=CARTESIAN_POINT('Ctrl Pts',(-0.851873382630387,-6.96575462400956,
10.6875868963149));
#76716=CARTESIAN_POINT('Ctrl Pts',(-1.39657024243448,-6.87538818450214,
10.6628559552064));
#76717=CARTESIAN_POINT('Ctrl Pts',(-1.64322505556015,-6.82064355797329,
10.6515640744785));
#76718=CARTESIAN_POINT('Ctrl Pts',(-2.0649757731466,-6.7028266784728,10.6316864536703));
#76719=CARTESIAN_POINT('Ctrl Pts',(-2.241515136561,-6.64587227581451,10.6231810823639));
#76720=CARTESIAN_POINT('Ctrl Pts',(-2.80079190623852,-6.44061801051559,
10.5957884557022));
#76721=CARTESIAN_POINT('Ctrl Pts',(-3.17285346079602,-6.26570104768405,
10.5769207822906));
#76722=CARTESIAN_POINT('Ctrl Pts',(-3.69805703859718,-5.95994617579252,
10.549352670991));
#76723=CARTESIAN_POINT('Ctrl Pts',(-3.86436596968462,-5.85348285204863,
10.5404595072674));
#76724=CARTESIAN_POINT('Ctrl Pts',(-4.24370203358389,-5.58742803797586,
10.5196559655641));
#76725=CARTESIAN_POINT('Ctrl Pts',(-4.45257443430411,-5.422447680154,10.5077914500351));
#76726=CARTESIAN_POINT('Ctrl Pts',(-4.75607783328552,-5.15333482244536,
10.4895493550559));
#76727=CARTESIAN_POINT('Ctrl Pts',(-4.85779286038752,-5.05756702575083,
10.483241303967));
#76728=CARTESIAN_POINT('Ctrl Pts',(-4.99884051926767,-4.91658318781238,
10.4741562363185));
#76729=CARTESIAN_POINT('Ctrl Pts',(-5.04055870617977,-4.87380391841118,
10.4714261515064));
#76730=CARTESIAN_POINT('Ctrl Pts',(-5.20565561878988,-4.70012052963085,
10.4604545036656));
#76731=CARTESIAN_POINT('Ctrl Pts',(-5.32452265652367,-4.56502369617191,
10.4521732286008));
#76732=CARTESIAN_POINT('Ctrl Pts',(-5.62112227210478,-4.2005620928327,10.4305535735194));
#76733=CARTESIAN_POINT('Ctrl Pts',(-5.7900515260717,-3.96447293077758,10.4172532673156));
#76734=CARTESIAN_POINT('Ctrl Pts',(-6.05025523930506,-3.54855865402196,
10.3949528946717));
#76735=CARTESIAN_POINT('Ctrl Pts',(-6.14929087420723,-3.3740303049451,10.3858983310391));
#76736=CARTESIAN_POINT('Ctrl Pts',(-6.37408834214991,-2.93500734957092,
10.3637259735005));
#76737=CARTESIAN_POINT('Ctrl Pts',(-6.49102774827429,-2.66642608209169,
10.3506794603042));
#76738=CARTESIAN_POINT('Ctrl Pts',(-6.63611703659724,-2.2665389844744,10.3315525730326));
#76739=CARTESIAN_POINT('Ctrl Pts',(-6.67783909290207,-2.1404936139626,10.3255617227238));
#76740=CARTESIAN_POINT('Ctrl Pts',(-6.74796060119245,-1.906587122782,10.3144495070837));
#76741=CARTESIAN_POINT('Ctrl Pts',(-6.77741310604404,-1.79908807295501,
10.3093488189413));
#76742=CARTESIAN_POINT('Ctrl Pts',(-6.89976228177878,-1.30675695056456,
10.286066241257));
#76743=CARTESIAN_POINT('Ctrl Pts',(-6.96252792258015,-0.915175995298078,
10.267808296208));
#76744=CARTESIAN_POINT('Ctrl Pts',(-7.00480120457911,-0.347201324706604,
10.2418684589118));
#76745=CARTESIAN_POINT('Ctrl Pts',(-7.01125219422837,-0.1735872788153,10.2340036335229));
#76746=CARTESIAN_POINT('Ctrl Pts',(-7.01124999944015,8.86030272035515E-5,
10.2261737535422));
#76747=CARTESIAN_POINT('Ctrl Pts',(-7.01124999944231,8.84321612436983E-5,
10.2261737612454));
#76748=CARTESIAN_POINT('Ctrl Pts',(-7.01124533029536,0.370276789916301,
10.2094844524627));
#76749=CARTESIAN_POINT('Ctrl Pts',(-6.98192239085777,0.739881399521689,
10.1930195260008));
#76750=CARTESIAN_POINT('Ctrl Pts',(-6.90640727853726,1.21284610091569,10.1714608011783));
#76751=CARTESIAN_POINT('Ctrl Pts',(-6.88676134899585,1.31983900532265,10.1665477865801));
#76752=CARTESIAN_POINT('Ctrl Pts',(-6.8068752874671,1.70431378819719,10.1486905702379));
#76753=CARTESIAN_POINT('Ctrl Pts',(-6.73228487181659,1.97852834723244,10.1356004187491));
#76754=CARTESIAN_POINT('Ctrl Pts',(-6.61922587762499,2.31261910254185,10.1193784660519));
#76755=CARTESIAN_POINT('Ctrl Pts',(-6.59622056257768,2.37744202355948,10.1162170948538));
#76756=CARTESIAN_POINT('Ctrl Pts',(-6.5722680052526,2.44190905433291,10.1130597871067));
#76757=CARTESIAN_POINT('',(-7.01124999902902,-0.00011668600800139,10.7735343569104));
#76758=CARTESIAN_POINT('Ctrl Pts',(-6.57243166141306,2.44196984210433,10.6603064506077));
#76759=CARTESIAN_POINT('Ctrl Pts',(-6.86113553316664,1.66245293340731,10.6980490814309));
#76760=CARTESIAN_POINT('Ctrl Pts',(-7.01103588237741,0.831054505111012,
10.735791712254));
#76761=CARTESIAN_POINT('Ctrl Pts',(-7.01168925918796,-0.000116388681771435,
10.7735343430772));
#76762=CARTESIAN_POINT('Ctrl Pts',(-7.01124999902902,-0.00011668600800139,
10.7735343569104));
#76763=CARTESIAN_POINT('Ctrl Pts',(-7.01124799109669,-0.120766245883287,
10.7790132748816));
#76764=CARTESIAN_POINT('Ctrl Pts',(-7.00813125367059,-0.241405380892823,
10.7844921928528));
#76765=CARTESIAN_POINT('Ctrl Pts',(-7.00190453737324,-0.361883146902471,
10.789971110824));
#76766=CARTESIAN_POINT('Ctrl Pts',(-6.99220925361489,-0.549472571609852,
10.7985020381833));
#76767=CARTESIAN_POINT('Ctrl Pts',(-6.97496935380637,-0.736704258608883,
10.8070329655426));
#76768=CARTESIAN_POINT('Ctrl Pts',(-6.95023495748845,-0.922962945196363,
10.8155638929019));
#76769=CARTESIAN_POINT('Ctrl Pts',(-6.92550525696389,-1.10918627081151,
10.8240932006755));
#76770=CARTESIAN_POINT('Ctrl Pts',(-6.89328393961082,-1.29443666124397,
10.8326225084492));
#76771=CARTESIAN_POINT('Ctrl Pts',(-6.85367284810497,-1.47810522414635,
10.8411518162229));
#76772=CARTESIAN_POINT('Ctrl Pts',(-6.81202562040045,-1.67121493585999,
10.8501195575678));
#76773=CARTESIAN_POINT('Ctrl Pts',(-6.76220895396378,-1.86257555729251,
10.8590872989127));
#76774=CARTESIAN_POINT('Ctrl Pts',(-6.70440205432244,-2.0514920561623,10.8680550402576));
#76775=CARTESIAN_POINT('Ctrl Pts',(-6.6494231153614,-2.23116660581882,10.8765840723814));
#76776=CARTESIAN_POINT('Ctrl Pts',(-6.58721713263291,-2.4086301375784,10.8851131045052));
#76777=CARTESIAN_POINT('Ctrl Pts',(-6.51798943486467,-2.583300270873,10.893642136629));
#76778=CARTESIAN_POINT('Ctrl Pts',(-6.44876104463667,-2.75797215133014,
10.9021712540656));
#76779=CARTESIAN_POINT('Ctrl Pts',(-6.37251091485545,-2.92985029402879,
10.9107003715023));
#76780=CARTESIAN_POINT('Ctrl Pts',(-6.28949269640831,-3.09837186023992,
10.9192294889389));
#76781=CARTESIAN_POINT('Ctrl Pts',(-6.20645768023238,-3.26692752474438,
10.927760332139));
#76782=CARTESIAN_POINT('Ctrl Pts',(-6.11665197635673,-3.43212498199062,
10.936291175339));
#76783=CARTESIAN_POINT('Ctrl Pts',(-6.02037580528256,-3.59342479059579,
10.944822018539));
#76784=CARTESIAN_POINT('Ctrl Pts',(-6.00554384178086,-3.61827406375831,
10.9461362498132));
#76785=CARTESIAN_POINT('Ctrl Pts',(-5.99055839931713,-3.64303088294956,
10.9474504810873));
#76786=CARTESIAN_POINT('Ctrl Pts',(-5.97542066998606,-3.66769333221895,
10.9487647123615));
#76787=CARTESIAN_POINT('Ctrl Pts',(-5.87715876445461,-3.8277820223575,10.9572956397208));
#76788=CARTESIAN_POINT('Ctrl Pts',(-5.77244288573805,-3.98394701045112,
10.96582656708));
#76789=CARTESIAN_POINT('Ctrl Pts',(-5.66161140464517,-4.13567199682128,
10.9743574944393));
#76790=CARTESIAN_POINT('Ctrl Pts',(-5.55080096476639,-4.28736817839798,
10.982886802213));
#76791=CARTESIAN_POINT('Ctrl Pts',(-5.43387742002723,-4.43462579325325,
10.9914161099866));
#76792=CARTESIAN_POINT('Ctrl Pts',(-5.31122151291524,-4.57695888153328,
10.9999454177603));
#76793=CARTESIAN_POINT('Ctrl Pts',(-5.1822607017228,-4.72660834364486,11.0089131591052));
#76794=CARTESIAN_POINT('Ctrl Pts',(-5.04696290758847,-4.87081338721959,
11.0178809004501));
#76795=CARTESIAN_POINT('Ctrl Pts',(-4.90581801919283,-5.00904942330009,
11.026848641795));
#76796=CARTESIAN_POINT('Ctrl Pts',(-4.7715780538619,-5.14052283974373,11.0353776739188));
#76797=CARTESIAN_POINT('Ctrl Pts',(-4.63204964690216,-5.2665970759815,11.0439067060426));
#76798=CARTESIAN_POINT('Ctrl Pts',(-4.48769173061396,-5.38685896357786,
11.0524357381664));
#76799=CARTESIAN_POINT('Ctrl Pts',(-4.34333237036528,-5.50712205411076,
11.060964855603));
#76800=CARTESIAN_POINT('Ctrl Pts',(-4.19414364159007,-5.62157248633174,
11.0694939730396));
#76801=CARTESIAN_POINT('Ctrl Pts',(-4.04061756016206,-5.72983737072965,
11.0780230904763));
#76802=CARTESIAN_POINT('Ctrl Pts',(-3.88706041459529,-5.83812416121257,
11.0865539336763));
#76803=CARTESIAN_POINT('Ctrl Pts',(-3.729164414304,-5.94022272839675,11.0950847768763));
#76804=CARTESIAN_POINT('Ctrl Pts',(-3.56745127519244,-6.03580300884877,
11.1036156200763));
#76805=CARTESIAN_POINT('Ctrl Pts',(-3.54253832580481,-6.05052776592441,
11.1049298513505));
#76806=CARTESIAN_POINT('Ctrl Pts',(-3.517534835176,-6.06509790795472,11.1062440826248));
#76807=CARTESIAN_POINT('Ctrl Pts',(-3.49244276676198,-6.0795123228259,11.107558313899));
#76808=CARTESIAN_POINT('Ctrl Pts',(-3.32956533633588,-6.17307905541145,
11.1160892412583));
#76809=CARTESIAN_POINT('Ctrl Pts',(-3.16289771561957,-6.26011251430186,
11.1246201686175));
#76810=CARTESIAN_POINT('Ctrl Pts',(-2.99298404964067,-6.34032120961522,
11.1331510959768));
#76811=CARTESIAN_POINT('Ctrl Pts',(-2.82310264155287,-6.42051467741086,
11.1416804037504));
#76812=CARTESIAN_POINT('Ctrl Pts',(-2.64997669479013,-6.49388583662647,
11.1502097115241));
#76813=CARTESIAN_POINT('Ctrl Pts',(-2.47417304661047,-6.56019011141646,
11.1587390192978));
#76814=CARTESIAN_POINT('Ctrl Pts',(-2.28933253127214,-6.62990263699949,
11.1677067606427));
#76815=CARTESIAN_POINT('Ctrl Pts',(-2.10153211272916,-6.6918024793668,11.1766745019876));
#76816=CARTESIAN_POINT('Ctrl Pts',(-1.91145295365878,-6.74566336014844,
11.1856422433325));
#76817=CARTESIAN_POINT('Ctrl Pts',(-1.73067262208771,-6.79688932271075,
11.1941712754562));
#76818=CARTESIAN_POINT('Ctrl Pts',(-1.54783149561706,-6.84084397960362,
11.20270030758));
#76819=CARTESIAN_POINT('Ctrl Pts',(-1.36353024650465,-6.87738408331009,
11.2112293397038));
#76820=CARTESIAN_POINT('Ctrl Pts',(-1.17922715389277,-6.91392455251415,
11.2197584571405));
#76821=CARTESIAN_POINT('Ctrl Pts',(-0.993464210436353,-6.94305026396572,
11.2282875745771));
#76822=CARTESIAN_POINT('Ctrl Pts',(-0.806851869341063,-6.96466916826929,
11.2368166920138));
#76823=CARTESIAN_POINT('Ctrl Pts',(-0.620201769504061,-6.98629244689569,
11.2453475352138));
#76824=CARTESIAN_POINT('Ctrl Pts',(-0.432702233044765,-7.00040585033402,
11.2538783784138));
#76825=CARTESIAN_POINT('Ctrl Pts',(-0.244969304306911,-7.00696914524728,
11.2624092216138));
#76826=CARTESIAN_POINT('Ctrl Pts',(-0.216047838940853,-7.00798026305063,
11.263723452888));
#76827=CARTESIAN_POINT('Ctrl Pts',(-0.187120839258501,-7.00881229177017,
11.2650376841623));
#76828=CARTESIAN_POINT('Ctrl Pts',(-0.158190561489543,-7.00946519420388,
11.2663519154365));
#76829=CARTESIAN_POINT('Ctrl Pts',(0.0296014222860561,-7.0137033091718,
11.2748828427958));
#76830=CARTESIAN_POINT('Ctrl Pts',(0.217595963931144,-7.01039104812785,
11.283413770155));
#76831=CARTESIAN_POINT('Ctrl Pts',(0.4051757782064,-6.9995327809258,11.2919446975143));
#76832=CARTESIAN_POINT('Ctrl Pts',(0.592719980695167,-6.98867657515181,
11.300474005288));
#76833=CARTESIAN_POINT('Ctrl Pts',(0.77984930738174,-6.97027723981227,11.3090033130616));
#76834=CARTESIAN_POINT('Ctrl Pts',(0.965948991419823,-6.94439119782829,
11.3175326208353));
#76835=CARTESIAN_POINT('Ctrl Pts',(1.16161479163565,-6.91717453088232,11.3265003621802));
#76836=CARTESIAN_POINT('Ctrl Pts',(1.35614194622031,-6.88168123828715,11.3354681035251));
#76837=CARTESIAN_POINT('Ctrl Pts',(1.5488240502208,-6.83803850705432,11.34443584487));
#76838=CARTESIAN_POINT('Ctrl Pts',(1.73207998853247,-6.79653081383059,11.3529648769938));
#76839=CARTESIAN_POINT('Ctrl Pts',(1.91366676134555,-6.74765205227895,11.3614939091175));
#76840=CARTESIAN_POINT('Ctrl Pts',(2.09298836882461,-6.69156381202966,11.3700229412413));
#76841=CARTESIAN_POINT('Ctrl Pts',(2.27231176999349,-6.63547501074978,11.3785520586779));
#76842=CARTESIAN_POINT('Ctrl Pts',(2.44936966928575,-6.57217668117308,11.3870811761146));
#76843=CARTESIAN_POINT('Ctrl Pts',(2.62358197262553,-6.50188005083256,11.3956102935512));
#76844=CARTESIAN_POINT('Ctrl Pts',(2.79782952570986,-6.43156919682232,11.4041411367512));
#76845=CARTESIAN_POINT('Ctrl Pts',(2.96923004923471,-6.35425732927099,11.4126719799512));
#76846=CARTESIAN_POINT('Ctrl Pts',(3.13722332970476,-6.27020385171457,11.4212028231512));
#76847=CARTESIAN_POINT('Ctrl Pts',(3.16310377527063,-6.25725487277663,11.4225170544255));
#76848=CARTESIAN_POINT('Ctrl Pts',(3.18890339925198,-6.24414598323843,11.4238312856998));
#76849=CARTESIAN_POINT('Ctrl Pts',(3.2146202025958,-6.23087822987763,11.4251455169741));
#76850=CARTESIAN_POINT('Ctrl Pts',(3.38155290730832,-6.14475469716764,11.4336764443334));
#76851=CARTESIAN_POINT('Ctrl Pts',(3.54505116448901,-6.05190407164105,11.4422073716927));
#76852=CARTESIAN_POINT('Ctrl Pts',(3.7045750104399,-5.95262551774629,11.4507382990519));
#76853=CARTESIAN_POINT('Ctrl Pts',(3.86406857099377,-5.85336581175731,11.4592676068256));
#76854=CARTESIAN_POINT('Ctrl Pts',(4.0195889662208,-5.74768077442588,11.4677969145993));
#76855=CARTESIAN_POINT('Ctrl Pts',(4.17062334758744,-5.63591407449213,11.476326222373));
#76856=CARTESIAN_POINT('Ctrl Pts',(4.3294213769491,-5.51840221039114,11.4852939637179));
#76857=CARTESIAN_POINT('Ctrl Pts',(4.48325975390525,-5.39416718527567,11.4942617050628));
#76858=CARTESIAN_POINT('Ctrl Pts',(4.63157901569038,-5.26365865001869,11.5032294464077));
#76859=CARTESIAN_POINT('Ctrl Pts',(4.77264237821296,-5.13953469875525,11.5117584785314));
#76860=CARTESIAN_POINT('Ctrl Pts',(4.90871346980811,-5.00973659621219,11.5202875106552));
#76861=CARTESIAN_POINT('Ctrl Pts',(5.03934623655124,-4.87469138209352,11.528816542779));
#76862=CARTESIAN_POINT('Ctrl Pts',(5.16998030996718,-4.73964481716591,11.5373456602157));
#76863=CARTESIAN_POINT('Ctrl Pts',(5.29517573927452,-4.5993512581201,11.5458747776523));
#76864=CARTESIAN_POINT('Ctrl Pts',(5.41452418602606,-4.45427372322794,11.554403895089));
#76865=CARTESIAN_POINT('Ctrl Pts',(5.53389678148686,-4.30916683365789,11.562934738289));
#76866=CARTESIAN_POINT('Ctrl Pts',(5.6474198376326,-4.15927427195977,11.571465581489));
#76867=CARTESIAN_POINT('Ctrl Pts',(5.75472552247272,-4.00509184957113,11.579996424689));
#76868=CARTESIAN_POINT('Ctrl Pts',(5.77125665352394,-3.9813390555407,11.5813106559632));
#76869=CARTESIAN_POINT('Ctrl Pts',(5.78764030715153,-3.95748450720761,11.5826248872374));
#76870=CARTESIAN_POINT('Ctrl Pts',(5.80387522874341,-3.93353008017972,11.5839391185116));
#76871=CARTESIAN_POINT('Ctrl Pts',(5.90925921975167,-3.77803729826333,11.5924700458709));
#76872=CARTESIAN_POINT('Ctrl Pts',(6.00840889593352,-3.61828041899149,11.6010009732301));
#76873=CARTESIAN_POINT('Ctrl Pts',(6.10099322995065,-3.45478048081153,11.6095319005894));
#76874=CARTESIAN_POINT('Ctrl Pts',(6.19355998695104,-3.29131158288457,11.618061208363));
#76875=CARTESIAN_POINT('Ctrl Pts',(6.27956373833922,-3.12410131048978,11.6265905161367));
#76876=CARTESIAN_POINT('Ctrl Pts',(6.35871855945826,-2.95369680977941,11.6351198239104));
#76877=CARTESIAN_POINT('Ctrl Pts',(6.44194219035925,-2.77453297527768,11.6440875652553));
#76878=CARTESIAN_POINT('Ctrl Pts',(6.51759406510952,-2.59183819829493,11.6530553066002));
#76879=CARTESIAN_POINT('Ctrl Pts',(6.58539803079892,-2.40627499227535,11.6620230479451));
#76880=CARTESIAN_POINT('Ctrl Pts',(6.64988497118259,-2.22978968964862,11.6705520800688));
#76881=CARTESIAN_POINT('Ctrl Pts',(6.70727338892337,-2.05071021315633,11.6790811121926));
#76882=CARTESIAN_POINT('Ctrl Pts',(6.75737590055037,-1.86962496270269,11.6876101443164));
#76883=CARTESIAN_POINT('Ctrl Pts',(6.80747891333487,-1.68853790091811,11.696139261753));
#76884=CARTESIAN_POINT('Ctrl Pts',(6.85029579585306,-1.50544532105624,11.7046683791897));
#76885=CARTESIAN_POINT('Ctrl Pts',(6.88568949677476,-1.32094917256713,11.7131974966263));
#76886=CARTESIAN_POINT('Ctrl Pts',(6.92109035918214,-1.13641569352227,11.7217283398263));
#76887=CARTESIAN_POINT('Ctrl Pts',(6.94906498328526,-0.950478379528501,
11.7302591830263));
#76888=CARTESIAN_POINT('Ctrl Pts',(6.96952757673796,-0.76374859711106,11.7387900262263));
#76889=CARTESIAN_POINT('Ctrl Pts',(6.97267997089618,-0.734981672888097,
11.7401042575005));
#76890=CARTESIAN_POINT('Ctrl Pts',(6.97565417904955,-0.706195953020086,
11.7414184887748));
#76891=CARTESIAN_POINT('Ctrl Pts',(6.97844999683549,-0.677393684770329,
11.7427327200491));
#76892=CARTESIAN_POINT('Ctrl Pts',(6.99659818650985,-0.490432635349663,
11.7512636474084));
#76893=CARTESIAN_POINT('Ctrl Pts',(7.0072317929105,-0.302709847237606,11.7597945747676));
#76894=CARTESIAN_POINT('Ctrl Pts',(7.01030941215522,-0.114841231045246,
11.7683255021269));
#76895=CARTESIAN_POINT('Ctrl Pts',(7.01338644711788,0.0729917185319949,
11.7768548099006));
#76896=CARTESIAN_POINT('Ctrl Pts',(7.00891035259778,0.260970134912832,11.7853841176742));
#76897=CARTESIAN_POINT('Ctrl Pts',(6.99689182124385,0.448476760056742,11.7939134254479));
#76898=CARTESIAN_POINT('Ctrl Pts',(6.9842554991193,0.645621822629625,11.8028811667928));
#76899=CARTESIAN_POINT('Ctrl Pts',(6.96328091396697,0.842244950637739,11.8118489081377));
#76900=CARTESIAN_POINT('Ctrl Pts',(6.93404253432215,1.03763225408199,11.8208166494826));
#76901=CARTESIAN_POINT('Ctrl Pts',(6.90623452005778,1.22346105127444,11.8293456816064));
#76902=CARTESIAN_POINT('Ctrl Pts',(6.870951978804,1.40817172144332,11.8378747137301));
#76903=CARTESIAN_POINT('Ctrl Pts',(6.82831187180202,1.5911579255082,11.8464037458539));
#76904=CARTESIAN_POINT('Ctrl Pts',(6.78567133828632,1.77414595991857,11.8549328632905));
#76905=CARTESIAN_POINT('Ctrl Pts',(6.73567316461057,1.95540919628536,11.8634619807272));
#76906=CARTESIAN_POINT('Ctrl Pts',(6.67848499248496,2.13435347767263,11.8719910981638));
#76907=CARTESIAN_POINT('Ctrl Pts',(6.62128524902705,2.31333396626264,11.8805219413638));
#76908=CARTESIAN_POINT('Ctrl Pts',(6.556892695528,2.48999427131952,11.8890527845638));
#76909=CARTESIAN_POINT('Ctrl Pts',(6.48552449095859,2.66375649031145,11.8975836277638));
#76910=CARTESIAN_POINT('Ctrl Pts',(6.47452975992965,2.69052567796768,11.8988978590381));
#76911=CARTESIAN_POINT('Ctrl Pts',(6.46336956671342,2.71722612121925,11.9002120903123));
#76912=CARTESIAN_POINT('Ctrl Pts',(6.4520448070097,2.74385574891231,11.9015263215866));
#76913=CARTESIAN_POINT('Ctrl Pts',(6.37853361892237,2.91671377162142,11.9100572489459));
#76914=CARTESIAN_POINT('Ctrl Pts',(6.29805924023454,3.08664550243246,11.9185881763051));
#76915=CARTESIAN_POINT('Ctrl Pts',(6.21087998261419,3.25309028526145,11.9271191036644));
#76916=CARTESIAN_POINT('Ctrl Pts',(6.12371727586372,3.41950346876258,11.935648411438));
#76917=CARTESIAN_POINT('Ctrl Pts',(6.02985237242374,3.58243075422884,11.9441777192117));
#76918=CARTESIAN_POINT('Ctrl Pts',(5.92958997594226,3.74133522685486,11.9527070269854));
#76919=CARTESIAN_POINT('Ctrl Pts',(5.82417377311273,3.90840789522019,11.9616747683303));
#76920=CARTESIAN_POINT('Ctrl Pts',(5.7116852314054,4.07103297223653,11.9706425096752));
#76921=CARTESIAN_POINT('Ctrl Pts',(5.59253128927933,4.22861920027468,11.9796102510201));
#76922=CARTESIAN_POINT('Ctrl Pts',(5.4792064551898,4.37849618150225,11.9881392831438));
#76923=CARTESIAN_POINT('Ctrl Pts',(5.35985298726444,4.52381527551863,11.9966683152676));
#76924=CARTESIAN_POINT('Ctrl Pts',(5.23486368244281,4.66409999772103,12.0051973473914));
#76925=CARTESIAN_POINT('Ctrl Pts',(5.10987312739806,4.80438612314112,12.013726464828));
#76926=CARTESIAN_POINT('Ctrl Pts',(4.97924682892356,4.9396375496616,12.0222555822646));
#76927=CARTESIAN_POINT('Ctrl Pts',(4.84341625951693,5.06941273714688,12.0307846997013));
#76928=CARTESIAN_POINT('Ctrl Pts',(4.70755820644357,5.19921418306587,12.0393155429012));
#76929=CARTESIAN_POINT('Ctrl Pts',(4.56649400128168,5.32353696597768,12.0478463861012));
#76930=CARTESIAN_POINT('Ctrl Pts',(4.42069082235599,5.44197750965929,12.0563772293012));
#76931=CARTESIAN_POINT('Ctrl Pts',(4.39822890468348,5.46022403734727,12.0576914605755));
#76932=CARTESIAN_POINT('Ctrl Pts',(4.37565457964087,5.47833103685979,12.0590056918498));
#76933=CARTESIAN_POINT('Ctrl Pts',(4.35296962466576,5.49629711799109,12.0603199231241));
#76934=CARTESIAN_POINT('Ctrl Pts',(4.20571722942396,5.61291839771571,12.0688508504834));
#76935=CARTESIAN_POINT('Ctrl Pts',(4.0537502967726,5.72363863137833,12.0773817778426));
#76936=CARTESIAN_POINT('Ctrl Pts',(3.89756389109848,5.82808907595837,12.0859127052019));
#76937=CARTESIAN_POINT('Ctrl Pts',(3.74140713721253,5.93251969075589,12.0944420129756));
#76938=CARTESIAN_POINT('Ctrl Pts',(3.5810327633266,6.03068272171986,12.1029713207493));
#76939=CARTESIAN_POINT('Ctrl Pts',(3.41696521332584,6.1222524689383,12.111500628523));
#76940=CARTESIAN_POINT('Ctrl Pts',(3.24446406897338,6.21852919266078,12.1204683698679));
#76941=CARTESIAN_POINT('Ctrl Pts',(3.06788037503395,6.30751675766089,12.1294361112128));
#76942=CARTESIAN_POINT('Ctrl Pts',(2.88785434964569,6.38889065626674,12.1384038525576));
#76943=CARTESIAN_POINT('Ctrl Pts',(2.71663534425694,6.46628367738049,12.1469328846814));
#76944=CARTESIAN_POINT('Ctrl Pts',(2.54230306279958,6.53679002485036,12.1554619168052));
#76945=CARTESIAN_POINT('Ctrl Pts',(2.36543039462724,6.60017921049676,12.163990948929));
#76946=CARTESIAN_POINT('Ctrl Pts',(2.18855595726061,6.6635690302026,12.1725200663657));
#76947=CARTESIAN_POINT('Ctrl Pts',(2.00914137174163,6.71984144557955,12.1810491838023));
#76948=CARTESIAN_POINT('Ctrl Pts',(1.8277767709993,6.76881515761033,12.189578301239));
#76949=CARTESIAN_POINT('Ctrl Pts',(1.64637547333213,6.81779877887711,12.198109144439));
#76950=CARTESIAN_POINT('Ctrl Pts',(1.46302366824735,6.85948066824455,12.206639987639));
#76951=CARTESIAN_POINT('Ctrl Pts',(1.27832467986038,6.89372994650645,12.215170830839));
#76952=CARTESIAN_POINT('Ctrl Pts',(1.24987061252392,6.89900626814958,12.2164850621132));
#76953=CARTESIAN_POINT('Ctrl Pts',(1.22138459165351,6.90410628749476,12.2177992933874));
#76954=CARTESIAN_POINT('Ctrl Pts',(1.1928688431785,6.90902963414357,12.2191135246616));
#76955=CARTESIAN_POINT('Ctrl Pts',(1.00776764857753,6.94098802187192,12.2276444520209));
#76956=CARTESIAN_POINT('Ctrl Pts',(0.821349726612002,6.96550897478315,12.2361753793801));
#76957=CARTESIAN_POINT('Ctrl Pts',(0.634226223665535,6.98250554312096,12.2447063067394));
#76958=CARTESIAN_POINT('Ctrl Pts',(0.44713824587523,6.99949888468215,12.2532356145131));
#76959=CARTESIAN_POINT('Ctrl Pts',(0.259345259236782,7.0089706646968,12.2617649222868));
#76960=CARTESIAN_POINT('Ctrl Pts',(0.071463615970264,7.01088578669575,12.2702942300605));
#76961=CARTESIAN_POINT('Ctrl Pts',(-0.126075741850434,7.01289935206193,
12.2792619714054));
#76962=CARTESIAN_POINT('Ctrl Pts',(-0.323712748584714,7.00655890577502,
12.2882297127503));
#76963=CARTESIAN_POINT('Ctrl Pts',(-0.520729958005908,6.99188578806428,
12.2971974540951));
#76964=CARTESIAN_POINT('Ctrl Pts',(-0.70810892484529,6.97793049124006,12.3057264862189));
#76965=CARTESIAN_POINT('Ctrl Pts',(-0.894926956630577,6.95643834403778,
12.3142555183427));
#76966=CARTESIAN_POINT('Ctrl Pts',(-1.08057071195963,6.9274810356258,12.3227845504665));
#76967=CARTESIAN_POINT('Ctrl Pts',(-1.26621632421679,6.89852343756421,12.3313136679031));
#76968=CARTESIAN_POINT('Ctrl Pts',(-1.45068733450797,6.86210057947786,12.3398427853397));
#76969=CARTESIAN_POINT('Ctrl Pts',(-1.63337879291733,6.81833559465563,12.3483719027764));
#76970=CARTESIAN_POINT('Ctrl Pts',(-1.81610721672529,6.77456175452006,12.3569027459764));
#76971=CARTESIAN_POINT('Ctrl Pts',(-1.99705507191243,6.7234428927166,12.3654335891764));
#76972=CARTESIAN_POINT('Ctrl Pts',(-2.17562994733623,6.66515272853922,12.3739644323764));
#76973=CARTESIAN_POINT('Ctrl Pts',(-2.20314055567612,6.65617275376423,12.3752786636506));
#76974=CARTESIAN_POINT('Ctrl Pts',(-2.2305948751188,6.64702267581864,12.3765928949249));
#76975=CARTESIAN_POINT('Ctrl Pts',(-2.25799077380797,6.63770323439502,12.3779071261992));
#76976=CARTESIAN_POINT('Ctrl Pts',(-2.43582280857313,6.57720895201938,12.3864380535585));
#76977=CARTESIAN_POINT('Ctrl Pts',(-2.61125281161355,6.50955370244616,12.3949689809177));
#76978=CARTESIAN_POINT('Ctrl Pts',(-2.783702519971,6.4349535229718,12.403499908277));
#76979=CARTESIAN_POINT('Ctrl Pts',(-2.95611948897335,6.36036750624545,12.4120292160506));
#76980=CARTESIAN_POINT('Ctrl Pts',(-3.12555701150585,6.27883931231684,12.4205585238243));
#76981=CARTESIAN_POINT('Ctrl Pts',(-3.29145706134546,6.19063300283736,12.429087831598));
#76982=CARTESIAN_POINT('Ctrl Pts',(-3.46588490186243,6.09789260826032,12.4380555729429));
#76983=CARTESIAN_POINT('Ctrl Pts',(-3.63640168893796,5.99776961881503,12.4470233142878));
#76984=CARTESIAN_POINT('Ctrl Pts',(-3.80238762400336,5.89062602100372,12.4559910556327));
#76985=CARTESIAN_POINT('Ctrl Pts',(-3.96025339173896,5.78872397538899,12.4645200877564));
#76986=CARTESIAN_POINT('Ctrl Pts',(-4.11402073983235,5.68047199133421,12.4730491198802));
#76987=CARTESIAN_POINT('Ctrl Pts',(-4.26318537528538,5.5662264612979,12.481578152004));
#76988=CARTESIAN_POINT('Ctrl Pts',(-4.41235150277912,5.45197978850424,12.4901072694406));
#76989=CARTESIAN_POINT('Ctrl Pts',(-4.55691458451787,5.33173963869023,12.4986363868772));
#76990=CARTESIAN_POINT('Ctrl Pts',(-4.69640230864733,5.20590356401576,12.5071655043139));
#76991=CARTESIAN_POINT('Ctrl Pts',(-4.83591825642416,5.08004202793945,12.5156963475138));
#76992=CARTESIAN_POINT('Ctrl Pts',(-4.97035656874706,4.94858251132437,12.5242271907138));
#76993=CARTESIAN_POINT('Ctrl Pts',(-5.09928014619986,4.81196098831567,12.5327580339138));
#76994=CARTESIAN_POINT('Ctrl Pts',(-5.11914165267813,4.79091356380326,12.5340722651881));
#76995=CARTESIAN_POINT('Ctrl Pts',(-5.13887234810774,4.76974369747548,12.5353864964624));
#76996=CARTESIAN_POINT('Ctrl Pts',(-5.15847071434015,4.74845305881768,12.5367007277367));
#76997=CARTESIAN_POINT('Ctrl Pts',(-5.28568623754314,4.6102527770157,12.5452315724605));
#76998=CARTESIAN_POINT('Ctrl Pts',(-5.40736656653399,4.46691356332463,12.5537624171842));
#76999=CARTESIAN_POINT('Ctrl Pts',(-5.52310728351011,4.31890176981807,12.562293261908));
#77000=CARTESIAN_POINT('Ctrl Pts',(-5.63883447817802,4.17090726893886,12.5708231099496));
#77001=CARTESIAN_POINT('Ctrl Pts',(-5.74862325482246,4.01824151702849,12.5793529579912));
#77002=CARTESIAN_POINT('Ctrl Pts',(-5.85210986254844,3.86140346495459,12.5878828060328));
#77003=CARTESIAN_POINT('Ctrl Pts',(-5.95558215690717,3.70458710535557,12.5964114743));
#77004=CARTESIAN_POINT('Ctrl Pts',(-6.0527538545703,3.54359985365895,12.6049401425672));
#77005=CARTESIAN_POINT('Ctrl Pts',(-6.14330460870189,3.37896952445596,12.6134688108344));
#77006=CARTESIAN_POINT('Ctrl Pts',(-6.23386368139959,3.21432407126764,12.6219982625991));
#77007=CARTESIAN_POINT('Ctrl Pts',(-6.31780044538522,3.04603513900085,12.6305277143639));
#77008=CARTESIAN_POINT('Ctrl Pts',(-6.3948401306816,2.87465585166714,12.6390571661286));
#77009=CARTESIAN_POINT('Ctrl Pts',(-6.45877643285204,2.732425806742,12.6461358763191));
#77010=CARTESIAN_POINT('Ctrl Pts',(-6.51796310877441,2.5880677856993,12.6532145865095));
#77011=CARTESIAN_POINT('Ctrl Pts',(-6.57226799596304,2.44190907933526,12.6602932967));
#77012=CARTESIAN_POINT('Origin',(0.,0.,10.));
#77013=CARTESIAN_POINT('',(-6.57184683924635,2.44175302781609,14.6603043765569));
#77014=CARTESIAN_POINT('',(-6.57226804984416,2.4419089343171,14.1134456015891));
#77015=CARTESIAN_POINT('',(-6.57226799596304,2.44190907933527,10.));
#77016=CARTESIAN_POINT('Ctrl Pts',(-6.57226804984416,2.44190893431709,14.1134456015891));
#77017=CARTESIAN_POINT('Ctrl Pts',(-6.48988173044915,2.66364733213147,14.1025828518473));
#77018=CARTESIAN_POINT('Ctrl Pts',(-6.39630361412272,2.88113588408464,14.0916770028235));
#77019=CARTESIAN_POINT('Ctrl Pts',(-6.20477826197012,3.270675629613,14.0717600846099));
#77020=CARTESIAN_POINT('Ctrl Pts',(-6.11023863081956,3.44406416570828,14.0627446265518));
#77021=CARTESIAN_POINT('Ctrl Pts',(-5.80031227068627,3.9594459635228,14.035439112705));
#77022=CARTESIAN_POINT('Ctrl Pts',(-5.56258254002533,4.2870170627201,14.0174075629248));
#77023=CARTESIAN_POINT('Ctrl Pts',(-5.17403817579258,4.73526728233403,13.9908142506871));
#77024=CARTESIAN_POINT('Ctrl Pts',(-5.04437180995973,4.87316514332628,13.9823164042756));
#77025=CARTESIAN_POINT('Ctrl Pts',(-4.72658268366533,5.18483684998203,13.9620929363086));
#77026=CARTESIAN_POINT('Ctrl Pts',(-4.53420453237304,5.35388677028809,13.9503106104565));
#77027=CARTESIAN_POINT('Ctrl Pts',(-4.09882958945337,5.69613542265287,13.924829527098));
#77028=CARTESIAN_POINT('Ctrl Pts',(-3.85314222011895,5.86512258394285,13.9111641428651));
#77029=CARTESIAN_POINT('Ctrl Pts',(-3.38651301337097,6.14406628020359,13.8864515842056));
#77030=CARTESIAN_POINT('Ctrl Pts',(-3.16909023227608,6.25898481690349,13.8753782590726));
#77031=CARTESIAN_POINT('Ctrl Pts',(-2.73841179111228,6.45841318393376,13.8540790468738));
#77032=CARTESIAN_POINT('Ctrl Pts',(-2.52616017117184,6.54434979977739,13.843858869066));
#77033=CARTESIAN_POINT('Ctrl Pts',(-2.16646658765174,6.66987166256495,13.8267472874566));
#77034=CARTESIAN_POINT('Ctrl Pts',(-2.02125552842448,6.71530274275546,13.8198910068932));
#77035=CARTESIAN_POINT('Ctrl Pts',(-1.63487962710397,6.822516228019,13.8016439752891));
#77036=CARTESIAN_POINT('Ctrl Pts',(-1.3917075404866,6.87624221271912,13.7901835469605));
#77037=CARTESIAN_POINT('Ctrl Pts',(-0.840175372970261,6.96763611611037,
13.7644616339783));
#77038=CARTESIAN_POINT('Ctrl Pts',(-0.531120257163189,6.99798292517838,
13.7502416090816));
#77039=CARTESIAN_POINT('Ctrl Pts',(0.181645536548465,7.02046808966678,13.7178637521637));
#77040=CARTESIAN_POINT('Ctrl Pts',(0.584707402117657,6.99843479598702,13.6998792989317));
#77041=CARTESIAN_POINT('Ctrl Pts',(1.17163332084612,6.91526944372014,13.6733053088329));
#77042=CARTESIAN_POINT('Ctrl Pts',(1.35846081373189,6.88100708483956,13.6647784087037));
#77043=CARTESIAN_POINT('Ctrl Pts',(1.79384769552674,6.78273672186202,13.6444997429995));
#77044=CARTESIAN_POINT('Ctrl Pts',(2.04074158588925,6.71258355814904,13.6326911383502));
#77045=CARTESIAN_POINT('Ctrl Pts',(2.56460529817627,6.53215039256923,13.6071974954196));
#77046=CARTESIAN_POINT('Ctrl Pts',(2.83952635221048,6.41742037794411,13.5935457310602));
#77047=CARTESIAN_POINT('Ctrl Pts',(3.32676001282588,6.17662955546867,13.5688407075346));
#77048=CARTESIAN_POINT('Ctrl Pts',(3.5413121731163,6.05617007167114,13.5577616718927));
#77049=CARTESIAN_POINT('Ctrl Pts',(3.94207716266246,5.80256919672595,13.5364782323738));
#77050=CARTESIAN_POINT('Ctrl Pts',(4.12897741638742,5.67109571939389,13.5262792566597));
#77051=CARTESIAN_POINT('Ctrl Pts',(4.42922490054694,5.43716583396649,13.5091833949684));
#77052=CARTESIAN_POINT('Ctrl Pts',(4.54624057387714,5.33970987365993,13.5023213004557));
#77053=CARTESIAN_POINT('Ctrl Pts',(4.84620827224397,5.07286991086351,13.4840515739854));
#77054=CARTESIAN_POINT('Ctrl Pts',(5.02345829493919,4.89740832209359,13.4725739360711));
#77055=CARTESIAN_POINT('Ctrl Pts',(5.39795781404628,4.48491737642743,13.4469403718156));
#77056=CARTESIAN_POINT('Ctrl Pts',(5.58968999466384,4.24356030890051,13.4328247814249));
#77057=CARTESIAN_POINT('Ctrl Pts',(5.99858913327381,3.65282013906985,13.4002009206419));
#77058=CARTESIAN_POINT('Ctrl Pts',(6.20214284058919,3.29539007315769,13.3818826938069));
#77059=CARTESIAN_POINT('Ctrl Pts',(6.45048723142797,2.75375762287443,13.3551672738472));
#77060=CARTESIAN_POINT('Ctrl Pts',(6.5210129851148,2.58231573513183,13.3468420622052));
#77061=CARTESIAN_POINT('Ctrl Pts',(6.67134828613846,2.17127315620059,13.326954777041));
#77062=CARTESIAN_POINT('Ctrl Pts',(6.74517234014827,1.92975711192974,13.3153370480986));
#77063=CARTESIAN_POINT('Ctrl Pts',(6.8756245571424,1.40278755445331,13.2903578840909));
#77064=CARTESIAN_POINT('Ctrl Pts',(6.92784099962088,1.11671380222594,13.2770266146276));
#77065=CARTESIAN_POINT('Ctrl Pts',(6.99018049632219,0.592679883307333,13.2530232141164));
#77066=CARTESIAN_POINT('Ctrl Pts',(7.00622988329145,0.355862965151497,13.2423242106312));
#77067=CARTESIAN_POINT('Ctrl Pts',(7.01457524698399,-0.137060179496263,
13.2201855464205));
#77068=CARTESIAN_POINT('Ctrl Pts',(7.00490678516095,-0.392850657460589,
13.2087707119927));
#77069=CARTESIAN_POINT('Ctrl Pts',(6.97473271599155,-0.718165076226803,
13.1940898122617));
#77070=CARTESIAN_POINT('Ctrl Pts',(6.9671105582604,-0.788687455659186,13.1908968216263));
#77071=CARTESIAN_POINT('Ctrl Pts',(6.94282124280033,-0.985426909372901,
13.1819446345389));
#77072=CARTESIAN_POINT('Ctrl Pts',(6.92378495850714,-1.11132076662028,13.1761573600352));
#77073=CARTESIAN_POINT('Ctrl Pts',(6.85264042021602,-1.50836258796409,13.1577099118988));
#77074=CARTESIAN_POINT('Ctrl Pts',(6.78794220051204,-1.77698582695205,13.1449735971886));
#77075=CARTESIAN_POINT('Ctrl Pts',(6.63373968894409,-2.28373638118698,13.120643079893));
#77076=CARTESIAN_POINT('Ctrl Pts',(6.54679125341049,-2.52219786746139,13.1090568645139));
#77077=CARTESIAN_POINT('Ctrl Pts',(6.33139713751134,-3.02617441237579,13.0842104105928));
#77078=CARTESIAN_POINT('Ctrl Pts',(6.19874104588227,-3.2893668581869,13.07100892477));
#77079=CARTESIAN_POINT('Ctrl Pts',(5.92623914614782,-3.75462576597372,13.0468571513832));
#77080=CARTESIAN_POINT('Ctrl Pts',(5.7915769575567,-3.95918656590113,13.0359157636759));
#77081=CARTESIAN_POINT('Ctrl Pts',(5.56187415965321,-4.27124809640272,13.0183664630607));
#77082=CARTESIAN_POINT('Ctrl Pts',(5.47376146129888,-4.3835987796216,13.0118464496891));
#77083=CARTESIAN_POINT('Ctrl Pts',(5.1957290971398,-4.71664776684635,12.9919466769759));
#77084=CARTESIAN_POINT('Ctrl Pts',(4.99543886527827,-4.92828153788388,12.9785181364631));
#77085=CARTESIAN_POINT('Ctrl Pts',(4.70567971801063,-5.19858278208314,12.9603589361663));
#77086=CARTESIAN_POINT('Ctrl Pts',(4.62718110597341,-5.26857474276685,12.955552163469));
#77087=CARTESIAN_POINT('Ctrl Pts',(4.37862847841751,-5.48035114091313,12.9406705061009));
#77088=CARTESIAN_POINT('Ctrl Pts',(4.20341205452278,-5.6158673035093,12.9306568739139));
#77089=CARTESIAN_POINT('Ctrl Pts',(3.78284448264097,-5.91041608574044,12.9075512508823));
#77090=CARTESIAN_POINT('Ctrl Pts',(3.53337802338744,-6.0628516570412,12.8945251024392));
#77091=CARTESIAN_POINT('Ctrl Pts',(3.13823435722511,-6.27160936871312,12.8744563144973));
#77092=CARTESIAN_POINT('Ctrl Pts',(2.99897940001549,-6.33937858309311,12.8674800403988));
#77093=CARTESIAN_POINT('Ctrl Pts',(2.62347826779143,-6.50697452681015,12.8487708491087));
#77094=CARTESIAN_POINT('Ctrl Pts',(2.38380876437409,-6.59854598723767,12.8369615147659));
#77095=CARTESIAN_POINT('Ctrl Pts',(1.85424117501637,-6.76825311556731,12.811377009426));
#77096=CARTESIAN_POINT('Ctrl Pts',(1.56324006235294,-6.84132637222216,12.7976383887479));
#77097=CARTESIAN_POINT('Ctrl Pts',(0.855568587195019,-6.97150426794817,
12.7649596695206));
#77098=CARTESIAN_POINT('Ctrl Pts',(0.436695241808399,-7.01021907867285,
12.7462354263558));
#77099=CARTESIAN_POINT('Ctrl Pts',(-0.163179941827193,-7.01166313000463,
12.7193342721605));
#77100=CARTESIAN_POINT('Ctrl Pts',(-0.343185637050606,-7.00516021896718,
12.7112415635933));
#77101=CARTESIAN_POINT('Ctrl Pts',(-0.769108155320197,-6.97331602692858,
12.6918310613502));
#77102=CARTESIAN_POINT('Ctrl Pts',(-1.01432928660154,-6.94188715756695,
12.6804597123928));
#77103=CARTESIAN_POINT('Ctrl Pts',(-1.47788151274357,-6.85738516255359,
12.6587786344256));
#77104=CARTESIAN_POINT('Ctrl Pts',(-1.69633470984525,-6.8066375957765,12.6484799003081));
#77105=CARTESIAN_POINT('Ctrl Pts',(-2.00825421886854,-6.71822553786148,
12.6336734228701));
#77106=CARTESIAN_POINT('Ctrl Pts',(-2.10393107729957,-6.68887985024936,
12.6291167729688));
#77107=CARTESIAN_POINT('Ctrl Pts',(-2.58074358319704,-6.53139035754671,
12.60631797778));
#77108=CARTESIAN_POINT('Ctrl Pts',(-2.95098538578073,-6.37267508528968,
12.5883699807238));
#77109=CARTESIAN_POINT('Ctrl Pts',(-3.47347277529501,-6.09334533611682,
12.5618108019302));
#77110=CARTESIAN_POINT('Ctrl Pts',(-3.63763677496041,-5.99678808579302,
12.5532612756259));
#77111=CARTESIAN_POINT('Ctrl Pts',(-4.0136257607369,-5.75451461614941,12.5329398890637));
#77112=CARTESIAN_POINT('Ctrl Pts',(-4.22177221571216,-5.60359409819699,
12.5211110930139));
#77113=CARTESIAN_POINT('Ctrl Pts',(-4.65195936006898,-5.25407745300491,
12.4956078013151));
#77114=CARTESIAN_POINT('Ctrl Pts',(-4.87059536823905,-5.05206508726229,
12.4819665011341));
#77115=CARTESIAN_POINT('Ctrl Pts',(-5.40298159409744,-4.49337581611234,
12.4468864383951));
#77116=CARTESIAN_POINT('Ctrl Pts',(-5.69452329112035,-4.11765027914722,
12.4257872801048));
#77117=CARTESIAN_POINT('Ctrl Pts',(-6.0266051379498,-3.58620364131152,12.3976400975817));
#77118=CARTESIAN_POINT('Ctrl Pts',(-6.10308650553591,-3.45444069495734,
12.3907750264937));
#77119=CARTESIAN_POINT('Ctrl Pts',(-6.29333432179012,-3.10060983671043,
12.3724936953937));
#77120=CARTESIAN_POINT('Ctrl Pts',(-6.39964465845916,-2.87478420958052,
12.3610072612852));
#77121=CARTESIAN_POINT('Ctrl Pts',(-6.60945928994317,-2.35943369831851,
12.3354063821366));
#77122=CARTESIAN_POINT('Ctrl Pts',(-6.7064248963462,-2.06778877808697,12.3213318384269));
#77123=CARTESIAN_POINT('Ctrl Pts',(-6.88833652734206,-1.37085309518822,
12.2886232045153));
#77124=CARTESIAN_POINT('Ctrl Pts',(-6.95715104834616,-0.962534456948641,
12.2701853129887));
#77125=CARTESIAN_POINT('Ctrl Pts',(-7.00402891719657,-0.367372067515399,
12.2434166832279));
#77126=CARTESIAN_POINT('Ctrl Pts',(-7.01125028116588,-0.183715007268657,
12.2351614322727));
#77127=CARTESIAN_POINT('Ctrl Pts',(-7.01124991933926,0.0527219778476604,
12.224417531267));
#77128=CARTESIAN_POINT('Ctrl Pts',(-7.01065540621941,0.105431274551816,
12.2220151425037));
#77129=CARTESIAN_POINT('Ctrl Pts',(-7.00253636237598,0.465329391008556,
12.2055710359533));
#77130=CARTESIAN_POINT('Ctrl Pts',(-6.97541837636501,0.771741537925146,
12.19138509787));
#77131=CARTESIAN_POINT('Ctrl Pts',(-6.89070485524561,1.31751841335441,12.1660295661737));
#77132=CARTESIAN_POINT('Ctrl Pts',(-6.8404535809429,1.55751929512058,12.1548446687587));
#77133=CARTESIAN_POINT('Ctrl Pts',(-6.71974142120346,2.01346896744278,12.1334725173748));
#77134=CARTESIAN_POINT('Ctrl Pts',(-6.65116662782657,2.22955761477444,12.1232869808214));
#77135=CARTESIAN_POINT('Ctrl Pts',(-6.57226802086842,2.44190901230376,12.1131304899038));
#77136=CARTESIAN_POINT('',(-7.01089646739046,9.29430367064582E-6,12.7735343569104));
#77137=CARTESIAN_POINT('Ctrl Pts',(-6.57226799596304,2.44190907933526,12.6602932967));
#77138=CARTESIAN_POINT('Ctrl Pts',(-6.63771323763456,2.26576670328787,12.668824166077));
#77139=CARTESIAN_POINT('Ctrl Pts',(-6.69606694557729,2.08700883280449,12.6773550354539));
#77140=CARTESIAN_POINT('Ctrl Pts',(-6.74714280676067,1.90622414937955,12.6858859048309));
#77141=CARTESIAN_POINT('Ctrl Pts',(-6.76631859965158,1.83835080242298,12.6890887129787));
#77142=CARTESIAN_POINT('Ctrl Pts',(-6.78446905917518,1.77019192375625,12.6922915211265));
#77143=CARTESIAN_POINT('Ctrl Pts',(-6.80158615379011,1.70177917341546,12.6954943292742));
#77144=CARTESIAN_POINT('Ctrl Pts',(-6.84778947410182,1.51711604637734,12.7041395096671));
#77145=CARTESIAN_POINT('Ctrl Pts',(-6.88647402267709,1.33054685313653,12.71278469006));
#77146=CARTESIAN_POINT('Ctrl Pts',(-6.91750562972503,1.14269087036808,12.7214298704529));
#77147=CARTESIAN_POINT('Ctrl Pts',(-6.9486768695701,0.953989592791284,12.7301139515291));
#77148=CARTESIAN_POINT('Ctrl Pts',(-6.97212604646289,0.763990200189306,
12.7387980326054));
#77149=CARTESIAN_POINT('Ctrl Pts',(-6.98776927354008,0.573329872123468,
12.7474821136816));
#77150=CARTESIAN_POINT('Ctrl Pts',(-7.00341250061727,0.382669544057622,
12.7561661947579));
#77151=CARTESIAN_POINT('Ctrl Pts',(-7.0112497463365,0.191348574450929,12.7648502758341));
#77152=CARTESIAN_POINT('Ctrl Pts',(-7.01124999999384,9.29477234728852E-6,
12.7735343569104));
#77153=CARTESIAN_POINT('Ctrl Pts',(-7.01065084487527,9.29397804994014E-6,
12.7735343569104));
#77154=CARTESIAN_POINT('Ctrl Pts',(-7.01062348710872,-0.593030242553413,
12.8004522148775));
#77155=CARTESIAN_POINT('Ctrl Pts',(-6.78980718077563,-2.35224106726475,
12.8803012733571));
#77156=CARTESIAN_POINT('Ctrl Pts',(-5.33497512123331,-4.99561196811091,
13.0130815323492));
#77157=CARTESIAN_POINT('Ctrl Pts',(-2.29473593201848,-6.93918478514677,
13.1718751338868));
#77158=CARTESIAN_POINT('Ctrl Pts',(1.30483947524629,-7.19134844267406,13.3306687354243));
#77159=CARTESIAN_POINT('Ctrl Pts',(4.58636348188468,-5.69063867172615,13.4894623369618));
#77160=CARTESIAN_POINT('Ctrl Pts',(6.74997271289944,-2.80284977393084,13.6482559384993));
#77161=CARTESIAN_POINT('Ctrl Pts',(7.26829275987721,0.768126836418118,13.8070495400368));
#77162=CARTESIAN_POINT('Ctrl Pts',(6.0149843910269,4.15187442678777,13.9658431415743));
#77163=CARTESIAN_POINT('Ctrl Pts',(3.29553842701307,6.52361287602135,14.124636743112));
#77164=CARTESIAN_POINT('Ctrl Pts',(-0.227186892364047,7.30523679260615,
14.2834303446494));
#77165=CARTESIAN_POINT('Ctrl Pts',(-3.69453596762048,6.306227276595,14.4422239461869));
#77166=CARTESIAN_POINT('Ctrl Pts',(-5.72519280635199,4.29984055996828,14.5678486234894));
#77167=CARTESIAN_POINT('Ctrl Pts',(-6.42048420230567,2.84995900409766,14.6405421002794));
#77168=CARTESIAN_POINT('Ctrl Pts',(-6.57184683924635,2.44175302781609,14.6603043765569));
#77169=CARTESIAN_POINT('Origin',(0.,0.,10.));
#77170=CARTESIAN_POINT('',(-6.57226799596304,2.44190907933525,16.660297082902));
#77171=CARTESIAN_POINT('',(-6.57226800013471,2.44190906810743,16.1128890894906));
#77172=CARTESIAN_POINT('',(-6.57226799596304,2.44190907933527,10.));
#77173=CARTESIAN_POINT('',(-7.01124982298433,-0.000107840775152304,14.2261657896268));
#77174=CARTESIAN_POINT('Ctrl Pts',(-6.57226800013471,2.44190906810743,16.1128890894906));
#77175=CARTESIAN_POINT('Ctrl Pts',(-6.47321406132191,2.70850746067215,16.1000058294698));
#77176=CARTESIAN_POINT('Ctrl Pts',(-6.35802203610628,2.96885445807938,16.0872561549564));
#77177=CARTESIAN_POINT('Ctrl Pts',(-6.11278607817882,3.44290730218137,16.063349230731));
#77178=CARTESIAN_POINT('Ctrl Pts',(-5.9865259289693,3.65804157181628,16.0522047637981));
#77179=CARTESIAN_POINT('Ctrl Pts',(-5.76512324278877,3.99301443674072,16.0340052163809));
#77180=CARTESIAN_POINT('Ctrl Pts',(-5.67705232938408,4.11726672994885,16.0270415683926));
#77181=CARTESIAN_POINT('Ctrl Pts',(-5.44697938517922,4.42042679168906,16.0095706924358));
#77182=CARTESIAN_POINT('Ctrl Pts',(-5.30014880499447,4.5954521419498,15.9990469678999));
#77183=CARTESIAN_POINT('Ctrl Pts',(-4.9779943555893,4.94344655030019,15.9772751995181));
#77184=CARTESIAN_POINT('Ctrl Pts',(-4.80156860392471,5.11498132426437,15.9660499864233));
#77185=CARTESIAN_POINT('Ctrl Pts',(-4.39253707364053,5.47282278803232,15.9414226446631));
#77186=CARTESIAN_POINT('Ctrl Pts',(-4.15633294329696,5.65429669936464,15.9280881994101));
#77187=CARTESIAN_POINT('Ctrl Pts',(-3.69635153410875,5.96325623571244,15.9032689427213));
#77188=CARTESIAN_POINT('Ctrl Pts',(-3.47570383842022,6.0944990142313,15.891797475402));
#77189=CARTESIAN_POINT('Ctrl Pts',(-3.08003929870703,6.30135401943445,15.8715281027282));
#77190=CARTESIAN_POINT('Ctrl Pts',(-2.90820878087578,6.38247790616418,15.8628131036066));
#77191=CARTESIAN_POINT('Ctrl Pts',(-2.36238037897974,6.61354847374406,15.8355561554066));
#77192=CARTESIAN_POINT('Ctrl Pts',(-1.97861052089875,6.73832154450749,15.8170388773893));
#77193=CARTESIAN_POINT('Ctrl Pts',(-1.39396728244381,6.87411447245193,15.7898084032682));
#77194=CARTESIAN_POINT('Ctrl Pts',(-1.19988063888418,6.91063546964989,15.7809130319414));
#77195=CARTESIAN_POINT('Ctrl Pts',(-0.742005937103939,6.97691953969843,
15.7601389480075));
#77196=CARTESIAN_POINT('Ctrl Pts',(-0.477558167889971,6.99999401830781,
15.7483059297299));
#77197=CARTESIAN_POINT('Ctrl Pts',(-0.071541594459456,7.01230200129441,
15.7300409646309));
#77198=CARTESIAN_POINT('Ctrl Pts',(0.0694518297413624,7.01232297728411,
15.7236763218157));
#77199=CARTESIAN_POINT('Ctrl Pts',(0.269598471889345,7.00631548122516,15.7145556093177));
#77200=CARTESIAN_POINT('Ctrl Pts',(0.328820463306528,7.00378590394022,15.7118477134487));
#77201=CARTESIAN_POINT('Ctrl Pts',(0.564864238061188,6.99070318140796,15.7010250888106));
#77202=CARTESIAN_POINT('Ctrl Pts',(0.741289758964006,6.97420185498736,15.6928712188857));
#77203=CARTESIAN_POINT('Ctrl Pts',(1.21556669494736,6.91164077589433,15.6708602767436));
#77204=CARTESIAN_POINT('Ctrl Pts',(1.5113885660617,6.85303513894415,15.6570445299789));
#77205=CARTESIAN_POINT('Ctrl Pts',(2.04796722688772,6.71028777253538,15.6318160627858));
#77206=CARTESIAN_POINT('Ctrl Pts',(2.28968221947585,6.63170342031206,15.6203815247903));
#77207=CARTESIAN_POINT('Ctrl Pts',(2.78430226587554,6.4406216954805,15.5965970575234));
#77208=CARTESIAN_POINT('Ctrl Pts',(3.03589054895038,6.32592388874584,15.5842764082701));
#77209=CARTESIAN_POINT('Ctrl Pts',(3.39248247578323,6.13717129633892,15.5660809455926));
#77210=CARTESIAN_POINT('Ctrl Pts',(3.50326970837654,6.07461188121227,15.5603107276888));
#77211=CARTESIAN_POINT('Ctrl Pts',(3.8770596907804,5.84991179339844,15.5403914030376));
#77212=CARTESIAN_POINT('Ctrl Pts',(4.13101616092723,5.67342620114508,15.5261290515184));
#77213=CARTESIAN_POINT('Ctrl Pts',(4.5640574494822,5.3279501468504,15.5006975734885));
#77214=CARTESIAN_POINT('Ctrl Pts',(4.7474702178148,5.16519148501618,15.4895121993205));
#77215=CARTESIAN_POINT('Ctrl Pts',(5.13528968010257,4.78290025263909,15.4648364469547));
#77216=CARTESIAN_POINT('Ctrl Pts',(5.33490156270971,4.55918454745838,15.451416581044));
#77217=CARTESIAN_POINT('Ctrl Pts',(5.67545653054044,4.12440384653347,15.4266795025067));
#77218=CARTESIAN_POINT('Ctrl Pts',(5.82044042599043,3.91713966465796,15.4153751288039));
#77219=CARTESIAN_POINT('Ctrl Pts',(6.0519929210181,3.54478534353158,15.3954709343119));
#77220=CARTESIAN_POINT('Ctrl Pts',(6.14376517877187,3.38323349232264,15.3869516693107));
#77221=CARTESIAN_POINT('Ctrl Pts',(6.41712351483554,2.85413772396954,15.3595685492939));
#77222=CARTESIAN_POINT('Ctrl Pts',(6.57295313255433,2.47424260436356,15.3407246351983));
#77223=CARTESIAN_POINT('Ctrl Pts',(6.72443327156962,1.98736912548396,15.3175940616596));
#77224=CARTESIAN_POINT('Ctrl Pts',(6.75211111071317,1.89119926224203,15.3130693715883));
#77225=CARTESIAN_POINT('Ctrl Pts',(6.80701456618315,1.68382859921106,15.3033945398204));
#77226=CARTESIAN_POINT('Ctrl Pts',(6.83359439481513,1.57248655484323,15.2982495684081));
#77227=CARTESIAN_POINT('Ctrl Pts',(6.91411086075386,1.19445148976342,15.2809054776283));
#77228=CARTESIAN_POINT('Ctrl Pts',(6.9552485774386,0.925288465248311,15.2687713686226));
#77229=CARTESIAN_POINT('Ctrl Pts',(6.99284093723039,0.524293531278006,15.2506312357174));
#77230=CARTESIAN_POINT('Ctrl Pts',(7.00139882810741,0.39385532063017,15.24471480721));
#77231=CARTESIAN_POINT('Ctrl Pts',(7.01113784027787,0.134658067137653,15.2328823042758));
#77232=CARTESIAN_POINT('Ctrl Pts',(7.01242829845094,0.00595524213021864,
15.2269784786135));
#77233=CARTESIAN_POINT('Ctrl Pts',(7.00274564231746,-0.547200268871436,
15.2015473216456));
#77234=CARTESIAN_POINT('Ctrl Pts',(6.9567734181557,-0.970150860339461,15.1820183440202));
#77235=CARTESIAN_POINT('Ctrl Pts',(6.81204441730288,-1.68764841325407,15.1488231010692));
#77236=CARTESIAN_POINT('Ctrl Pts',(6.73151808987719,-1.9846346023707,15.1350453103604));
#77237=CARTESIAN_POINT('Ctrl Pts',(6.54694360840102,-2.52259064812961,15.1095705677517));
#77238=CARTESIAN_POINT('Ctrl Pts',(6.44836945883007,-2.76486185781343,15.0978863546916));
#77239=CARTESIAN_POINT('Ctrl Pts',(6.25261318948531,-3.17818601317203,15.0771209286326));
#77240=CARTESIAN_POINT('Ctrl Pts',(6.16133430604431,-3.35171531608751,15.0681250871579));
#77241=CARTESIAN_POINT('Ctrl Pts',(5.86542071670862,-3.86122966625953,15.0410256747702));
#77242=CARTESIAN_POINT('Ctrl Pts',(5.63967235195088,-4.18406047064741,15.0229525707483));
#77243=CARTESIAN_POINT('Ctrl Pts',(5.18872032020449,-4.72565879527589,14.9909741946301));
#77244=CARTESIAN_POINT('Ctrl Pts',(4.97365607875764,-4.9515067511912,14.9770068633338));
#77245=CARTESIAN_POINT('Ctrl Pts',(4.5600833701806,-5.33159016168186,14.9518470206776));
#77246=CARTESIAN_POINT('Ctrl Pts',(4.36695640702267,-5.49089266049856,14.9406627538777));
#77247=CARTESIAN_POINT('Ctrl Pts',(4.04300218969833,-5.73018685385692,14.9224074571156));
#77248=CARTESIAN_POINT('Ctrl Pts',(3.91734723294093,-5.8168115766629,14.9154288695813));
#77249=CARTESIAN_POINT('Ctrl Pts',(3.39161092388185,-6.15448046359543,14.8867444051407));
#77250=CARTESIAN_POINT('Ctrl Pts',(2.9694697078568,-6.36890287010425,14.8649897459829));
#77251=CARTESIAN_POINT('Ctrl Pts',(2.25495160802314,-6.64523477725838,14.8302705939297));
#77252=CARTESIAN_POINT('Ctrl Pts',(1.97452636909528,-6.73388454633304,14.8171006516703));
#77253=CARTESIAN_POINT('Ctrl Pts',(1.44955634332344,-6.86421632964355,14.7928724134066));
#77254=CARTESIAN_POINT('Ctrl Pts',(1.20677118307273,-6.91103315866354,14.7818245875844));
#77255=CARTESIAN_POINT('Ctrl Pts',(0.811968626806374,-6.9657219929638,14.7637600545402));
#77256=CARTESIAN_POINT('Ctrl Pts',(0.661279679390137,-6.98163901305464,
14.7568323441896));
#77257=CARTESIAN_POINT('Ctrl Pts',(0.280341268960479,-7.00943293982593,
14.7392994496589));
#77258=CARTESIAN_POINT('Ctrl Pts',(0.0497985847253759,-7.0148600681602,
14.7286765207645));
#77259=CARTESIAN_POINT('Ctrl Pts',(-0.425974199871209,-7.00260129428196,
14.7068268352416));
#77260=CARTESIAN_POINT('Ctrl Pts',(-0.67085810083832,-6.98339686005644,
14.6956218542012));
#77261=CARTESIAN_POINT('Ctrl Pts',(-1.21022597131532,-6.91246027691765,
14.6709704752847));
#77262=CARTESIAN_POINT('Ctrl Pts',(-1.5034326253318,-6.85466613445188,14.6575931814329));
#77263=CARTESIAN_POINT('Ctrl Pts',(-2.03824900714496,-6.71327125673849,
14.6328151647518));
#77264=CARTESIAN_POINT('Ctrl Pts',(-2.28070177805989,-6.63482217396105,
14.6214275118978));
#77265=CARTESIAN_POINT('Ctrl Pts',(-2.69359025074597,-6.47591370039997,
14.6013436667967));
#77266=CARTESIAN_POINT('Ctrl Pts',(-2.86605324530143,-6.40145479332655,
14.5927292390086));
#77267=CARTESIAN_POINT('Ctrl Pts',(-3.40162189590929,-6.1442430883952,14.5654092401235));
#77268=CARTESIAN_POINT('Ctrl Pts',(-3.75194879847424,-5.93680448944979,
14.5467259846613));
#77269=CARTESIAN_POINT('Ctrl Pts',(-4.33345536788112,-5.52034398292059,
14.5142777345529));
#77270=CARTESIAN_POINT('Ctrl Pts',(-4.57241919879514,-5.32409803969959,
14.5004294443539));
#77271=CARTESIAN_POINT('Ctrl Pts',(-4.97954552277554,-4.94206056938269,
14.4754216982898));
#77272=CARTESIAN_POINT('Ctrl Pts',(-5.15218694091067,-4.76180664406206,
14.4642708526047));
#77273=CARTESIAN_POINT('Ctrl Pts',(-5.41419227337445,-4.45728033082596,
14.4460623757251));
#77274=CARTESIAN_POINT('Ctrl Pts',(-5.50974036375189,-4.33861558836717,
14.4390963386193));
#77275=CARTESIAN_POINT('Ctrl Pts',(-5.76967118537896,-3.99335009238114,
14.4192569208734));
#77276=CARTESIAN_POINT('Ctrl Pts',(-5.92445947460721,-3.75988456864519,
14.4063519711039));
#77277=CARTESIAN_POINT('Ctrl Pts',(-6.17781879655627,-3.32307854214122,
14.3832172779257));
#77278=CARTESIAN_POINT('Ctrl Pts',(-6.28131766397622,-3.1230349350003,14.3729688694029));
#77279=CARTESIAN_POINT('Ctrl Pts',(-6.45961563677712,-2.73355131727058,
14.3535934252928));
#77280=CARTESIAN_POINT('Ctrl Pts',(-6.53614067663435,-2.54515293123263,
14.3444624188076));
#77281=CARTESIAN_POINT('Ctrl Pts',(-6.71009702690288,-2.05703842655861,
14.321233622511));
#77282=CARTESIAN_POINT('Ctrl Pts',(-6.79571099819986,-1.75360051321066,
14.3071991625631));
#77283=CARTESIAN_POINT('Ctrl Pts',(-6.88269316615911,-1.34074929814142,
14.2880559608511));
#77284=CARTESIAN_POINT('Ctrl Pts',(-6.90235109867921,-1.23556569372825,
14.2831709090337));
#77285=CARTESIAN_POINT('Ctrl Pts',(-6.98059134672087,-0.756448238171518,
14.2609281236194));
#77286=CARTESIAN_POINT('Ctrl Pts',(-7.01124416818815,-0.378589122575148,
14.2434505387525));
#77287=CARTESIAN_POINT('Ctrl Pts',(-7.01124999916793,-0.000108017167545701,
14.2261654923484));
#77288=CARTESIAN_POINT('Ctrl Pts',(-7.01124999917043,-0.000107854693215219,
14.2261654849283));
#77289=CARTESIAN_POINT('Ctrl Pts',(-7.01125249254275,0.161977411666877,
14.2187631303534));
#77290=CARTESIAN_POINT('Ctrl Pts',(-7.00563439082637,0.324015580569475,
14.2113972867494));
#77291=CARTESIAN_POINT('Ctrl Pts',(-6.96413850419295,0.921565848855817,
14.1843028034796));
#77292=CARTESIAN_POINT('Ctrl Pts',(-6.89319891062956,1.35363011315425,14.1649058588365));
#77293=CARTESIAN_POINT('Ctrl Pts',(-6.74939118881894,1.90274460620333,14.1393430625006));
#77294=CARTESIAN_POINT('Ctrl Pts',(-6.7127397031953,2.02826123620837,14.1334263278157));
#77295=CARTESIAN_POINT('Ctrl Pts',(-6.64125641127595,2.2498358571789,14.1228073803761));
#77296=CARTESIAN_POINT('Ctrl Pts',(-6.60780328543634,2.34626773728307,14.11813097137));
#77297=CARTESIAN_POINT('Ctrl Pts',(-6.57226804984416,2.44190893431709,14.1134456015891));
#77298=CARTESIAN_POINT('',(-7.01125169162915,0.000100138860277758,14.7735343587116));
#77299=CARTESIAN_POINT('Ctrl Pts',(-6.57184683924635,2.44175302781609,14.6603043765569));
#77300=CARTESIAN_POINT('Ctrl Pts',(-6.82589327429279,1.75662177524929,14.6934733007919));
#77301=CARTESIAN_POINT('Ctrl Pts',(-6.99426377786268,0.93198229720219,14.7312166275764));
#77302=CARTESIAN_POINT('Ctrl Pts',(-7.01180477314546,0.100836115687778,
14.7689599543609));
#77303=CARTESIAN_POINT('Ctrl Pts',(-7.01173456867506,0.000100185423145271,
14.7735343569104));
#77304=CARTESIAN_POINT('Ctrl Pts',(-7.01124999928488,0.000100138697088386,
14.7735343587179));
#77305=CARTESIAN_POINT('Ctrl Pts',(-7.01125267389351,-0.187163629012723,
14.7820385643826));
#77306=CARTESIAN_POINT('Ctrl Pts',(-7.00374855171984,-0.374461240683102,
14.7905427700473));
#77307=CARTESIAN_POINT('Ctrl Pts',(-6.98875556332075,-0.561179328426533,
14.799046975712));
#77308=CARTESIAN_POINT('Ctrl Pts',(-6.97376533234169,-0.747863076105076,
14.8075496173345));
#77309=CARTESIAN_POINT('Ctrl Pts',(-6.9512890083875,-0.933967203653135,
14.816052258957));
#77310=CARTESIAN_POINT('Ctrl Pts',(-6.92139650471126,-1.11888202553745,
14.8245549005794));
#77311=CARTESIAN_POINT('Ctrl Pts',(-6.8915029616306,-1.30380327717031,14.8330578378507));
#77312=CARTESIAN_POINT('Ctrl Pts',(-6.85419276906023,-1.487534833791,14.841560775122));
#77313=CARTESIAN_POINT('Ctrl Pts',(-6.80958736459116,-1.66947491340852,
14.8500637123933));
#77314=CARTESIAN_POINT('Ctrl Pts',(-6.76498375237899,-1.85140768262575,
14.8585663080143));
#77315=CARTESIAN_POINT('Ctrl Pts',(-6.71308558969616,-2.03154881797963,
14.8670689036353));
#77316=CARTESIAN_POINT('Ctrl Pts',(-6.65406490118876,-2.20930913483556,
14.8755714992563));
#77317=CARTESIAN_POINT('Ctrl Pts',(-6.59502990840115,-2.38711253376063,
14.8840761555702));
#77318=CARTESIAN_POINT('Ctrl Pts',(-6.52886903775336,-2.56253366664827,
14.8925808118841));
#77319=CARTESIAN_POINT('Ctrl Pts',(-6.45580374874602,-2.73499991228095,
14.9010854681979));
#77320=CARTESIAN_POINT('Ctrl Pts',(-6.4056331363489,-2.85342464280321,14.9069252290651));
#77321=CARTESIAN_POINT('Ctrl Pts',(-6.35220815662905,-2.97045651455718,
14.9127649899323));
#77322=CARTESIAN_POINT('Ctrl Pts',(-6.29561354753464,-3.08591584826909,
14.9186047507994));
#77323=CARTESIAN_POINT('Ctrl Pts',(-6.21293815891979,-3.25458288982283,
14.9271356781587));
#77324=CARTESIAN_POINT('Ctrl Pts',(-6.12346653014017,-3.4199544303168,14.935666605518));
#77325=CARTESIAN_POINT('Ctrl Pts',(-6.02748666786554,-3.5814844731205,14.9441975328773));
#77326=CARTESIAN_POINT('Ctrl Pts',(-5.93152502724454,-3.74298384965294,
14.952726840651));
#77327=CARTESIAN_POINT('Ctrl Pts',(-5.82905777520553,-3.90064292077405,
14.9612561484246));
#77328=CARTESIAN_POINT('Ctrl Pts',(-5.72041797044929,-4.05394188486476,
14.9697854561983));
#77329=CARTESIAN_POINT('Ctrl Pts',(-5.60619373389166,-4.21512090371173,
14.9787531975432));
#77330=CARTESIAN_POINT('Ctrl Pts',(-5.48514584979197,-4.37147945782676,
14.9877209388881));
#77331=CARTESIAN_POINT('Ctrl Pts',(-5.35771237882822,-4.52244896358719,
14.996688680233));
#77332=CARTESIAN_POINT('Ctrl Pts',(-5.23651305720476,-4.66603291798798,
15.0052177123568));
#77333=CARTESIAN_POINT('Ctrl Pts',(-5.10953820610418,-4.80474224204222,
15.0137467444806));
#77334=CARTESIAN_POINT('Ctrl Pts',(-4.97720561001781,-4.93812220161746,
15.0222757766044));
#77335=CARTESIAN_POINT('Ctrl Pts',(-4.84487169025588,-5.07150349534466,
15.030804894041));
#77336=CARTESIAN_POINT('Ctrl Pts',(-4.70718013638103,-5.19955510299028,
15.0393340114776));
#77337=CARTESIAN_POINT('Ctrl Pts',(-4.564585478796,-5.32185925868626,15.0478631289143));
#77338=CARTESIAN_POINT('Ctrl Pts',(-4.42196196891348,-5.44418816114307,
15.0563939721143));
#77339=CARTESIAN_POINT('Ctrl Pts',(-4.27443360686351,-5.56076709028424,
15.0649248153143));
#77340=CARTESIAN_POINT('Ctrl Pts',(-4.12248854157675,-5.67121810434658,
15.0734556585142));
#77341=CARTESIAN_POINT('Ctrl Pts',(-4.09908042679984,-5.68823379359926,
15.0747698897885));
#77342=CARTESIAN_POINT('Ctrl Pts',(-4.07556754898652,-5.70510412730578,
15.0760841210628));
#77343=CARTESIAN_POINT('Ctrl Pts',(-4.05195175757022,-5.72182781258084,
15.077398352337));
#77344=CARTESIAN_POINT('Ctrl Pts',(-3.89865712438817,-5.83038446243009,
15.0859292796963));
#77345=CARTESIAN_POINT('Ctrl Pts',(-3.74097119772733,-5.932795727898,15.0944602070555));
#77346=CARTESIAN_POINT('Ctrl Pts',(-3.57940810442678,-6.02871994576493,
15.1029911344148));
#77347=CARTESIAN_POINT('Ctrl Pts',(-3.41787568367117,-6.12462595254278,
15.1115204421885));
#77348=CARTESIAN_POINT('Ctrl Pts',(-3.25246782836961,-6.2140472131687,15.1200497499622));
#77349=CARTESIAN_POINT('Ctrl Pts',(-3.08372569427818,-6.29668662114835,
15.1285790577359));
#77350=CARTESIAN_POINT('Ctrl Pts',(-2.90630967733213,-6.38357395776686,
15.1375467990808));
#77351=CARTESIAN_POINT('Ctrl Pts',(-2.72520788662829,-6.46296368691256,
15.1465145404256));
#77352=CARTESIAN_POINT('Ctrl Pts',(-2.54107702163925,-6.53456610132586,
15.1554822817705));
#77353=CARTESIAN_POINT('Ctrl Pts',(-2.36595398875098,-6.60266566722387,
15.1640113138943));
#77354=CARTESIAN_POINT('Ctrl Pts',(-2.1880914764758,-6.66372151148871,15.1725403460181));
#77355=CARTESIAN_POINT('Ctrl Pts',(-2.00807391033613,-6.71753420036901,
15.1810693781419));
#77356=CARTESIAN_POINT('Ctrl Pts',(-1.82805454354573,-6.77134742751822,
15.1895984955785));
#77357=CARTESIAN_POINT('Ctrl Pts',(-1.64588037411524,-6.81791726992008,
15.1981276130152));
#77358=CARTESIAN_POINT('Ctrl Pts',(-1.46215040842577,-6.85709433693604,
15.2066567304518));
#77359=CARTESIAN_POINT('Ctrl Pts',(-1.27838326720843,-6.89627933095586,
15.2151875736518));
#77360=CARTESIAN_POINT('Ctrl Pts',(-1.09306000066057,-6.92806849899944,
15.2237184168518));
#77361=CARTESIAN_POINT('Ctrl Pts',(-0.906790083467622,-6.95236350509845,
15.2322492600517));
#77362=CARTESIAN_POINT('Ctrl Pts',(-0.878094004441462,-6.95610630707885,
15.233563491326));
#77363=CARTESIAN_POINT('Ctrl Pts',(-0.849375472554494,-6.95967134686518,
15.2348777226002));
#77364=CARTESIAN_POINT('Ctrl Pts',(-0.82063673039657,-6.96305837396356,
15.2361919538745));
#77365=CARTESIAN_POINT('Ctrl Pts',(-0.634088041024037,-6.98504421671893,
15.2447228812337));
#77366=CARTESIAN_POINT('Ctrl Pts',(-0.446623371802602,-6.99953271404237,
15.2532538085928));
#77367=CARTESIAN_POINT('Ctrl Pts',(-0.258857652592978,-7.00646981569136,
15.261784735952));
#77368=CARTESIAN_POINT('Ctrl Pts',(-0.0711275804627589,-7.01340560034055,
15.2703140437257));
#77369=CARTESIAN_POINT('Ctrl Pts',(0.116903121738672,-7.01279283896196,
15.2788433514993));
#77370=CARTESIAN_POINT('Ctrl Pts',(0.304617106579406,-7.00462953916045,
15.2873726592729));
#77371=CARTESIAN_POINT('Ctrl Pts',(0.501980187799274,-6.99604661976255,
15.2963404006178));
#77372=CARTESIAN_POINT('Ctrl Pts',(0.698992770738884,-6.97911647346185,
15.3053081419628));
#77373=CARTESIAN_POINT('Ctrl Pts',(0.894939586006176,-6.95389888479111,
15.3142758833077));
#77374=CARTESIAN_POINT('Ctrl Pts',(1.08130052324435,-6.92991496112717,15.3228049154314));
#77375=CARTESIAN_POINT('Ctrl Pts',(1.26669714844205,-6.89843511430174,15.3313339475551));
#77376=CARTESIAN_POINT('Ctrl Pts',(1.45052084732403,-6.85956382242912,15.3398629796788));
#77377=CARTESIAN_POINT('Ctrl Pts',(1.63434638492899,-6.82069214174081,15.3483920971153));
#77378=CARTESIAN_POINT('Ctrl Pts',(1.81659866587765,-6.77442893478876,15.3569212145519));
#77379=CARTESIAN_POINT('Ctrl Pts',(1.99668021413705,-6.72092959976324,15.3654503319884));
#77380=CARTESIAN_POINT('Ctrl Pts',(2.17679819971142,-6.66741943979679,15.3739811751884));
#77381=CARTESIAN_POINT('Ctrl Pts',(2.35474428207199,-6.60667031551607,15.3825120183883));
#77382=CARTESIAN_POINT('Ctrl Pts',(2.52993621872838,-6.53888746589711,15.3910428615882));
#77383=CARTESIAN_POINT('Ctrl Pts',(2.5569256635951,-6.52844508186041,15.3923570928628));
#77384=CARTESIAN_POINT('Ctrl Pts',(2.58384977831759,-6.51783585807759,15.3936713241374));
#77385=CARTESIAN_POINT('Ctrl Pts',(2.61070647377534,-6.50706064750341,15.394985555412));
#77386=CARTESIAN_POINT('Ctrl Pts',(2.78503843687495,-6.43711668827126,15.4035164827715));
#77387=CARTESIAN_POINT('Ctrl Pts',(2.95658779836659,-6.36015088199504,15.4120474101311));
#77388=CARTESIAN_POINT('Ctrl Pts',(3.12478871300326,-6.27640996602257,15.4205783374906));
#77389=CARTESIAN_POINT('Ctrl Pts',(3.29295769491275,-6.19268494815522,15.4291076452646));
#77390=CARTESIAN_POINT('Ctrl Pts',(3.45777922458081,-6.10218752384163,15.4376369530385));
#77391=CARTESIAN_POINT('Ctrl Pts',(3.61871023981204,-6.00521130042728,15.4461662608125));
#77392=CARTESIAN_POINT('Ctrl Pts',(3.78791362151531,-5.90325019042656,15.4551340021572));
#77393=CARTESIAN_POINT('Ctrl Pts',(3.95281566599083,-5.79412685004287,15.464101743502));
#77394=CARTESIAN_POINT('Ctrl Pts',(4.11281687907556,-5.67823598326903,15.4730694848467));
#77395=CARTESIAN_POINT('Ctrl Pts',(4.26499070231872,-5.5680145922187,15.4815985169708));
#77396=CARTESIAN_POINT('Ctrl Pts',(4.41273147077283,-5.45167218924217,15.4901275490948));
#77397=CARTESIAN_POINT('Ctrl Pts',(4.55555472963676,-5.32959169803693,15.4986565812189));
#77398=CARTESIAN_POINT('Ctrl Pts',(4.69837941710968,-5.20750998570504,15.5071856986557));
#77399=CARTESIAN_POINT('Ctrl Pts',(4.83628626605543,-5.07969027187068,15.5157148160926));
#77400=CARTESIAN_POINT('Ctrl Pts',(4.96882496409711,-4.94655486562773,15.5242439335294));
#77401=CARTESIAN_POINT('Ctrl Pts',(5.10139047973582,-4.81339252105108,15.5327747767297));
#77402=CARTESIAN_POINT('Ctrl Pts',(5.22858545966223,-4.67491255350123,15.5413056199299));
#77403=CARTESIAN_POINT('Ctrl Pts',(5.34999681375057,-4.5315737504049,15.5498364631302));
#77404=CARTESIAN_POINT('Ctrl Pts',(5.36870101387559,-4.509491485703,15.5511506944033));
#77405=CARTESIAN_POINT('Ctrl Pts',(5.38726802491303,-4.48729397047949,15.5524649256764));
#77406=CARTESIAN_POINT('Ctrl Pts',(5.40569642042965,-4.46498295323219,15.5537791569495));
#77407=CARTESIAN_POINT('Ctrl Pts',(5.52531867163153,-4.3201578594079,15.5623100843081));
#77408=CARTESIAN_POINT('Ctrl Pts',(5.63913799204196,-4.17049797480998,15.5708410116668));
#77409=CARTESIAN_POINT('Ctrl Pts',(5.74677554440972,-4.01649068275708,15.5793719390254));
#77410=CARTESIAN_POINT('Ctrl Pts',(5.854392661927,-3.86251262878991,15.5879012467985));
#77411=CARTESIAN_POINT('Ctrl Pts',(5.95583017811103,-3.70418906531051,15.5964305545716));
#77412=CARTESIAN_POINT('Ctrl Pts',(6.05075168607242,-3.54203763333929,15.6049598623446));
#77413=CARTESIAN_POINT('Ctrl Pts',(6.15055246172042,-3.37155110156459,15.6139276036898));
#77414=CARTESIAN_POINT('Ctrl Pts',(6.24314950152241,-3.19683311189914,15.622895345035));
#77415=CARTESIAN_POINT('Ctrl Pts',(6.32820521176638,-3.0185170796722,15.6318630863802));
#77416=CARTESIAN_POINT('Ctrl Pts',(6.40909992728111,-2.84892441320293,15.6403921185034));
#77417=CARTESIAN_POINT('Ctrl Pts',(6.48317339141995,-2.67607762758904,15.6489211506266));
#77418=CARTESIAN_POINT('Ctrl Pts',(6.55018339351771,-2.50054475540529,15.6574501827497));
#77419=CARTESIAN_POINT('Ctrl Pts',(6.61719406589258,-2.3250101274289,15.6659793001857));
#77420=CARTESIAN_POINT('Ctrl Pts',(6.67714102887042,-2.14678964641217,15.6745084176218));
#77421=CARTESIAN_POINT('Ctrl Pts',(6.72983089626059,-1.96646959555351,15.6830375350578));
#77422=CARTESIAN_POINT('Ctrl Pts',(6.78253142480604,-1.78611305912071,15.6915683782572));
#77423=CARTESIAN_POINT('Ctrl Pts',(6.82797183996303,-1.60365639852797,15.7000992214567));
#77424=CARTESIAN_POINT('Ctrl Pts',(6.86600889366878,-1.41970012135,15.7086300646561));
#77425=CARTESIAN_POINT('Ctrl Pts',(6.87186874649866,-1.39136047339163,15.7099442959331));
#77426=CARTESIAN_POINT('Ctrl Pts',(6.8775529907978,-1.36298525616568,15.71125852721));
#77427=CARTESIAN_POINT('Ctrl Pts',(6.88306121050986,-1.33457668752101,15.712572758487));
#77428=CARTESIAN_POINT('Ctrl Pts',(6.91881612143904,-1.15017121812908,15.7211036858473));
#77429=CARTESIAN_POINT('Ctrl Pts',(6.9471622224435,-0.964296482546905,15.7296346132076));
#77430=CARTESIAN_POINT('Ctrl Pts',(6.9680000249124,-0.777561711583614,15.7381655405678));
#77431=CARTESIAN_POINT('Ctrl Pts',(6.98883387135136,-0.590862391975856,
15.7466948483425));
#77432=CARTESIAN_POINT('Ctrl Pts',(7.00216222993002,-0.403303667003667,
15.7552241561173));
#77433=CARTESIAN_POINT('Ctrl Pts',(7.00793734741366,-0.215501037641931,
15.763753463892));
#77434=CARTESIAN_POINT('Ctrl Pts',(7.01400932431902,-0.0180447553275768,
15.7727212052364));
#77435=CARTESIAN_POINT('Ctrl Pts',(7.0117310595895,0.17968080497015,15.7816889465807));
#77436=CARTESIAN_POINT('Ctrl Pts',(7.00110914759811,0.376957910008705,15.7906566879251));
#77437=CARTESIAN_POINT('Ctrl Pts',(6.99100686820331,0.564584058192902,15.7991857200499));
#77438=CARTESIAN_POINT('Ctrl Pts',(6.97335780402424,0.75180424923359,15.8077147521747));
#77439=CARTESIAN_POINT('Ctrl Pts',(6.94822102678319,0.93800379821618,15.8162437842995));
#77440=CARTESIAN_POINT('Ctrl Pts',(6.92308399810814,1.12420520968483,15.824772901737));
#77441=CARTESIAN_POINT('Ctrl Pts',(6.89045915088879,1.30938565568474,15.8333020191746));
#77442=CARTESIAN_POINT('Ctrl Pts',(6.85045716252722,1.49293778399487,15.8418311366122));
#77443=CARTESIAN_POINT('Ctrl Pts',(6.81044708024879,1.67652705185048,15.8503619798132));
#77444=CARTESIAN_POINT('Ctrl Pts',(6.7630569416163,1.85848704497405,15.8588928230141));
#77445=CARTESIAN_POINT('Ctrl Pts',(6.70844825699151,2.03822190788138,15.8674236662151));
#77446=CARTESIAN_POINT('Ctrl Pts',(6.7000354378544,2.06591121965774,15.8687378974849));
#77447=CARTESIAN_POINT('Ctrl Pts',(6.6914513948919,2.09354774952639,15.8700521287547));
#77448=CARTESIAN_POINT('Ctrl Pts',(6.68269682383722,2.12112935088268,15.8713663600245));
#77449=CARTESIAN_POINT('Ctrl Pts',(6.62586922322023,2.30016681787704,15.8798972873826));
#77450=CARTESIAN_POINT('Ctrl Pts',(6.56183281267897,2.47694989647158,15.8884282147407));
#77451=CARTESIAN_POINT('Ctrl Pts',(6.49079170234618,2.65089600687277,15.8969591420988));
#77452=CARTESIAN_POINT('Ctrl Pts',(6.41976407907667,2.82480909382896,15.9054884498714));
#77453=CARTESIAN_POINT('Ctrl Pts',(6.34173452556159,2.99588600406622,15.9140177576439));
#77454=CARTESIAN_POINT('Ctrl Pts',(6.25695558195389,3.16356340349867,15.9225470654165));
#77455=CARTESIAN_POINT('Ctrl Pts',(6.16781873074729,3.33985995507027,15.9315148067619));
#77456=CARTESIAN_POINT('Ctrl Pts',(6.07122048289653,3.5123979688746,15.9404825481074));
#77457=CARTESIAN_POINT('Ctrl Pts',(5.96751001349756,3.68055033946098,15.9494502894529));
#77458=CARTESIAN_POINT('Ctrl Pts',(5.86887314487242,3.84047655889336,15.9579793215755));
#77459=CARTESIAN_POINT('Ctrl Pts',(5.76380346821951,3.99643569594641,15.9665083536982));
#77460=CARTESIAN_POINT('Ctrl Pts',(5.65264693906213,4.14791624129653,15.9750373858208));
#77461=CARTESIAN_POINT('Ctrl Pts',(5.54148929804606,4.29939830185195,15.9835665032563));
#77462=CARTESIAN_POINT('Ctrl Pts',(5.4242448666277,4.44640143624321,15.9920956206917));
#77463=CARTESIAN_POINT('Ctrl Pts',(5.30130140845831,4.58844526383153,16.0006247381272));
#77464=CARTESIAN_POINT('Ctrl Pts',(5.17833307417169,4.7305178322651,16.0091555813261));
#77465=CARTESIAN_POINT('Ctrl Pts',(5.04966361108679,4.86762885876985,16.017686424525));
#77466=CARTESIAN_POINT('Ctrl Pts',(4.91571992023791,4.99933237825574,16.0262172677239));
#77467=CARTESIAN_POINT('Ctrl Pts',(4.89508503291352,5.01962215276915,16.0275314990033));
#77468=CARTESIAN_POINT('Ctrl Pts',(4.87432504185004,5.03978365965778,16.0288457302827));
#77469=CARTESIAN_POINT('Ctrl Pts',(4.85344158498705,5.05981534679067,16.0301599615621));
#77470=CARTESIAN_POINT('Ctrl Pts',(4.71788306016509,5.18984487088935,16.0386908889215));
#77471=CARTESIAN_POINT('Ctrl Pts',(4.57707285503567,5.31444585360377,16.0472218162808));
#77472=CARTESIAN_POINT('Ctrl Pts',(4.43146892713431,5.43320436854193,16.0557527436401));
#77473=CARTESIAN_POINT('Ctrl Pts',(4.28589264195185,5.5519403373284,16.0642820514138));
#77474=CARTESIAN_POINT('Ctrl Pts',(4.13552468734416,5.66483585838425,16.0728113591876));
#77475=CARTESIAN_POINT('Ctrl Pts',(3.98085634081318,5.7715170758049,16.0813406669613));
#77476=CARTESIAN_POINT('Ctrl Pts',(3.81823754891069,5.8836820474021,16.0903084083061));
#77477=CARTESIAN_POINT('Ctrl Pts',(3.65086490236855,5.98897679978346,16.099276149651));
#77478=CARTESIAN_POINT('Ctrl Pts',(3.47934504643782,6.08701771069615,16.1082438909959));
#77479=CARTESIAN_POINT('Ctrl Pts',(3.3162160817572,6.18026238028118,16.1167729231197));
#77480=CARTESIAN_POINT('Ctrl Pts',(3.14933626687556,6.26694580878486,16.1253019552436));
#77481=CARTESIAN_POINT('Ctrl Pts',(2.97925411531266,6.34678434160895,16.1338309873674));
#77482=CARTESIAN_POINT('Ctrl Pts',(2.8091702624791,6.42662367302921,16.1423601048041));
#77483=CARTESIAN_POINT('Ctrl Pts',(2.63588428751379,6.49961784478217,16.1508892222408));
#77484=CARTESIAN_POINT('Ctrl Pts',(2.45996652388457,6.56553053940558,16.1594183396775));
#77485=CARTESIAN_POINT('Ctrl Pts',(2.28401316543242,6.63145657066223,16.1679491828775));
#77486=CARTESIAN_POINT('Ctrl Pts',(2.10542724180266,6.69029815638646,16.1764800260775));
#77487=CARTESIAN_POINT('Ctrl Pts',(1.92479698862914,6.74186792477161,16.1850108692775));
#77488=CARTESIAN_POINT('Ctrl Pts',(1.89696973613013,6.74981257934058,16.1863251005515));
#77489=CARTESIAN_POINT('Ctrl Pts',(1.86909399370878,6.75758474548673,16.1876393318256));
#77490=CARTESIAN_POINT('Ctrl Pts',(1.84117194226723,6.76518384388096,16.1889535630996));
#77491=CARTESIAN_POINT('Ctrl Pts',(1.6599245489094,6.81451104960965,16.1974844904631));
#77492=CARTESIAN_POINT('Ctrl Pts',(1.47666268897109,6.85655875452296,16.2060154178265));
#77493=CARTESIAN_POINT('Ctrl Pts',(1.29198654137254,6.89118257916682,16.21454634519));
#77494=CARTESIAN_POINT('Ctrl Pts',(1.10734545430354,6.92579983052201,16.2230756529679));
#77495=CARTESIAN_POINT('Ctrl Pts',(0.921290916223461,6.95299595784342,16.2316049607458));
#77496=CARTESIAN_POINT('Ctrl Pts',(0.734433194305613,6.97267770986169,16.2401342685236));
#77497=CARTESIAN_POINT('Ctrl Pts',(0.537970390793006,6.99337116657229,16.2491020098664));
#77498=CARTESIAN_POINT('Ctrl Pts',(0.340620014977392,7.00575732159409,16.2580697512092));
#77499=CARTESIAN_POINT('Ctrl Pts',(0.143098313982019,7.00978954284902,16.267037492552));
#77500=CARTESIAN_POINT('Ctrl Pts',(-0.0447604644297263,7.0136245045541,
16.27556652468));
#77501=CARTESIAN_POINT('Ctrl Pts',(-0.232773874737426,7.00990335278436,
16.284095556808));
#77502=CARTESIAN_POINT('Ctrl Pts',(-0.420324544240595,6.99863942777515,
16.292624588936));
#77503=CARTESIAN_POINT('Ctrl Pts',(-0.607877089746412,6.98737539009691,
16.3011537063769));
#77504=CARTESIAN_POINT('Ctrl Pts',(-0.794966579746772,6.96856845001131,
16.3096828238178));
#77505=CARTESIAN_POINT('Ctrl Pts',(-0.980979128331375,6.94228395503081,
16.3182119412587));
#77506=CARTESIAN_POINT('Ctrl Pts',(-1.16702931429466,6.91599414170217,16.3267427844628));
#77507=CARTESIAN_POINT('Ctrl Pts',(-1.35200182054923,6.88222379533962,16.335273627667));
#77508=CARTESIAN_POINT('Ctrl Pts',(-1.53529045784463,6.84108980883538,16.3438044708711));
#77509=CARTESIAN_POINT('Ctrl Pts',(-1.56352725110343,6.83475285369201,16.3451187021265));
#77510=CARTESIAN_POINT('Ctrl Pts',(-1.5917241011711,6.82824123295892,16.3464329333818));
#77511=CARTESIAN_POINT('Ctrl Pts',(-1.61987881577253,6.82155548131886,16.3477471646371));
#77512=CARTESIAN_POINT('Ctrl Pts',(-1.80263647253457,6.77815698409637,16.3562780919815));
#77513=CARTESIAN_POINT('Ctrl Pts',(-1.98368036090121,6.72740238701715,16.3648090193258));
#77514=CARTESIAN_POINT('Ctrl Pts',(-2.16241437270051,6.66945204969931,16.3733399466702));
#77515=CARTESIAN_POINT('Ctrl Pts',(-2.34111445207794,6.61151271417835,16.381869254429));
#77516=CARTESIAN_POINT('Ctrl Pts',(-2.51750523886751,6.5463804590188,16.3903985621877));
#77517=CARTESIAN_POINT('Ctrl Pts',(-2.69100622734431,6.47426536735205,16.3989278699465));
#77518=CARTESIAN_POINT('Ctrl Pts',(-2.87342571941059,6.39844333021178,16.4078956112989));
#77519=CARTESIAN_POINT('Ctrl Pts',(-3.05265015788515,6.31490179316538,16.4168633526512));
#77520=CARTESIAN_POINT('Ctrl Pts',(-3.22802827723604,6.22394248076447,16.4258310940035));
#77521=CARTESIAN_POINT('Ctrl Pts',(-3.39482675551182,6.13743297233983,16.4343601261124));
#77522=CARTESIAN_POINT('Ctrl Pts',(-3.55814595624871,6.04421426208676,16.4428891582213));
#77523=CARTESIAN_POINT('Ctrl Pts',(-3.71745013063991,5.94459343342379,16.4514181903302));
#77524=CARTESIAN_POINT('Ctrl Pts',(-3.87675589849528,5.84497160828839,16.4599473077521));
#77525=CARTESIAN_POINT('Ctrl Pts',(-4.03204630186012,5.73894770187934,16.4684764251739));
#77526=CARTESIAN_POINT('Ctrl Pts',(-4.18281353555963,5.62687279838803,16.4770055425957));
#77527=CARTESIAN_POINT('Ctrl Pts',(-4.33361127518242,5.51477521789772,16.4855363857811));
#77528=CARTESIAN_POINT('Ctrl Pts',(-4.47988377199704,5.39662437836349,16.4940672289665));
#77529=CARTESIAN_POINT('Ctrl Pts',(-4.62115464027263,5.27281294502154,16.502598072152));
#77530=CARTESIAN_POINT('Ctrl Pts',(-4.64291832747283,5.25373899623116,16.5039123034928));
#77531=CARTESIAN_POINT('Ctrl Pts',(-4.66456337440864,5.23453077896803,16.5052265348337));
#77532=CARTESIAN_POINT('Ctrl Pts',(-4.68608811179318,5.21518981159944,16.5065407661746));
#77533=CARTESIAN_POINT('Ctrl Pts',(-4.82580898526699,5.08964417513982,16.515071674014));
#77534=CARTESIAN_POINT('Ctrl Pts',(-4.9605056051731,4.95845889673718,16.5236025818534));
#77535=CARTESIAN_POINT('Ctrl Pts',(-5.08973123700736,4.82205998485414,16.5321334896928));
#77536=CARTESIAN_POINT('Ctrl Pts',(-5.21893223860777,4.68568707042261,16.5406627715525));
#77537=CARTESIAN_POINT('Ctrl Pts',(-5.34266412260317,4.54410272777213,16.5491920534121));
#77538=CARTESIAN_POINT('Ctrl Pts',(-5.46051764513451,4.39776916284548,16.5577213352718));
#77539=CARTESIAN_POINT('Ctrl Pts',(-5.57862951534997,4.25111481889759,16.566269314241));
#77540=CARTESIAN_POINT('Ctrl Pts',(-5.69083701234519,4.09969063387712,16.5748172932102));
#77541=CARTESIAN_POINT('Ctrl Pts',(-5.79676882468995,3.94399515156937,16.5833652721794));
#77542=CARTESIAN_POINT('Ctrl Pts',(-5.90246402738797,3.78864743120634,16.5918941583544));
#77543=CARTESIAN_POINT('Ctrl Pts',(-6.00191139183001,3.62904773780094,16.6004230445295));
#77544=CARTESIAN_POINT('Ctrl Pts',(-6.09478521133198,3.46572067400548,16.6089519307045));
#77545=CARTESIAN_POINT('Ctrl Pts',(-6.18797089231485,3.30184517341417,16.6175094560708));
#77546=CARTESIAN_POINT('Ctrl Pts',(-6.27453863167416,3.13421748467873,16.626066981437));
#77547=CARTESIAN_POINT('Ctrl Pts',(-6.35420545475499,2.96339325794973,16.6346245068033));
#77548=CARTESIAN_POINT('Ctrl Pts',(-6.43387227783583,2.79256903122072,16.6431820321695));
#77549=CARTESIAN_POINT('Ctrl Pts',(-6.50663805954855,2.61854855142873,16.6517395575358));
#77550=CARTESIAN_POINT('Ctrl Pts',(-6.57226799596304,2.44190907933527,16.660297082902));
#77551=CARTESIAN_POINT('Origin',(0.,0.,10.));
#77552=CARTESIAN_POINT('',(-6.57226799068689,2.44190909353574,18.6606197598975));
#77553=CARTESIAN_POINT('',(-6.57226799602084,2.4419090791797,18.1135379835087));
#77554=CARTESIAN_POINT('',(-6.57226799596304,2.44190907933527,10.));
#77555=CARTESIAN_POINT('',(5.31037376991263,4.57794244025893,20.));
#77556=CARTESIAN_POINT('Ctrl Pts',(5.31037376991263,4.57794244025893,20.));
#77557=CARTESIAN_POINT('Ctrl Pts',(5.55565403033897,4.29341945242257,19.9829453662211));
#77558=CARTESIAN_POINT('Ctrl Pts',(5.77767458878684,3.98964000774632,19.9662196358398));
#77559=CARTESIAN_POINT('Ctrl Pts',(6.08131410266316,3.49529120368377,19.940098230979));
#77560=CARTESIAN_POINT('Ctrl Pts',(6.1806630589801,3.31645053343412,19.9308546963185));
#77561=CARTESIAN_POINT('Ctrl Pts',(6.41359417612191,2.85021658136766,19.907128727684));
#77562=CARTESIAN_POINT('Ctrl Pts',(6.53577546978317,2.5576468760439,19.8925703550586));
#77563=CARTESIAN_POINT('Ctrl Pts',(6.69473545277011,2.0903225110574,19.8698046355055));
#77564=CARTESIAN_POINT('Ctrl Pts',(6.74535157808797,1.92071957393734,19.8616423248671));
#77565=CARTESIAN_POINT('Ctrl Pts',(6.8152036502563,1.64961803264622,19.8488003608201));
#77566=CARTESIAN_POINT('Ctrl Pts',(6.83870751356947,1.54929681753912,19.8440923805288));
#77567=CARTESIAN_POINT('Ctrl Pts',(6.9143733926581,1.19094681265089,19.8274618806421));
#77568=CARTESIAN_POINT('Ctrl Pts',(6.95420852687898,0.930538557183069,19.8156952816196));
#77569=CARTESIAN_POINT('Ctrl Pts',(7.00881853782953,0.360400403229322,19.7900396878859));
#77570=CARTESIAN_POINT('Ctrl Pts',(7.017895173745,0.0506844751069775,19.7761629443979));
#77571=CARTESIAN_POINT('Ctrl Pts',(6.99209058764831,-0.648427924427146,
19.7444234601358));
#77572=CARTESIAN_POINT('Ctrl Pts',(6.94519564887154,-1.03635691554328,19.7265001555966));
#77573=CARTESIAN_POINT('Ctrl Pts',(6.82655782453199,-1.61068380040626,19.6995319153759));
#77574=CARTESIAN_POINT('Ctrl Pts',(6.77876578482327,-1.8012580651144,19.6905184966276));
#77575=CARTESIAN_POINT('Ctrl Pts',(6.65032448269472,-2.2352778291736,19.6699693779279));
#77576=CARTESIAN_POINT('Ctrl Pts',(6.56419733625245,-2.47681250315935,19.65850962379));
#77577=CARTESIAN_POINT('Ctrl Pts',(6.34902861498852,-2.98953904402741,19.6336010567148));
#77578=CARTESIAN_POINT('Ctrl Pts',(6.21540594260978,-3.25825620184757,19.620165435284));
#77579=CARTESIAN_POINT('Ctrl Pts',(5.83012947859726,-3.9225460193432,19.5853624107861));
#77580=CARTESIAN_POINT('Ctrl Pts',(5.55529778581468,-4.30295532809216,19.5638058413775));
#77581=CARTESIAN_POINT('Ctrl Pts',(5.14165688626341,-4.76917849267796,19.5351939530897));
#77582=CARTESIAN_POINT('Ctrl Pts',(5.03486121828757,-4.88178997914994,19.5280970198765));
#77583=CARTESIAN_POINT('Ctrl Pts',(4.74773465933112,-5.16509921326354,19.509814228205));
#77584=CARTESIAN_POINT('Ctrl Pts',(4.56191851216949,-5.32992844535567,19.4987169755029));
#77585=CARTESIAN_POINT('Ctrl Pts',(4.12664730964557,-5.67656647657017,19.4737940545565));
#77586=CARTESIAN_POINT('Ctrl Pts',(3.87314804944286,-5.85246486991511,19.4599770166617));
#77587=CARTESIAN_POINT('Ctrl Pts',(3.24938844208059,-6.2269526488941,19.4269736096934));
#77588=CARTESIAN_POINT('Ctrl Pts',(2.87124052423138,-6.4101036203911,19.4076836649396));
#77589=CARTESIAN_POINT('Ctrl Pts',(2.31094660388895,-6.62189052319189,19.3801419837845));
#77590=CARTESIAN_POINT('Ctrl Pts',(2.14049861486476,-6.67893524115426,19.3719020764516));
#77591=CARTESIAN_POINT('Ctrl Pts',(1.72437665409792,-6.80063266404377,19.3522215577717));
#77592=CARTESIAN_POINT('Ctrl Pts',(1.47701297532513,-6.85860891162722,19.3408675238262));
#77593=CARTESIAN_POINT('Ctrl Pts',(0.932207350322201,-6.95545063084083,
19.316082598644));
#77594=CARTESIAN_POINT('Ctrl Pts',(0.634316160635225,-6.98891576151712,
19.3026646152065));
#77595=CARTESIAN_POINT('Ctrl Pts',(-0.124644237268658,-7.02524261816539,
19.2682337929834));
#77596=CARTESIAN_POINT('Ctrl Pts',(-0.585535579499694,-7.00190686331401,
19.2470436360377));
#77597=CARTESIAN_POINT('Ctrl Pts',(-1.19980159345292,-6.90970025782923,
19.2185170065727));
#77598=CARTESIAN_POINT('Ctrl Pts',(-1.35794966021049,-6.88036744296449,
19.2111570507939));
#77599=CARTESIAN_POINT('Ctrl Pts',(-1.77425050592426,-6.78823912375196,
19.1918237362095));
#77600=CARTESIAN_POINT('Ctrl Pts',(-2.03008335220301,-6.71616862577159,
19.1799590454234));
#77601=CARTESIAN_POINT('Ctrl Pts',(-2.54972011497008,-6.53736841838324,
19.1553416626722));
#77602=CARTESIAN_POINT('Ctrl Pts',(-2.81236293520454,-6.42875336597622,
19.1426042906477));
#77603=CARTESIAN_POINT('Ctrl Pts',(-3.48462403918343,-6.10164008147154,
19.1087121466996));
#77604=CARTESIAN_POINT('Ctrl Pts',(-3.88039834917778,-5.85790973655747,
19.0873556188328));
#77605=CARTESIAN_POINT('Ctrl Pts',(-4.3727690342133,-5.48275957578848,19.0589313843948));
#77606=CARTESIAN_POINT('Ctrl Pts',(-4.49318056685592,-5.3845233618943,19.0518229749148));
#77607=CARTESIAN_POINT('Ctrl Pts',(-4.77148915802518,-5.1416271231717,19.0350754083327));
#77608=CARTESIAN_POINT('Ctrl Pts',(-4.92622018437202,-4.99357541539983,
19.0254867024873));
#77609=CARTESIAN_POINT('Ctrl Pts',(-5.23516438800496,-4.66961003420178,
19.0054335969687));
#77610=CARTESIAN_POINT('Ctrl Pts',(-5.38783954789928,-4.4925925650562,18.9949805237359));
#77611=CARTESIAN_POINT('Ctrl Pts',(-5.59301834925927,-4.22916425451325,
18.9799308442156));
#77612=CARTESIAN_POINT('Ctrl Pts',(-5.65293930776931,-4.14873010642308,
18.9753991570484));
#77613=CARTESIAN_POINT('Ctrl Pts',(-5.97047727161498,-3.70282940005589,
18.9505847048781));
#77614=CARTESIAN_POINT('Ctrl Pts',(-6.19440298925313,-3.31464917833267,
18.9300080082272));
#77615=CARTESIAN_POINT('Ctrl Pts',(-6.44880809220584,-2.75647615086778,
18.9018250263312));
#77616=CARTESIAN_POINT('Ctrl Pts',(-6.51237863114435,-2.60273185054225,
18.8942076656584));
#77617=CARTESIAN_POINT('Ctrl Pts',(-6.65046309758209,-2.23194254520588,
18.8762599453689));
#77618=CARTESIAN_POINT('Ctrl Pts',(-6.71991072903908,-2.01321378874463,
18.865991669355));
#77619=CARTESIAN_POINT('Ctrl Pts',(-6.83706346274827,-1.56993525329702,
18.8454543787509));
#77620=CARTESIAN_POINT('Ctrl Pts',(-6.88471681233285,-1.34566219767677,
18.8351972394528));
#77621=CARTESIAN_POINT('Ctrl Pts',(-6.93728882573627,-1.02062451566611,
18.8203517590086));
#77622=CARTESIAN_POINT('Ctrl Pts',(-6.95115568489195,-0.921458118086937,
18.8158259878938));
#77623=CARTESIAN_POINT('Ctrl Pts',(-7.01323504839045,-0.395622882039393,
18.7918147907539));
#77624=CARTESIAN_POINT('Ctrl Pts',(-7.02429911688816,0.0345009806129306,
18.7720628725));
#77625=CARTESIAN_POINT('Ctrl Pts',(-6.98755142286396,0.589862748977917,
18.7464806984229));
#77626=CARTESIAN_POINT('Ctrl Pts',(-6.97569749796841,0.716559743081308,
18.7406447006897));
#77627=CARTESIAN_POINT('Ctrl Pts',(-6.94460089884169,0.973356402409076,
18.7288464105356));
#77628=CARTESIAN_POINT('Ctrl Pts',(-6.92513284087342,1.1033766193804,18.7228976715111));
#77629=CARTESIAN_POINT('Ctrl Pts',(-6.85429960972639,1.49995522653845,18.7047562101925));
#77630=CARTESIAN_POINT('Ctrl Pts',(-6.79110456959091,1.76413981815084,18.6926508731029));
#77631=CARTESIAN_POINT('Ctrl Pts',(-6.67031407091704,2.16475174188527,18.6738737089538));
#77632=CARTESIAN_POINT('Ctrl Pts',(-6.6234614295815,2.30412468515178,18.6672617016403));
#77633=CARTESIAN_POINT('Ctrl Pts',(-6.57226799068689,2.44190909353574,18.6606197598975));
#77634=CARTESIAN_POINT('',(-5.31040820991542,4.5779024898487,19.999999977237));
#77635=CARTESIAN_POINT('Origin',(0.,0.,20.));
#77636=CARTESIAN_POINT('',(-7.01125027639237,-0.000179547635693209,18.226489882947));
#77637=CARTESIAN_POINT('Ctrl Pts',(-5.31040820991542,4.5779024898487,19.999999977237));
#77638=CARTESIAN_POINT('Ctrl Pts',(-5.18798945140932,4.71990935470875,19.9914851839));
#77639=CARTESIAN_POINT('Ctrl Pts',(-5.05984933106507,4.85702836085778,19.9829703905629));
#77640=CARTESIAN_POINT('Ctrl Pts',(-4.92640288943302,4.98880558184883,19.9744555972259));
#77641=CARTESIAN_POINT('Ctrl Pts',(-4.79298172464453,5.12055784217282,19.9659424167239));
#77642=CARTESIAN_POINT('Ctrl Pts',(-4.6542564637124,5.24697011976722,19.9574292362219));
#77643=CARTESIAN_POINT('Ctrl Pts',(-4.51067912035527,5.36762521378784,19.9489160557199));
#77644=CARTESIAN_POINT('Ctrl Pts',(-4.36709695434415,5.48828436052151,19.9404025892667));
#77645=CARTESIAN_POINT('Ctrl Pts',(-4.2186626136012,5.60318573534523,19.9318891228134));
#77646=CARTESIAN_POINT('Ctrl Pts',(-4.06586200678471,5.71195174211798,19.9233756563602));
#77647=CARTESIAN_POINT('Ctrl Pts',(-3.91306982999273,5.82071174825943,19.9148626595957));
#77648=CARTESIAN_POINT('Ctrl Pts',(-3.75591212076988,5.92333688501612,19.9063496628312));
#77649=CARTESIAN_POINT('Ctrl Pts',(-3.59490490813367,6.01949211013491,19.8978366660668));
#77650=CARTESIAN_POINT('Ctrl Pts',(-3.43385658166986,6.11567188887018,19.889321495475));
#77651=CARTESIAN_POINT('Ctrl Pts',(-3.26895705176141,6.20537829485712,19.8808063248831));
#77652=CARTESIAN_POINT('Ctrl Pts',(-3.10074907371748,6.28832105926059,19.8722911542913));
#77653=CARTESIAN_POINT('Ctrl Pts',(-2.94870341965684,6.36329423835694,19.8645941669241));
#77654=CARTESIAN_POINT('Ctrl Pts',(-2.79395503517537,6.4327416004527,19.8568971795569));
#77655=CARTESIAN_POINT('Ctrl Pts',(-2.63692048472963,6.49648188789235,19.8492001921897));
#77656=CARTESIAN_POINT('Ctrl Pts',(-2.46287341495907,6.56712755296231,19.8406693428096));
#77657=CARTESIAN_POINT('Ctrl Pts',(-2.28595593848525,6.63078694304454,19.8321384934295));
#77658=CARTESIAN_POINT('Ctrl Pts',(-2.10674665552219,6.68724495528211,19.8236076440493));
#77659=CARTESIAN_POINT('Ctrl Pts',(-1.92757135827927,6.74369226067363,19.815078412482));
#77660=CARTESIAN_POINT('Ctrl Pts',(-1.7461054138216,6.79294082162602,19.8065491809146));
#77661=CARTESIAN_POINT('Ctrl Pts',(-1.5629435514884,6.83482509047312,19.7980199493472));
#77662=CARTESIAN_POINT('Ctrl Pts',(-1.37036403797662,6.87886292681973,19.789052169456));
#77663=CARTESIAN_POINT('Ctrl Pts',(-1.17590996346703,6.91475912243078,19.7800843895647));
#77664=CARTESIAN_POINT('Ctrl Pts',(-0.980286876873871,6.94238173838985,
19.7711166096734));
#77665=CARTESIAN_POINT('Ctrl Pts',(-0.794236169154417,6.96865270332425,
19.7625876480642));
#77666=CARTESIAN_POINT('Ctrl Pts',(-0.607128448303999,6.98744038349346,
19.7540586864549));
#77667=CARTESIAN_POINT('Ctrl Pts',(-0.419578243030414,6.99868420922644,
19.7455297248456));
#77668=CARTESIAN_POINT('Ctrl Pts',(-0.232026111967852,7.00992815041243,
19.7370006756599));
#77669=CARTESIAN_POINT('Ctrl Pts',(-0.0440317932571628,7.01362806729796,
19.7284716264742));
#77670=CARTESIAN_POINT('Ctrl Pts',(0.143787428283975,7.00977544133673,19.7199425772885));
#77671=CARTESIAN_POINT('Ctrl Pts',(0.331644731820408,7.00592203422177,19.7114117987632));
#77672=CARTESIAN_POINT('Ctrl Pts',(0.519326561139531,6.99451303291472,19.7028810202379));
#77673=CARTESIAN_POINT('Ctrl Pts',(0.70621711009679,6.97559201472582,19.6943502417127));
#77674=CARTESIAN_POINT('Ctrl Pts',(0.735016010041088,6.97267638034673,19.6930356913592));
#77675=CARTESIAN_POINT('Ctrl Pts',(0.763796129616165,6.96958247142347,19.6917211410057));
#77676=CARTESIAN_POINT('Ctrl Pts',(0.792555226703233,6.96631055689634,19.6904065906522));
#77677=CARTESIAN_POINT('Ctrl Pts',(0.979182207176351,6.94507805690804,19.6818760529093));
#77678=CARTESIAN_POINT('Ctrl Pts',(1.16498755152204,6.91633800535125,19.6733455151664));
#77679=CARTESIAN_POINT('Ctrl Pts',(1.34936030466879,6.88017829207094,19.6648149774235));
#77680=CARTESIAN_POINT('Ctrl Pts',(1.53369791849532,6.84402547041491,19.6562860655027));
#77681=CARTESIAN_POINT('Ctrl Pts',(1.71660318558908,6.80045586793386,19.6477571535819));
#77682=CARTESIAN_POINT('Ctrl Pts',(1.89747469270541,6.74960860739662,19.6392282416612));
#77683=CARTESIAN_POINT('Ctrl Pts',(2.08765656171744,6.69614398382329,19.6302603039489));
#77684=CARTESIAN_POINT('Ctrl Pts',(2.27558941965171,6.63463278937865,19.6212923662367));
#77685=CARTESIAN_POINT('Ctrl Pts',(2.46059050773937,6.56529671193336,19.6123244285245));
#77686=CARTESIAN_POINT('Ctrl Pts',(2.6365289878981,6.4993571857825,19.6037958012199));
#77687=CARTESIAN_POINT('Ctrl Pts',(2.80981574927779,6.42634117637166,19.5952671739153));
#77688=CARTESIAN_POINT('Ctrl Pts',(2.97988221300527,6.34648946734451,19.5867385466107));
#77689=CARTESIAN_POINT('Ctrl Pts',(3.14995034945622,6.26663697291956,19.5782098354211));
#77690=CARTESIAN_POINT('Ctrl Pts',(3.31679784912225,6.17994877762485,19.5696811242314));
#77691=CARTESIAN_POINT('Ctrl Pts',(3.47987861391564,6.08671269199661,19.5611524130417));
#77692=CARTESIAN_POINT('Ctrl Pts',(3.6429923841662,5.99345773657931,19.5526219757502));
#77693=CARTESIAN_POINT('Ctrl Pts',(3.80233763150214,5.89365239680338,19.5440915384587));
#77694=CARTESIAN_POINT('Ctrl Pts',(3.95739447931174,5.78762952318244,19.5355611011672));
#77695=CARTESIAN_POINT('Ctrl Pts',(3.98131594971838,5.77127279292784,19.5342450638163));
#77696=CARTESIAN_POINT('Ctrl Pts',(4.00513540809726,5.75476816370005,19.5329290264655));
#77697=CARTESIAN_POINT('Ctrl Pts',(4.02885100789913,5.73811694884744,19.5316129891146));
#77698=CARTESIAN_POINT('Ctrl Pts',(4.18258888964484,5.63017439115037,19.5230816934143));
#77699=CARTESIAN_POINT('Ctrl Pts',(4.33201243443761,5.51603136176059,19.514550397714));
#77700=CARTESIAN_POINT('Ctrl Pts',(4.47662714238184,5.3960574487852,19.5060191020136));
#77701=CARTESIAN_POINT('Ctrl Pts',(4.62121448336393,5.27610623973516,19.4974894207801));
#77702=CARTESIAN_POINT('Ctrl Pts',(4.76099456804004,5.15032654452421,19.4889597395466));
#77703=CARTESIAN_POINT('Ctrl Pts',(4.8955057910262,5.01912837179215,19.4804300583131));
#77704=CARTESIAN_POINT('Ctrl Pts',(5.03692220244502,4.88119508741199,19.4714625024185));
#77705=CARTESIAN_POINT('Ctrl Pts',(5.17251429392865,4.73727261406377,19.4624949465238));
#77706=CARTESIAN_POINT('Ctrl Pts',(5.30178872069088,4.58788218284373,19.4535273906291));
#77707=CARTESIAN_POINT('Ctrl Pts',(5.42474695774191,4.44579078460535,19.4449979785011));
#77708=CARTESIAN_POINT('Ctrl Pts',(5.54198992424946,4.29875324043526,19.4364685663731));
#77709=CARTESIAN_POINT('Ctrl Pts',(5.65313348451946,4.14725311124181,19.4279391542451));
#77710=CARTESIAN_POINT('Ctrl Pts',(5.7642781654629,3.99575145445495,19.4194096561141));
#77711=CARTESIAN_POINT('Ctrl Pts',(5.86932313880391,3.83978737149075,19.4108801579831));
#77712=CARTESIAN_POINT('Ctrl Pts',(5.96792650977962,3.67987496205641,19.402350659852));
#77713=CARTESIAN_POINT('Ctrl Pts',(6.06654981684823,3.51993022077966,19.3938194371869));
#77714=CARTESIAN_POINT('Ctrl Pts',(6.15872876038105,3.35603581968886,19.3852882145219));
#77715=CARTESIAN_POINT('Ctrl Pts',(6.24416602015155,3.18873286358151,19.3767569918568));
#77716=CARTESIAN_POINT('Ctrl Pts',(6.2573106041863,3.16299318312217,19.3754444570969));
#77717=CARTESIAN_POINT('Ctrl Pts',(6.27029570105889,3.13717286887965,19.374131922337));
#77718=CARTESIAN_POINT('Ctrl Pts',(6.28312032557758,3.11127394113953,19.3728193875771));
#77719=CARTESIAN_POINT('Ctrl Pts',(6.36647279498715,2.94294623851925,19.3642886884315));
#77720=CARTESIAN_POINT('Ctrl Pts',(6.44307130431841,2.77123815692641,19.3557579892859));
#77721=CARTESIAN_POINT('Ctrl Pts',(6.51265843964136,2.5967107291857,19.3472272901403));
#77722=CARTESIAN_POINT('Ctrl Pts',(6.58223233947808,2.42221649659459,19.3386982135353));
#77723=CARTESIAN_POINT('Ctrl Pts',(6.6447974132034,2.24490427231277,19.3301691369303));
#77724=CARTESIAN_POINT('Ctrl Pts',(6.70014446921764,2.06535484944168,19.3216400603253));
#77725=CARTESIAN_POINT('Ctrl Pts',(6.75833886257202,1.87656848041739,19.3126722041348));
#77726=CARTESIAN_POINT('Ctrl Pts',(6.80855287612425,1.68530900095786,19.3037043479443));
#77727=CARTESIAN_POINT('Ctrl Pts',(6.85060260265691,1.49227026472099,19.2947364917539));
#77728=CARTESIAN_POINT('Ctrl Pts',(6.89059360966207,1.30868254395132,19.2862076943203));
#77729=CARTESIAN_POINT('Ctrl Pts',(6.92320057024404,1.12348594464433,19.2776788968867));
#77730=CARTESIAN_POINT('Ctrl Pts',(6.94831751475442,0.937288790425337,19.2691500994531));
#77731=CARTESIAN_POINT('Ctrl Pts',(6.97343470978042,0.751089779081735,19.2606212169536));
#77732=CARTESIAN_POINT('Ctrl Pts',(6.99106170173282,0.563890496800545,19.252092334454));
#77733=CARTESIAN_POINT('Ctrl Pts',(7.0011442243662,0.376305875749824,19.2435634519545));
#77734=CARTESIAN_POINT('Ctrl Pts',(7.01122878832538,0.188683275976775,19.2350328426819));
#77735=CARTESIAN_POINT('Ctrl Pts',(7.01376581664533,0.000675487465281344,
19.2265022334094));
#77736=CARTESIAN_POINT('Ctrl Pts',(7.00875310516585,-0.187100169235761,
19.2179716241368));
#77737=CARTESIAN_POINT('Ctrl Pts',(7.00798022766499,-0.216052080964084,
19.2166563447711));
#77738=CARTESIAN_POINT('Ctrl Pts',(7.00702797435457,-0.244998475659424,
19.2153410654053));
#77739=CARTESIAN_POINT('Ctrl Pts',(7.00589644736758,-0.273937093622513,
19.2140257860396));
#77740=CARTESIAN_POINT('Ctrl Pts',(6.99855724805962,-0.461635917751245,
19.2054947500839));
#77741=CARTESIAN_POINT('Ctrl Pts',(6.98366933982935,-0.649071725155701,
19.1969637141282));
#77742=CARTESIAN_POINT('Ctrl Pts',(6.96127512095335,-0.835628657296986,
19.1884326781726));
#77743=CARTESIAN_POINT('Ctrl Pts',(6.9388851500791,-1.02215020110084,19.1799032604852));
#77744=CARTESIAN_POINT('Ctrl Pts',(6.90899174655451,-1.20779289846891,19.1713738427979));
#77745=CARTESIAN_POINT('Ctrl Pts',(6.87168910763913,-1.39194661192652,19.1628444251106));
#77746=CARTESIAN_POINT('Ctrl Pts',(6.83246973865202,-1.58556273798198,19.1538767383932));
#77747=CARTESIAN_POINT('Ctrl Pts',(6.78505972286755,-1.77753247551099,19.1449090516758));
#77748=CARTESIAN_POINT('Ctrl Pts',(6.72962952354261,-1.9671586205397,19.1359413649585));
#77749=CARTESIAN_POINT('Ctrl Pts',(6.67691000526172,-2.14751155343776,19.1274122214664));
#77750=CARTESIAN_POINT('Ctrl Pts',(6.61693607122333,-2.32574431516057,19.1188830779744));
#77751=CARTESIAN_POINT('Ctrl Pts',(6.54990572828462,-2.50127197903073,19.1103539344824));
#77752=CARTESIAN_POINT('Ctrl Pts',(6.48287471454436,-2.67680139948192,19.1018247056355));
#77753=CARTESIAN_POINT('Ctrl Pts',(6.40878726305569,-2.84962538310911,19.0932954767887));
#77754=CARTESIAN_POINT('Ctrl Pts',(6.32788994435908,-3.01917793688601,19.0847662479419));
#77755=CARTESIAN_POINT('Ctrl Pts',(6.24697626283045,-3.18876478549493,19.0762352939162));
#77756=CARTESIAN_POINT('Ctrl Pts',(6.1592500956831,-3.35507860668506,19.0677043398906));
#77757=CARTESIAN_POINT('Ctrl Pts',(6.06500487318369,-3.51757621818748,19.0591733858649));
#77758=CARTESIAN_POINT('Ctrl Pts',(6.0504914749463,-3.5426002192542,19.0578596520773));
#77759=CARTESIAN_POINT('Ctrl Pts',(6.03582356627391,-3.56753376894369,19.0565459182897));
#77760=CARTESIAN_POINT('Ctrl Pts',(6.02100231375902,-3.59237493870121,19.0552321845021));
#77761=CARTESIAN_POINT('Ctrl Pts',(5.92475871613629,-3.75368408205597,19.0467012950977));
#77762=CARTESIAN_POINT('Ctrl Pts',(5.82201244059844,-3.91115091479425,19.0381704056934));
#77763=CARTESIAN_POINT('Ctrl Pts',(5.71309534362803,-4.06425493259413,19.029639516289));
#77764=CARTESIAN_POINT('Ctrl Pts',(5.60419892977575,-4.21732987627641,19.0211102468818));
#77765=CARTESIAN_POINT('Ctrl Pts',(5.48913421041692,-4.36604340895412,19.0125809774747));
#77766=CARTESIAN_POINT('Ctrl Pts',(5.36827579144815,-4.50990483152935,19.0040517080675));
#77767=CARTESIAN_POINT('Ctrl Pts',(5.24120402305307,-4.66116219139263,18.9950839476423));
#77768=CARTESIAN_POINT('Ctrl Pts',(5.10772737401113,-4.80705511621083,18.986116187217));
#77769=CARTESIAN_POINT('Ctrl Pts',(4.96832911193144,-4.94705290026643,18.9771484267918));
#77770=CARTESIAN_POINT('Ctrl Pts',(4.83575121102563,-5.08020099024009,18.9686194334222));
#77771=CARTESIAN_POINT('Ctrl Pts',(4.69781753508435,-5.20801678046617,18.9600904400527));
#77772=CARTESIAN_POINT('Ctrl Pts',(4.55498178807121,-5.33008137581779,18.9515614466831));
#77773=CARTESIAN_POINT('Ctrl Pts',(4.41214461187468,-5.45214719252117,18.9430323679743));
#77774=CARTESIAN_POINT('Ctrl Pts',(4.26440550148309,-5.56846150289737,18.9345032892655));
#77775=CARTESIAN_POINT('Ctrl Pts',(4.11225174759387,-5.67864527214997,18.9259742105567));
#77776=CARTESIAN_POINT('Ctrl Pts',(3.96006720244786,-5.7888513392207,18.9174434058238));
#77777=CARTESIAN_POINT('Ctrl Pts',(3.80346647799771,-5.89292420839794,18.9089126010908));
#77778=CARTESIAN_POINT('Ctrl Pts',(3.6429671003538,-5.99052729467447,18.9003817963578));
#77779=CARTESIAN_POINT('Ctrl Pts',(3.61823776881749,-6.00556572731472,18.8990673918934));
#77780=CARTESIAN_POINT('Ctrl Pts',(3.59341593729415,-6.02045065357043,18.897752987429));
#77781=CARTESIAN_POINT('Ctrl Pts',(3.56850355590312,-6.03518093631059,18.8964385829646));
#77782=CARTESIAN_POINT('Ctrl Pts',(3.40681370596188,-6.13078549407908,18.8879076498001));
#77783=CARTESIAN_POINT('Ctrl Pts',(3.24125192648159,-6.21990487450771,18.8793767166356));
#77784=CARTESIAN_POINT('Ctrl Pts',(3.07235866038221,-6.30224077804668,18.8708457834711));
#77785=CARTESIAN_POINT('Ctrl Pts',(2.90349745789746,-6.3845610504907,18.8623164698653));
#77786=CARTESIAN_POINT('Ctrl Pts',(2.73130630606696,-6.46010028189103,18.8537871562595));
#77787=CARTESIAN_POINT('Ctrl Pts',(2.55634892730108,-6.52860679811448,18.8452578426536));
#77788=CARTESIAN_POINT('Ctrl Pts',(2.37239836777744,-6.60063469473256,18.8362901042181));
#77789=CARTESIAN_POINT('Ctrl Pts',(2.18539004318896,-6.66488769423388,18.8273223657825));
#77790=CARTESIAN_POINT('Ctrl Pts',(1.99600222015603,-6.72113098366876,18.818354627347));
#77791=CARTESIAN_POINT('Ctrl Pts',(1.81587922292988,-6.77462285925311,18.8098255894211));
#77792=CARTESIAN_POINT('Ctrl Pts',(1.63360429009838,-6.82086986851293,18.8012965514952));
#77793=CARTESIAN_POINT('Ctrl Pts',(1.44977624868172,-6.85972123276583,18.7927675135693));
#77794=CARTESIAN_POINT('Ctrl Pts',(1.26594636924264,-6.89857298547785,18.784238390365));
#77795=CARTESIAN_POINT('Ctrl Pts',(1.08056365043727,-6.9300288852799,18.7757092671606));
#77796=CARTESIAN_POINT('Ctrl Pts',(0.894237342332065,-6.95398922476005,
18.7671801439563));
#77797=CARTESIAN_POINT('Ctrl Pts',(0.707873335172129,-6.97795441209104,
18.7586492950704));
#77798=CARTESIAN_POINT('Ctrl Pts',(0.520565661225884,-6.99442097193293,
18.7501184461845));
#77799=CARTESIAN_POINT('Ctrl Pts',(0.332929811888472,-7.00334093864178,
18.7415875972986));
#77800=CARTESIAN_POINT('Ctrl Pts',(0.304023893006349,-7.00471508881099,
18.740273392008));
#77801=CARTESIAN_POINT('Ctrl Pts',(0.275110191864145,-7.00591024057634,
18.7389591867175));
#77802=CARTESIAN_POINT('Ctrl Pts',(0.246190963911276,-7.00692632841166,
18.737644981427));
#77803=CARTESIAN_POINT('Ctrl Pts',(0.0584668930673313,-7.01352208349517,
18.7291140494303));
#77804=CARTESIAN_POINT('Ctrl Pts',(-0.129554522942743,-7.01257059255586,
18.7205831174336));
#77805=CARTESIAN_POINT('Ctrl Pts',(-0.31725599199883,-7.00406847468247,
18.7120521854369));
#77806=CARTESIAN_POINT('Ctrl Pts',(-0.504921828007146,-6.99556797084212,
18.7035228729433));
#77807=CARTESIAN_POINT('Ctrl Pts',(-0.692267532516735,-6.97951971442561,
18.6949935604497));
#77808=CARTESIAN_POINT('Ctrl Pts',(-0.878677678046428,-6.95597240510649,
18.6864642479561));
#77809=CARTESIAN_POINT('Ctrl Pts',(-1.07466973887797,-6.93121470928806,
18.6774965089506));
#77810=CARTESIAN_POINT('Ctrl Pts',(-1.26962716618774,-6.89816674783037,
18.668528769945));
#77811=CARTESIAN_POINT('Ctrl Pts',(-1.46284201475234,-6.85694682802597,
18.6595610309395));
#77812=CARTESIAN_POINT('Ctrl Pts',(-1.64660478770015,-6.81774338781308,
18.6510319939686));
#77813=CARTESIAN_POINT('Ctrl Pts',(-1.82879107709652,-6.77114849393829,
18.6425029569977));
#77814=CARTESIAN_POINT('Ctrl Pts',(-2.00880290052994,-6.71731624008596,
18.6339739200268));
#77815=CARTESIAN_POINT('Ctrl Pts',(-2.18881652506152,-6.66348344761803,
18.6254447977191));
#77816=CARTESIAN_POINT('Ctrl Pts',(-2.36665534772529,-6.60241324131081,
18.6169156754114));
#77817=CARTESIAN_POINT('Ctrl Pts',(-2.5417366673616,-6.53430954855137,18.6083865531037));
#77818=CARTESIAN_POINT('Ctrl Pts',(-2.7168534126708,-6.46619207580016,18.5998557050271));
#77819=CARTESIAN_POINT('Ctrl Pts',(-2.88921125551704,-6.39103838602187,
18.5913248569505));
#77820=CARTESIAN_POINT('Ctrl Pts',(-3.05824676884958,-6.30910082843198,
18.582794008874));
#77821=CARTESIAN_POINT('Ctrl Pts',(-3.08428733395646,-6.29647803538067,
18.5814797992125));
#77822=CARTESIAN_POINT('Ctrl Pts',(-3.11024909430534,-6.28369433482796,
18.580165589551));
#77823=CARTESIAN_POINT('Ctrl Pts',(-3.13613003795766,-6.27075074831712,
18.5788513798895));
#77824=CARTESIAN_POINT('Ctrl Pts',(-3.30413086052554,-6.18673011869823,
18.5703204581765));
#77825=CARTESIAN_POINT('Ctrl Pts',(-3.46878197991479,-6.09593981105469,
18.5617895364636));
#77826=CARTESIAN_POINT('Ctrl Pts',(-3.62953971911893,-5.99867218556224,
18.5532586147506));
#77827=CARTESIAN_POINT('Ctrl Pts',(-3.79026693713249,-5.90142302713552,
18.5447293127039));
#77828=CARTESIAN_POINT('Ctrl Pts',(-3.94710198822778,-5.79769916344609,
18.5362000106572));
#77829=CARTESIAN_POINT('Ctrl Pts',(-4.09952774958241,-5.68783779593826,
18.5276707086105));
#77830=CARTESIAN_POINT('Ctrl Pts',(-4.25978883871199,-5.57232909023393,
18.5187029644223));
#77831=CARTESIAN_POINT('Ctrl Pts',(-4.41517508286484,-5.45003547304751,
18.509735220234));
#77832=CARTESIAN_POINT('Ctrl Pts',(-4.56512141629977,-5.32139953554901,
18.5007674760458));
#77833=CARTESIAN_POINT('Ctrl Pts',(-4.70773211005469,-5.19905669549259,
18.4922384497549));
#77834=CARTESIAN_POINT('Ctrl Pts',(-4.84542218018709,-5.07097747392741,
18.483709423464));
#77835=CARTESIAN_POINT('Ctrl Pts',(-4.97774024638283,-4.93758327545376,
18.475180397173));
#77836=CARTESIAN_POINT('Ctrl Pts',(-5.11005963591569,-4.80418774288039,
18.4666512855817));
#77837=CARTESIAN_POINT('Ctrl Pts',(-5.23700670082084,-4.66547734685421,
18.4581221739904));
#77838=CARTESIAN_POINT('Ctrl Pts',(-5.35816732152366,-4.521909941281,18.4495930623992));
#77839=CARTESIAN_POINT('Ctrl Pts',(-5.47935245785444,-4.37831348629323,
18.4410622250283));
#77840=CARTESIAN_POINT('Ctrl Pts',(-5.59474861470344,-4.22985829349008,
18.4325313876574));
#77841=CARTESIAN_POINT('Ctrl Pts',(-5.70398176399658,-4.07703551597169,
18.4240005502865));
#77842=CARTESIAN_POINT('Ctrl Pts',(-5.72081017823964,-4.05349170145661,
18.422686292975));
#77843=CARTESIAN_POINT('Ctrl Pts',(-5.73749239856006,-4.02984428476107,
18.4213720356635));
#77844=CARTESIAN_POINT('Ctrl Pts',(-5.75402714681736,-4.00609512570394,
18.420057778352));
#77845=CARTESIAN_POINT('Ctrl Pts',(-5.86135529224486,-3.85193776222923,
18.411526847148));
#77846=CARTESIAN_POINT('Ctrl Pts',(-5.96250314914113,-3.69343835465417,
18.402995915944));
#77847=CARTESIAN_POINT('Ctrl Pts',(-6.05713317387302,-3.53111374448161,
18.39446498474));
#77848=CARTESIAN_POINT('Ctrl Pts',(-6.15174523378733,-3.3688199504482,18.3859356730708));
#77849=CARTESIAN_POINT('Ctrl Pts',(-6.23984177667961,-3.20270266741765,
18.3774063614017));
#77850=CARTESIAN_POINT('Ctrl Pts',(-6.32113003023968,-3.03330540884069,
18.3688770497325));
#77851=CARTESIAN_POINT('Ctrl Pts',(-6.40659670132452,-2.85520071169926,
18.3599093103227));
#77852=CARTESIAN_POINT('Ctrl Pts',(-6.48453655148899,-2.67347028005893,
18.3509415709129));
#77853=CARTESIAN_POINT('Ctrl Pts',(-6.55466513137106,-2.48877310699236,
18.341973831503));
#77854=CARTESIAN_POINT('Ctrl Pts',(-6.62136300926237,-2.31311135087554,
18.3334447954221));
#77855=CARTESIAN_POINT('Ctrl Pts',(-6.68099549066131,-2.134766492544,18.3249157593412));
#77856=CARTESIAN_POINT('Ctrl Pts',(-6.7333678186597,-1.95432453321805,18.3163867232603));
#77857=CARTESIAN_POINT('Ctrl Pts',(-6.78574067054998,-1.77388076889159,
18.3078576018615));
#77858=CARTESIAN_POINT('Ctrl Pts',(-6.83085314168356,-1.59134015661709,
18.2993284804628));
#77859=CARTESIAN_POINT('Ctrl Pts',(-6.8685606331945,-1.40730287807238,18.290799359064));
#77860=CARTESIAN_POINT('Ctrl Pts',(-6.90627575428454,-1.22322836217992,
18.2822685119179));
#77861=CARTESIAN_POINT('Ctrl Pts',(-6.93658284265557,-1.03765687534071,
18.2737376647717));
#77862=CARTESIAN_POINT('Ctrl Pts',(-6.95938843614138,-0.851198659186938,
18.2652068176255));
#77863=CARTESIAN_POINT('Ctrl Pts',(-6.96290173566313,-0.822473971006945,
18.2638926040219));
#77864=CARTESIAN_POINT('Ctrl Pts',(-6.96623710401648,-0.79372825189046,
18.2625783904182));
#77865=CARTESIAN_POINT('Ctrl Pts',(-6.96939430864683,-0.764963746265907,
18.2612641768145));
#77866=CARTESIAN_POINT('Ctrl Pts',(-6.99107740060903,-0.567414491869339,
18.2522384031436));
#77867=CARTESIAN_POINT('Ctrl Pts',(-7.00435755886076,-0.368935936278,18.2432126294727));
#77868=CARTESIAN_POINT('Ctrl Pts',(-7.00918342474411,-0.170218332715454,
18.2341868558018));
#77869=CARTESIAN_POINT('Ctrl Pts',(-7.0105595408299,-0.113553166836021,
18.2316131182311));
#77870=CARTESIAN_POINT('Ctrl Pts',(-7.01124853702015,-0.0568685892723279,
18.2290393806603));
#77871=CARTESIAN_POINT('Ctrl Pts',(-7.01124999767256,-0.000180655715778411,
18.2264656430896));
#77872=CARTESIAN_POINT('Ctrl Pts',(-7.01124999770178,-0.00017951820933601,
18.2264903645786));
#77873=CARTESIAN_POINT('Ctrl Pts',(-7.01125577494277,0.225455981633749,
18.2161082295559));
#77874=CARTESIAN_POINT('Ctrl Pts',(-7.00036947495541,0.45096251588819,18.2057421677263));
#77875=CARTESIAN_POINT('Ctrl Pts',(-6.96472858178406,0.819141872311974,
18.1888528438194));
#77876=CARTESIAN_POINT('Ctrl Pts',(-6.94640026963132,0.962269013776619,
18.1822947481454));
#77877=CARTESIAN_POINT('Ctrl Pts',(-6.85270045561988,1.54951348992101,18.1553737625081));
#77878=CARTESIAN_POINT('Ctrl Pts',(-6.73903764732082,1.98641993334926,18.1353824772627));
#77879=CARTESIAN_POINT('Ctrl Pts',(-6.58028721034065,2.4202438351479,18.1145789804434));
#77880=CARTESIAN_POINT('Ctrl Pts',(-6.57629094993498,2.43108151336865,18.1140585918785));
#77881=CARTESIAN_POINT('Ctrl Pts',(-6.57226799602084,2.4419090791797,18.1135379835087));
#77882=CARTESIAN_POINT('Origin',(0.,0.,10.));
#77883=CARTESIAN_POINT('Ctrl Pts',(-6.57226799602084,2.4419090791797,18.1135379835087));
#77884=CARTESIAN_POINT('Ctrl Pts',(-6.53133773793476,2.55207068494202,18.1082412201375));
#77885=CARTESIAN_POINT('Ctrl Pts',(-6.48764442560255,2.6611854159813,18.1029188956554));
#77886=CARTESIAN_POINT('Ctrl Pts',(-6.30695942002566,3.08147038585748,18.0820569411487));
#77887=CARTESIAN_POINT('Ctrl Pts',(-6.15015392438222,3.38360801034555,18.0663501241534));
#77888=CARTESIAN_POINT('Ctrl Pts',(-5.86864123543347,3.84130686026723,18.0416943762633));
#77889=CARTESIAN_POINT('Ctrl Pts',(-5.75817549473653,4.00499751101801,18.0326790081895));
#77890=CARTESIAN_POINT('Ctrl Pts',(-5.39944115363625,4.4909951943229,18.0052513848175));
#77891=CARTESIAN_POINT('Ctrl Pts',(-5.12992452278029,4.79654896948932,17.9871027008005));
#77892=CARTESIAN_POINT('Ctrl Pts',(-4.69960032454455,5.20639762371295,17.9604604173751));
#77893=CARTESIAN_POINT('Ctrl Pts',(-4.55861995612133,5.33027220463726,17.952033971876));
#77894=CARTESIAN_POINT('Ctrl Pts',(-4.21508981287583,5.60851188158642,17.9319478743448));
#77895=CARTESIAN_POINT('Ctrl Pts',(-4.00876384610101,5.75779448881512,17.9202319016981));
#77896=CARTESIAN_POINT('Ctrl Pts',(-3.5436809163475,6.05715507631821,17.8947825417151));
#77897=CARTESIAN_POINT('Ctrl Pts',(-3.28250574277425,6.20257714731901,17.8810827646505));
#77898=CARTESIAN_POINT('Ctrl Pts',(-2.79124019713527,6.43636850206716,17.8563510001969));
#77899=CARTESIAN_POINT('Ctrl Pts',(-2.5642408750039,6.53012504120916,17.8452919196435));
#77900=CARTESIAN_POINT('Ctrl Pts',(-2.11497689976914,6.68863573172338,17.8239116387394));
#77901=CARTESIAN_POINT('Ctrl Pts',(-1.89349946819157,6.75467501023395,17.8135973338988));
#77902=CARTESIAN_POINT('Ctrl Pts',(-1.52228723506105,6.84566566269185,17.7964290318575));
#77903=CARTESIAN_POINT('Ctrl Pts',(-1.37428288747775,6.87690647911858,17.7896118758936));
#77904=CARTESIAN_POINT('Ctrl Pts',(-0.98282969575925,6.94639175307489,17.7715185702293));
#77905=CARTESIAN_POINT('Ctrl Pts',(-0.738177543202611,6.97663273517866,
17.7601749637869));
#77906=CARTESIAN_POINT('Ctrl Pts',(-0.183398802384542,7.01569486897031,
17.7345861519763));
#77907=CARTESIAN_POINT('Ctrl Pts',(0.126754820707417,7.0169472577802,17.7203819579545));
#77908=CARTESIAN_POINT('Ctrl Pts',(0.846874154652356,6.97208169737093,17.687618328165));
#77909=CARTESIAN_POINT('Ctrl Pts',(1.25471991553141,6.91034021910658,17.6692493842604));
#77910=CARTESIAN_POINT('Ctrl Pts',(1.83421043486687,6.76959301527378,17.642511571504));
#77911=CARTESIAN_POINT('Ctrl Pts',(2.01183802309883,6.7189451289178,17.6342161601171));
#77912=CARTESIAN_POINT('Ctrl Pts',(2.42641487902089,6.58281859570323,17.6143884008321));
#77913=CARTESIAN_POINT('Ctrl Pts',(2.66116811632201,6.49146912758555,17.602800622479));
#77914=CARTESIAN_POINT('Ctrl Pts',(3.15600305987535,6.26755131160755,17.5778092829768));
#77915=CARTESIAN_POINT('Ctrl Pts',(3.41376406077169,6.13096847145579,17.5644362120504));
#77916=CARTESIAN_POINT('Ctrl Pts',(3.86482288946793,5.85467229233321,17.5403776519203));
#77917=CARTESIAN_POINT('Ctrl Pts',(4.06093352070668,5.72039031683214,17.5296647633831));
#77918=CARTESIAN_POINT('Ctrl Pts',(4.45285995469801,5.42169838677391,17.5075367241649));
#77919=CARTESIAN_POINT('Ctrl Pts',(4.64726673012376,5.25601431003394,17.4961458788654));
#77920=CARTESIAN_POINT('Ctrl Pts',(4.88354866598726,5.03126229743105,17.4814921676409));
#77921=CARTESIAN_POINT('Ctrl Pts',(4.93414858539626,4.98164887497338,17.4783022024546));
#77922=CARTESIAN_POINT('Ctrl Pts',(5.07353905926242,4.84076846240518,17.4693521145051));
#77923=CARTESIAN_POINT('Ctrl Pts',(5.16060638394841,4.74783936484442,17.4635638527226));
#77924=CARTESIAN_POINT('Ctrl Pts',(5.42826320812631,4.44609673030629,17.4451170301998));
#77925=CARTESIAN_POINT('Ctrl Pts',(5.5990773457441,4.22896559385304,17.4323824610446));
#77926=CARTESIAN_POINT('Ctrl Pts',(5.90138954951528,3.79414303750813,17.4080568591738));
#77927=CARTESIAN_POINT('Ctrl Pts',(6.03473533685795,3.57825279917168,17.3964737812563));
#77928=CARTESIAN_POINT('Ctrl Pts',(6.29037366494197,3.10926715376298,17.3722594653965));
#77929=CARTESIAN_POINT('Ctrl Pts',(6.40974632530941,2.85508291359299,17.3596717378527));
#77930=CARTESIAN_POINT('Ctrl Pts',(6.60837584665915,2.35640389469369,17.3356250786124));
#77931=CARTESIAN_POINT('Ctrl Pts',(6.69006400772755,2.11336480498559,17.3241785838793));
#77932=CARTESIAN_POINT('Ctrl Pts',(6.79564330085926,1.73106141829922,17.3062202441551));
#77933=CARTESIAN_POINT('Ctrl Pts',(6.8289457084578,1.59462860734483,17.2998097485968));
#77934=CARTESIAN_POINT('Ctrl Pts',(6.91332233390364,1.19754536294385,17.2811943685785));
#77935=CARTESIAN_POINT('Ctrl Pts',(6.95371495757701,0.934873996140607,17.2689473466327));
#77936=CARTESIAN_POINT('Ctrl Pts',(6.99798936661613,0.474061066159394,17.2477059060085));
#77937=CARTESIAN_POINT('Ctrl Pts',(7.0085616606389,0.276865067678228,17.2386905353353));
#77938=CARTESIAN_POINT('Ctrl Pts',(7.01540315346882,-0.326580580999011,
17.2112891308239));
#77939=CARTESIAN_POINT('Ctrl Pts',(6.98471968828257,-0.732278758725528,
17.1931655772121));
#77940=CARTESIAN_POINT('Ctrl Pts',(6.88872141348215,-1.31850892653739,17.1665339124638));
#77941=CARTESIAN_POINT('Ctrl Pts',(6.85090468186664,-1.50268153047177,17.1580922539858));
#77942=CARTESIAN_POINT('Ctrl Pts',(6.7444976813099,-1.93243280045099,17.1379766420135));
#77943=CARTESIAN_POINT('Ctrl Pts',(6.66982445252792,-2.17623173407646,17.1262462788252));
#77944=CARTESIAN_POINT('Ctrl Pts',(6.47922635886562,-2.69561356648885,17.1007900355964));
#77945=CARTESIAN_POINT('Ctrl Pts',(6.35861599103292,-2.96895849518786,17.0870977161311));
#77946=CARTESIAN_POINT('Ctrl Pts',(6.10772186199823,-3.45161258521224,17.0623701269612));
#77947=CARTESIAN_POINT('Ctrl Pts',(5.98312763001639,-3.66334308149199,17.0513079683639));
#77948=CARTESIAN_POINT('Ctrl Pts',(5.72079747825706,-4.059925913999,17.029968743167));
#77949=CARTESIAN_POINT('Ctrl Pts',(5.5845505269411,-4.24538774841203,17.0196980445586));
#77950=CARTESIAN_POINT('Ctrl Pts',(5.34369734822726,-4.54153596251342,17.0025518482901));
#77951=CARTESIAN_POINT('Ctrl Pts',(5.24416405093607,-4.65611351135732,16.9957123191847));
#77952=CARTESIAN_POINT('Ctrl Pts',(4.97250429443794,-4.94906326508929,16.9775308935524));
#77953=CARTESIAN_POINT('Ctrl Pts',(4.79450538407557,-5.12169328135939,16.9661202686862));
#77954=CARTESIAN_POINT('Ctrl Pts',(4.3754672734317,-5.4870651028578,16.9405405962388));
#77955=CARTESIAN_POINT('Ctrl Pts',(4.13008625304336,-5.67406298365945,16.9264118914367));
#77956=CARTESIAN_POINT('Ctrl Pts',(3.52843577889293,-6.07279443747314,16.8936350917234));
#77957=CARTESIAN_POINT('Ctrl Pts',(3.16413259506985,-6.27032385217807,16.8751827475865));
#77958=CARTESIAN_POINT('Ctrl Pts',(2.66319233617672,-6.48710393375469,16.8507083923684));
#77959=CARTESIAN_POINT('Ctrl Pts',(2.54037925818996,-6.53617499077462,16.8447697234657));
#77960=CARTESIAN_POINT('Ctrl Pts',(2.29498709661735,-6.62626200791968,16.832955593691));
#77961=CARTESIAN_POINT('Ctrl Pts',(2.17251663596854,-6.66741960960383,16.8270757708442));
#77962=CARTESIAN_POINT('Ctrl Pts',(1.7874059135473,-6.78510259665264,16.8086451312496));
#77963=CARTESIAN_POINT('Ctrl Pts',(1.5213784048371,-6.84966018891278,16.7960269483759));
#77964=CARTESIAN_POINT('Ctrl Pts',(1.05714718378318,-6.93393037632997,16.7743603600334));
#77965=CARTESIAN_POINT('Ctrl Pts',(0.860616104300867,-6.96105539785072,
16.7652915256496));
#77966=CARTESIAN_POINT('Ctrl Pts',(0.421103786264986,-7.00281635562354,
16.7452193779524));
#77967=CARTESIAN_POINT('Ctrl Pts',(0.177974285219394,-7.0132084955377,16.7342586441171));
#77968=CARTESIAN_POINT('Ctrl Pts',(-0.373439342799838,-7.00808003194474,
16.7095072797542));
#77969=CARTESIAN_POINT('Ctrl Pts',(-0.681145051399979,-6.98488944475263,
16.6957761549718));
#77970=CARTESIAN_POINT('Ctrl Pts',(-1.11188518927663,-6.92368562289141,
16.6761375206015));
#77971=CARTESIAN_POINT('Ctrl Pts',(-1.23693917084852,-6.90244100766074,
16.670376238896));
#77972=CARTESIAN_POINT('Ctrl Pts',(-1.63347048804642,-6.82395433360602,
16.6518977433815));
#77973=CARTESIAN_POINT('Ctrl Pts',(-1.90215610330906,-6.75398993883881,
16.6390996309057));
#77974=CARTESIAN_POINT('Ctrl Pts',(-2.40957541225703,-6.5891705065465,16.6145901415609));
#77975=CARTESIAN_POINT('Ctrl Pts',(-2.64864766505702,-6.49676003461844,
16.6028879703152));
#77976=CARTESIAN_POINT('Ctrl Pts',(-3.18090903097595,-6.25674558791332,
16.5764155993003));
#77977=CARTESIAN_POINT('Ctrl Pts',(-3.46987517683895,-6.10123086062648,
16.5617436376327));
#77978=CARTESIAN_POINT('Ctrl Pts',(-3.94323687007113,-5.80193640726703,
16.5366577967459));
#77979=CARTESIAN_POINT('Ctrl Pts',(-4.1332767915154,-5.66812163071558,16.5262578023159));
#77980=CARTESIAN_POINT('Ctrl Pts',(-4.58211232271473,-5.31748371384333,
16.5004089646846));
#77981=CARTESIAN_POINT('Ctrl Pts',(-4.83257114760226,-5.09093681140747,
16.4848332158554));
#77982=CARTESIAN_POINT('Ctrl Pts',(-5.24816949750473,-4.65660461718289,
16.4572069757215));
#77983=CARTESIAN_POINT('Ctrl Pts',(-5.41968614758737,-4.45581145880002,
16.445143873667));
#77984=CARTESIAN_POINT('Ctrl Pts',(-5.72638183929998,-4.0527799460245,16.4221745402546));
#77985=CARTESIAN_POINT('Ctrl Pts',(-5.86316847114925,-3.85223731052618,
16.4112674976456));
#77986=CARTESIAN_POINT('Ctrl Pts',(-6.13392524450991,-3.40734379154622,
16.3879183058445));
#77987=CARTESIAN_POINT('Ctrl Pts',(-6.26428803646808,-3.16128498604509,
16.3755084088207));
#77988=CARTESIAN_POINT('Ctrl Pts',(-6.4328345428192,-2.79153832645471,16.3571500982043));
#77989=CARTESIAN_POINT('Ctrl Pts',(-6.48277698657554,-2.67350854187538,
16.3513209450489));
#77990=CARTESIAN_POINT('Ctrl Pts',(-6.6324184378392,-2.29096768202361,16.3325272908703));
#77991=CARTESIAN_POINT('Ctrl Pts',(-6.71937052319194,-2.02177319322608,
16.3194861559102));
#77992=CARTESIAN_POINT('Ctrl Pts',(-6.85147135246525,-1.50866756857715,
16.2951586814586));
#77993=CARTESIAN_POINT('Ctrl Pts',(-6.90040199395209,-1.26617269724376,
16.2838722597639));
#77994=CARTESIAN_POINT('Ctrl Pts',(-6.98624916328889,-0.683289388699604,
16.2571717977581));
#77995=CARTESIAN_POINT('Ctrl Pts',(-7.01125858868385,-0.341787511429588,
16.2418817111034));
#77996=CARTESIAN_POINT('Ctrl Pts',(-7.01124466201124,0.212568646146331,
16.2170454330908));
#77997=CARTESIAN_POINT('Ctrl Pts',(-7.00158828261392,0.424848241481843,
16.2075242251945));
#77998=CARTESIAN_POINT('Ctrl Pts',(-6.96549144408797,0.820913657941926,
16.1894710556958));
#77999=CARTESIAN_POINT('Ctrl Pts',(-6.94136090725623,1.0047273438697,16.1809707123927));
#78000=CARTESIAN_POINT('Ctrl Pts',(-6.8404564236361,1.59194968198766,16.1535746267476));
#78001=CARTESIAN_POINT('Ctrl Pts',(-6.73553476393021,1.9896563466863,16.134698335654));
#78002=CARTESIAN_POINT('Ctrl Pts',(-6.58847844020422,2.39794234569235,16.1150125326801));
#78003=CARTESIAN_POINT('Ctrl Pts',(-6.58042797879554,2.4199469208126,16.1139504014194));
#78004=CARTESIAN_POINT('Ctrl Pts',(-6.57226800013471,2.44190906810743,16.1128890894906));
#78005=CARTESIAN_POINT('',(-7.0112499981366,-0.00016164628603672,16.7735343569104));
#78006=CARTESIAN_POINT('Ctrl Pts',(-6.57226799596304,2.44190907933527,16.660297082902));
#78007=CARTESIAN_POINT('Ctrl Pts',(-6.58514542129488,2.40725017614552,16.6619761778387));
#78008=CARTESIAN_POINT('Ctrl Pts',(-6.59774827257987,2.37249050223351,16.6636552727754));
#78009=CARTESIAN_POINT('Ctrl Pts',(-6.61007499971753,2.33763450107353,16.6653343677121));
#78010=CARTESIAN_POINT('Ctrl Pts',(-6.67265846254533,2.16066869104471,16.6738592238545));
#78011=CARTESIAN_POINT('Ctrl Pts',(-6.72814251569491,1.98115620202462,16.6823840799969));
#78012=CARTESIAN_POINT('Ctrl Pts',(-6.77633856351089,1.79968392646465,16.6909089361393));
#78013=CARTESIAN_POINT('Ctrl Pts',(-6.82452658430392,1.61824187500369,16.6994323724719));
#78014=CARTESIAN_POINT('Ctrl Pts',(-6.86542894192989,1.43484098467328,16.7079558088046));
#78015=CARTESIAN_POINT('Ctrl Pts',(-6.89890725570808,1.25008209315963,16.7164792451373));
#78016=CARTESIAN_POINT('Ctrl Pts',(-6.93238090759436,1.0653489295243,16.7250014945722));
#78017=CARTESIAN_POINT('Ctrl Pts',(-6.95843252528074,0.879258444382991,
16.733523744007));
#78018=CARTESIAN_POINT('Ctrl Pts',(-6.97697497069008,0.69242098528582,16.7420459934418));
#78019=CARTESIAN_POINT('Ctrl Pts',(-6.99551756399199,0.505582035992998,
16.7505683108492));
#78020=CARTESIAN_POINT('Ctrl Pts',(-7.00655083429286,0.317996406289197,
16.7590906282566));
#78021=CARTESIAN_POINT('Ctrl Pts',(-7.01003949854652,0.130279665787652,
16.767612945664));
#78022=CARTESIAN_POINT('Ctrl Pts',(-7.01084748753039,0.0868036969395056,
16.7695867494128));
#78023=CARTESIAN_POINT('Ctrl Pts',(-7.01125100063413,0.0433207061692093,
16.7715605531616));
#78024=CARTESIAN_POINT('Ctrl Pts',(-7.0112499981366,-0.00016164628603672,
16.7735343569104));
#78025=CARTESIAN_POINT('Ctrl Pts',(-6.57226799068689,2.44190909353574,18.6606197598975));
#78026=CARTESIAN_POINT('Ctrl Pts',(-6.55458256276715,2.4895084788389,18.6583252162124));
#78027=CARTESIAN_POINT('Ctrl Pts',(-6.53637908263129,2.53691828524661,18.6560271977506));
#78028=CARTESIAN_POINT('Ctrl Pts',(-6.34950578661924,3.00824777710428,18.6330474945965));
#78029=CARTESIAN_POINT('Ctrl Pts',(-6.14035688537109,3.41493452497112,18.6120463439572));
#78030=CARTESIAN_POINT('Ctrl Pts',(-5.80529356625243,3.93478342108527,18.583636287599));
#78031=CARTESIAN_POINT('Ctrl Pts',(-5.71267994946519,4.06807616298501,18.576207268064));
#78032=CARTESIAN_POINT('Ctrl Pts',(-5.48133729766782,4.3775326923495,18.5586842567907));
#78033=CARTESIAN_POINT('Ctrl Pts',(-5.33861997283839,4.55049345230517,18.5486484067481));
#78034=CARTESIAN_POINT('Ctrl Pts',(-5.03271150353628,4.88698673714595,18.5282781650059));
#78035=CARTESIAN_POINT('Ctrl Pts',(-4.86923449019688,5.04988898793645,18.5179552406326));
#78036=CARTESIAN_POINT('Ctrl Pts',(-4.62367611942892,5.27155371416962,18.5030418091212));
#78037=CARTESIAN_POINT('Ctrl Pts',(-4.54789521056789,5.3370692648912,18.4985146599895));
#78038=CARTESIAN_POINT('Ctrl Pts',(-4.13498086892453,5.67886755600364,18.4742101598731));
#78039=CARTESIAN_POINT('Ctrl Pts',(-3.77404342110726,5.92487840940232,18.4541564401886));
#78040=CARTESIAN_POINT('Ctrl Pts',(-3.242360167737,6.21885906131579,18.4262355797459));
#78041=CARTESIAN_POINT('Ctrl Pts',(-3.08909591832835,6.29639546514875,18.4183677192841));
#78042=CARTESIAN_POINT('Ctrl Pts',(-2.77205432161874,6.44242143264674,18.4025303922832));
#78043=CARTESIAN_POINT('Ctrl Pts',(-2.60821163962649,6.51047715200553,18.3945656421109));
#78044=CARTESIAN_POINT('Ctrl Pts',(-2.06320144224783,6.7129793869552,18.3685009461884));
#78045=CARTESIAN_POINT('Ctrl Pts',(-1.67298773499486,6.82070373535555,18.3504665571867));
#78046=CARTESIAN_POINT('Ctrl Pts',(-1.08158271529183,6.93013475092709,18.3231586639686));
#78047=CARTESIAN_POINT('Ctrl Pts',(-0.886061138421088,6.95783606780917,
18.314143806508));
#78048=CARTESIAN_POINT('Ctrl Pts',(-0.425571818255266,7.00335100387356,
18.2929120378822));
#78049=CARTESIAN_POINT('Ctrl Pts',(-0.160241699369519,7.01443930242023,
18.2806741832081));
#78050=CARTESIAN_POINT('Ctrl Pts',(0.245827482243395,7.00835292333669,18.2620503839529));
#78051=CARTESIAN_POINT('Ctrl Pts',(0.386485679439094,7.00200487711029,18.2556228942669));
#78052=CARTESIAN_POINT('Ctrl Pts',(0.586026920853302,6.98696783929156,18.2465618493075));
#78053=CARTESIAN_POINT('Ctrl Pts',(0.645134947704559,6.9817582393844,18.2438834074806));
#78054=CARTESIAN_POINT('Ctrl Pts',(0.880753138408596,6.95797382925482,18.2332156076782));
#78055=CARTESIAN_POINT('Ctrl Pts',(1.05659691472483,6.93345005546821,18.2252730372193));
#78056=CARTESIAN_POINT('Ctrl Pts',(1.52729742197193,6.84948019116534,18.2038567245137));
#78057=CARTESIAN_POINT('Ctrl Pts',(1.81956694668522,6.77769789226068,18.1903810293141));
#78058=CARTESIAN_POINT('Ctrl Pts',(2.3485594573209,6.61108125147755,18.1652379015473));
#78059=CARTESIAN_POINT('Ctrl Pts',(2.58646861352615,6.52167948143408,18.15363616957));
#78060=CARTESIAN_POINT('Ctrl Pts',(3.07192843455,6.30850155802817,18.1292817568975));
#78061=CARTESIAN_POINT('Ctrl Pts',(3.31807333418695,6.18258247536715,18.1165372275004));
#78062=CARTESIAN_POINT('Ctrl Pts',(3.66578414484173,5.97794588678848,18.0980866228301));
#78063=CARTESIAN_POINT('Ctrl Pts',(3.77364609060732,5.91044893355489,18.0923037700712));
#78064=CARTESIAN_POINT('Ctrl Pts',(4.13696044959863,5.66909503045029,18.0726073341635));
#78065=CARTESIAN_POINT('Ctrl Pts',(4.38272739932649,5.48131230138458,18.0588444751542));
#78066=CARTESIAN_POINT('Ctrl Pts',(4.79977390069267,5.11662435263432,18.0339809489723));
#78067=CARTESIAN_POINT('Ctrl Pts',(4.97565379040086,4.9457598651466,18.0229388622396));
#78068=CARTESIAN_POINT('Ctrl Pts',(5.34582704617447,4.54636883134513,17.9981839042158));
#78069=CARTESIAN_POINT('Ctrl Pts',(5.53514067636744,4.31387863218984,17.9844428078976));
#78070=CARTESIAN_POINT('Ctrl Pts',(5.85572995542538,3.86418701494117,17.9590315263988));
#78071=CARTESIAN_POINT('Ctrl Pts',(5.99122114808128,3.65058713423913,17.9473952100159));
#78072=CARTESIAN_POINT('Ctrl Pts',(6.20573847891588,3.26816843022517,17.9274715867082));
#78073=CARTESIAN_POINT('Ctrl Pts',(6.29012433195544,3.10265249767159,17.919128472505));
#78074=CARTESIAN_POINT('Ctrl Pts',(6.53934905997762,2.56174114659309,17.8924263265319));
#78075=CARTESIAN_POINT('Ctrl Pts',(6.67788656577902,2.17518501476121,17.8741384016438));
#78076=CARTESIAN_POINT('Ctrl Pts',(6.80724963445372,1.6819606212768,17.8509845146513));
#78077=CARTESIAN_POINT('Ctrl Pts',(6.83056039668648,1.58463987738861,17.8464274245965));
#78078=CARTESIAN_POINT('Ctrl Pts',(6.87605250695625,1.37500134497382,17.8366293681007));
#78079=CARTESIAN_POINT('Ctrl Pts',(6.89758215531807,1.26257154065238,17.8313857131571));
#78080=CARTESIAN_POINT('Ctrl Pts',(6.96096076284132,0.881288036443326,17.813638932025));
#78081=CARTESIAN_POINT('Ctrl Pts',(6.98991291079394,0.610541472833123,17.8010883076366));
#78082=CARTESIAN_POINT('Ctrl Pts',(7.00937466701543,0.208262084983773,17.7826476501432));
#78083=CARTESIAN_POINT('Ctrl Pts',(7.01203894166487,0.0775724229597804,
17.7766950933235));
#78084=CARTESIAN_POINT('Ctrl Pts',(7.01007379652506,-0.18180591059101,17.7649676521403));
#78085=CARTESIAN_POINT('Ctrl Pts',(7.0055558984855,-0.310443448558691,17.7591853188952));
#78086=CARTESIAN_POINT('Ctrl Pts',(6.97092465084892,-0.862598097317044,
17.7343729716898));
#78087=CARTESIAN_POINT('Ctrl Pts',(6.90591976661297,-1.28301726522208,17.7154419265826));
#78088=CARTESIAN_POINT('Ctrl Pts',(6.72904978721014,-1.99294172322638,17.6822117280348));
#78089=CARTESIAN_POINT('Ctrl Pts',(6.63531696194163,-2.28571449999727,17.6681312389614));
#78090=CARTESIAN_POINT('Ctrl Pts',(6.42669735932324,-2.81490724271353,17.6419589531438));
#78091=CARTESIAN_POINT('Ctrl Pts',(6.31713590902911,-3.05285743066206,17.6299049845625));
#78092=CARTESIAN_POINT('Ctrl Pts',(6.10246935669569,-3.45776205930725,17.6090865492287));
#78093=CARTESIAN_POINT('Ctrl Pts',(6.00315165776121,-3.62745406270624,17.6002645423005));
#78094=CARTESIAN_POINT('Ctrl Pts',(5.68456426588421,-4.12278248941258,17.5738682960467));
#78095=CARTESIAN_POINT('Ctrl Pts',(5.44496429707679,-4.43440695890372,17.5563448717549));
#78096=CARTESIAN_POINT('Ctrl Pts',(4.96219934494556,-4.963790794616,17.5238205337869));
#78097=CARTESIAN_POINT('Ctrl Pts',(4.7275055404023,-5.18780550218222,17.5089601753391));
#78098=CARTESIAN_POINT('Ctrl Pts',(4.28541895943661,-5.5547783297998,17.4825233881553));
#78099=CARTESIAN_POINT('Ctrl Pts',(4.08423258697901,-5.70433385709519,17.4709919160538));
#78100=CARTESIAN_POINT('Ctrl Pts',(3.72264300981196,-5.94417265756288,17.4512749069998));
#78101=CARTESIAN_POINT('Ctrl Pts',(3.5658926489595,-6.03950914948238,17.4430343854042));
#78102=CARTESIAN_POINT('Ctrl Pts',(3.04382720564884,-6.32961457142564,17.4162542512617));
#78103=CARTESIAN_POINT('Ctrl Pts',(2.66498689040986,-6.49821087624218,17.3977908826496));
#78104=CARTESIAN_POINT('Ctrl Pts',(2.17883809683168,-6.66485590964755,17.3744533230881));
#78105=CARTESIAN_POINT('Ctrl Pts',(2.08349590294417,-6.69527328252417,17.369895785479));
#78106=CARTESIAN_POINT('Ctrl Pts',(1.76114285095497,-6.79056219558045,17.3545416326272));
#78107=CARTESIAN_POINT('Ctrl Pts',(1.53151605379391,-6.84600727960147,17.3436894004361));
#78108=CARTESIAN_POINT('Ctrl Pts',(1.07736912722764,-6.93166756745294,17.3224239485234));
#78109=CARTESIAN_POINT('Ctrl Pts',(0.853305623856332,-6.96280195982973,
17.3120247101515));
#78110=CARTESIAN_POINT('Ctrl Pts',(0.465224142115352,-6.99771002274748,
17.294304996123));
#78111=CARTESIAN_POINT('Ctrl Pts',(0.301855577424184,-7.00665849027971,
17.2869423355451));
#78112=CARTESIAN_POINT('Ctrl Pts',(-0.31487034555525,-7.01882804343387,
17.2592578592243));
#78113=CARTESIAN_POINT('Ctrl Pts',(-0.767857977525109,-6.98380127946097,
17.239071530554));
#78114=CARTESIAN_POINT('Ctrl Pts',(-1.31309911089605,-6.88792156656363,
17.2139122766892));
#78115=CARTESIAN_POINT('Ctrl Pts',(-1.41152849570265,-6.86842630052985,
17.2093391709666));
#78116=CARTESIAN_POINT('Ctrl Pts',(-1.73908280158202,-6.79621110509029,
17.1940072918837));
#78117=CARTESIAN_POINT('Ctrl Pts',(-1.96596790703423,-6.73408217683143,
17.1831951785447));
#78118=CARTESIAN_POINT('Ctrl Pts',(-2.387998090881,-6.59536487749762,17.1627549784192));
#78119=CARTESIAN_POINT('Ctrl Pts',(-2.58367594814301,-6.52119568161628,
17.1531392145756));
#78120=CARTESIAN_POINT('Ctrl Pts',(-2.91723454841433,-6.37739044629956,
17.1366116831451));
#78121=CARTESIAN_POINT('Ctrl Pts',(-3.05667272893022,-6.31174451470895,
17.1296685981729));
#78122=CARTESIAN_POINT('Ctrl Pts',(-3.60576021747791,-6.03077357350732,
17.1019685257737));
#78123=CARTESIAN_POINT('Ctrl Pts',(-3.99580179444336,-5.77973197456279,
17.081381589345));
#78124=CARTESIAN_POINT('Ctrl Pts',(-4.4367312836426,-5.42983216305697,17.0558080495292));
#78125=CARTESIAN_POINT('Ctrl Pts',(-4.5138578123915,-5.36588755094415,17.0512433669858));
#78126=CARTESIAN_POINT('Ctrl Pts',(-4.76446179643785,-5.14888736696189,
17.0360949011651));
#78127=CARTESIAN_POINT('Ctrl Pts',(-4.93173378149902,-4.9889014263526,17.0254592928678));
#78128=CARTESIAN_POINT('Ctrl Pts',(-5.24325703051603,-4.65994099330217,
17.0046125870816));
#78129=CARTESIAN_POINT('Ctrl Pts',(-5.38800240598723,-4.49179545947177,
16.9944144973066));
#78130=CARTESIAN_POINT('Ctrl Pts',(-5.6235730215545,-4.19033686984055,16.977013590253));
#78131=CARTESIAN_POINT('Ctrl Pts',(-5.71821836225299,-4.06023105500928,
16.9697713622525));
#78132=CARTESIAN_POINT('Ctrl Pts',(-5.98889905027684,-3.65987374037618,
16.9480780493933));
#78133=CARTESIAN_POINT('Ctrl Pts',(-6.15084999122691,-3.38062591369407,
16.9337020803631));
#78134=CARTESIAN_POINT('Ctrl Pts',(-6.38719282423073,-2.89948773449133,
16.9095315441764));
#78135=CARTESIAN_POINT('Ctrl Pts',(-6.47256455400576,-2.70354712639233,
16.8998455551178));
#78136=CARTESIAN_POINT('Ctrl Pts',(-6.6779079742761,-2.16650438430513,16.8735948063815));
#78137=CARTESIAN_POINT('Ctrl Pts',(-6.78067367814398,-1.81952062373872,
16.8569220515564));
#78138=CARTESIAN_POINT('Ctrl Pts',(-6.88455722143499,-1.33373202292574,
16.8341322263777));
#78139=CARTESIAN_POINT('Ctrl Pts',(-6.90903608853085,-1.20049609308365,
16.8279420002742));
#78140=CARTESIAN_POINT('Ctrl Pts',(-6.98395896766335,-0.71374121309055,
16.8056121326512));
#78141=CARTESIAN_POINT('Ctrl Pts',(-7.01124216365981,-0.35721143636207,
16.7897364775856));
#78142=CARTESIAN_POINT('Ctrl Pts',(-7.01124999831217,-0.000153842705974752,
16.7737082138839));
#78143=CARTESIAN_POINT('Origin',(0.,0.,24.4167025567876));
#78144=CARTESIAN_POINT('',(-8.12490033498142,-0.000187321799185458,17.4167025567876));
#78145=CARTESIAN_POINT('Ctrl Pts',(4.94687992157187,6.44602802604219,18.7083406766545));
#78146=CARTESIAN_POINT('Ctrl Pts',(5.82016762916966,5.77439204688032,18.6651775777328));
#78147=CARTESIAN_POINT('Ctrl Pts',(7.46076195865801,3.88189356139278,18.5690832782987));
#78148=CARTESIAN_POINT('Ctrl Pts',(8.46957003418644,0.089278768870349,18.420057778352));
#78149=CARTESIAN_POINT('Ctrl Pts',(7.480065253005,-3.97368988069115,18.2612641768145));
#78150=CARTESIAN_POINT('Ctrl Pts',(4.66731299336978,-7.0680815798286,18.1024705752769));
#78151=CARTESIAN_POINT('Ctrl Pts',(0.716914735007744,-8.43964576898856,
17.9436769737395));
#78152=CARTESIAN_POINT('Ctrl Pts',(-3.40822973045652,-7.75406717637959,
17.7848833722019));
#78153=CARTESIAN_POINT('Ctrl Pts',(-6.70262660827141,-5.17845383384662,
17.6260897706644));
#78154=CARTESIAN_POINT('Ctrl Pts',(-7.98609311183373,-2.21229264724039,
17.503362832193));
#78155=CARTESIAN_POINT('Ctrl Pts',(-8.12526575298013,-0.430719974176783,
17.433567094234));
#78156=CARTESIAN_POINT('Ctrl Pts',(-8.12490033498142,-0.000187321799185458,
17.4167025567876));
#78157=CARTESIAN_POINT('Ctrl Pts',(-8.12490033498142,-0.000187321799185458,
17.4167025567876));
#78158=CARTESIAN_POINT('Ctrl Pts',(-8.12411884851139,0.920553977010579,
17.3806358937215));
#78159=CARTESIAN_POINT('Ctrl Pts',(-7.73854515129239,3.1932071511791,17.2916380301429));
#78160=CARTESIAN_POINT('Ctrl Pts',(-5.66109559838795,6.30028445507239,17.1497089660519));
#78161=CARTESIAN_POINT('Ctrl Pts',(-1.95691771365938,8.24087742028646,16.9909153645144));
#78162=CARTESIAN_POINT('Ctrl Pts',(1.91681060280639,8.17778432394259,16.8437979275536));
#78163=CARTESIAN_POINT('Ctrl Pts',(4.11071045687717,7.08613171679798,16.7496116911053));
#78164=CARTESIAN_POINT('Ctrl Pts',(4.94678612080823,6.44590587665303,16.7083566551695));
#78165=CARTESIAN_POINT('',(-8.12524999730276,-0.00020935965107711,17.5832974432124));
#78166=CARTESIAN_POINT('Ctrl Pts',(-8.12524999730276,-0.00020935965107711,
17.5832974432124));
#78167=CARTESIAN_POINT('Ctrl Pts',(-8.12525538426066,0.208858526346167,
17.5751067683804));
#78168=CARTESIAN_POINT('Ctrl Pts',(-8.11718725248735,0.417953074078032,
17.5669160935484));
#78169=CARTESIAN_POINT('Ctrl Pts',(-8.10106550486504,0.626438543183453,
17.5587254187164));
#78170=CARTESIAN_POINT('Ctrl Pts',(-8.08475759734551,0.837331420865582,
17.5504401651067));
#78171=CARTESIAN_POINT('Ctrl Pts',(-8.06020892462738,1.04760075430505,17.5421549114969));
#78172=CARTESIAN_POINT('Ctrl Pts',(-8.0274942255562,1.25659222549,17.5338696578872));
#78173=CARTESIAN_POINT('Ctrl Pts',(-7.99515416061828,1.46319041961937,17.5256792833041));
#78174=CARTESIAN_POINT('Ctrl Pts',(-7.95483417279298,1.66853956545462,17.5174889087211));
#78175=CARTESIAN_POINT('Ctrl Pts',(-7.90665826764153,1.87201565197404,17.509298534138));
#78176=CARTESIAN_POINT('Ctrl Pts',(-7.8576452427206,2.07902740334725,17.5009658410149));
#78177=CARTESIAN_POINT('Ctrl Pts',(-7.80050083925289,2.28410008993034,17.4926331478919));
#78178=CARTESIAN_POINT('Ctrl Pts',(-7.73540939159931,2.48658985497351,17.4843004547688));
#78179=CARTESIAN_POINT('Ctrl Pts',(-7.67031794394573,2.68907962001667,17.4759677616458));
#78180=CARTESIAN_POINT('Ctrl Pts',(-7.5972795603539,2.88898615586395,17.4676350685228));
#78181=CARTESIAN_POINT('Ctrl Pts',(-7.51653138681063,3.08568363148113,17.4593023753997));
#78182=CARTESIAN_POINT('Ctrl Pts',(-7.43685433004201,3.27977193395646,17.4510802146515));
#78183=CARTESIAN_POINT('Ctrl Pts',(-7.34964262325963,3.47080453946901,17.4428580539032));
#78184=CARTESIAN_POINT('Ctrl Pts',(-7.25515605850115,3.65819602116865,17.434635893155));
#78185=CARTESIAN_POINT('Ctrl Pts',(-7.16068691028673,3.84555296132253,17.4264152479833));
#78186=CARTESIAN_POINT('Ctrl Pts',(-7.05894571328507,4.02926985380545,17.4181946028116));
#78187=CARTESIAN_POINT('Ctrl Pts',(-6.95023901936932,4.20878428244264,17.4099739576399));
#78188=CARTESIAN_POINT('Ctrl Pts',(-6.84154453784167,4.38827854396967,17.4017542359966));
#78189=CARTESIAN_POINT('Ctrl Pts',(-6.72588627446995,4.56357103183399,17.3935345143532));
#78190=CARTESIAN_POINT('Ctrl Pts',(-6.60361549295675,4.73412610559558,17.3853147927099));
#78191=CARTESIAN_POINT('Ctrl Pts',(-6.48133491430855,4.90469484534557,17.3770944124486));
#78192=CARTESIAN_POINT('Ctrl Pts',(-6.3524409285994,5.07052517105891,17.3688740321874));
#78193=CARTESIAN_POINT('Ctrl Pts',(-6.21732730281701,5.23111161916338,17.3606536519262));
#78194=CARTESIAN_POINT('Ctrl Pts',(-6.08221417704902,5.39169747298629,17.352433302086));
#78195=CARTESIAN_POINT('Ctrl Pts',(-5.94088164930919,5.54703926389823,17.3442129522459));
#78196=CARTESIAN_POINT('Ctrl Pts',(-5.79376317510849,5.69666532571967,17.3359926024058));
#78197=CARTESIAN_POINT('Ctrl Pts',(-5.64661324509857,5.84632337950459,17.3277704949499));
#78198=CARTESIAN_POINT('Ctrl Pts',(-5.49367510409307,5.99026305219196,17.319548387494));
#78199=CARTESIAN_POINT('Ctrl Pts',(-5.33541918058525,6.12804942293574,17.3113262800381));
#78200=CARTESIAN_POINT('Ctrl Pts',(-5.26601546468522,6.1884761413677,17.3077204446461));
#78201=CARTESIAN_POINT('Ctrl Pts',(-5.19558943929163,6.24771989754552,17.3041146092542));
#78202=CARTESIAN_POINT('Ctrl Pts',(-5.12418284498617,6.30574640575162,17.3005087738622));
#78203=CARTESIAN_POINT('Ctrl Pts',(-4.96135887548661,6.43806060578053,17.292286614024));
#78204=CARTESIAN_POINT('Ctrl Pts',(-4.79338046715548,6.56408672460702,17.2840644541859));
#78205=CARTESIAN_POINT('Ctrl Pts',(-4.6207558352372,6.68343497564099,17.2758422943477));
#78206=CARTESIAN_POINT('Ctrl Pts',(-4.44816302311957,6.80276122727944,17.2676216500956));
#78207=CARTESIAN_POINT('Ctrl Pts',(-4.27092593939041,6.91541190012624,17.2594010058435));
#78208=CARTESIAN_POINT('Ctrl Pts',(-4.08958285136217,7.02103978512759,17.2511803615913));
#78209=CARTESIAN_POINT('Ctrl Pts',(-3.90826013602747,7.12665580353643,17.2429606408741));
#78210=CARTESIAN_POINT('Ctrl Pts',(-3.7228325922447,7.2252504607178,17.2347409201569));
#78211=CARTESIAN_POINT('Ctrl Pts',(-3.53386493967195,7.31652145152718,17.2265211994396));
#78212=CARTESIAN_POINT('Ctrl Pts',(-3.34488214583468,7.40779975553644,17.2183008201072));
#78213=CARTESIAN_POINT('Ctrl Pts',(-3.15235894102377,7.49175308982551,17.2100804407748));
#78214=CARTESIAN_POINT('Ctrl Pts',(-2.95688293066066,7.56812598315248,17.2018600614424));
#78215=CARTESIAN_POINT('Ctrl Pts',(-2.761407643692,7.64449859384769,17.193639712531));
#78216=CARTESIAN_POINT('Ctrl Pts',(-2.56297984890816,7.7132907147765,17.1854193636196));
#78217=CARTESIAN_POINT('Ctrl Pts',(-2.36220583361238,7.7742955412145,17.1771990147081));
#78218=CARTESIAN_POINT('Ctrl Pts',(-2.16138889010998,7.83531341131151,17.1689769081747));
#78219=CARTESIAN_POINT('Ctrl Pts',(-1.95822500634198,7.88854057469016,17.1607548016412));
#78220=CARTESIAN_POINT('Ctrl Pts',(-1.75333535652475,7.93382018261444,17.1525326951077));
#78221=CARTESIAN_POINT('Ctrl Pts',(-1.66348010082346,7.95367775351526,17.1489268541801));
#78222=CARTESIAN_POINT('Ctrl Pts',(-1.57329309072578,7.97200742702453,17.1453210132524));
#78223=CARTESIAN_POINT('Ctrl Pts',(-1.48282738326448,7.9887990658134,17.1417151723247));
#78224=CARTESIAN_POINT('Ctrl Pts',(-1.27654442924292,8.02708792630468,17.1334930123575));
#78225=CARTESIAN_POINT('Ctrl Pts',(-1.06874362769325,8.05738902441135,17.1252708523903));
#78226=CARTESIAN_POINT('Ctrl Pts',(-0.860057740986279,8.07960322322016,
17.1170486924231));
#78227=CARTESIAN_POINT('Ctrl Pts',(-0.651410321219439,8.10181332729947,
17.1088280480416));
#78228=CARTESIAN_POINT('Ctrl Pts',(-0.441878435251749,8.11593947599364,
17.10060740366));
#78229=CARTESIAN_POINT('Ctrl Pts',(-0.232100864634496,8.12193429862221,
17.0923867592785));
#78230=CARTESIAN_POINT('Ctrl Pts',(-0.0223468611301164,8.1279284477724,
17.0841670384316));
#78231=CARTESIAN_POINT('Ctrl Pts',(0.18765247701369,8.12579308616848,17.0759473175847));
#78232=CARTESIAN_POINT('Ctrl Pts',(0.39725662308003,8.11553293000029,17.0677275967378));
#78233=CARTESIAN_POINT('Ctrl Pts',(0.606877563909257,8.10527195172579,17.0595072172767));
#78234=CARTESIAN_POINT('Ctrl Pts',(0.816102954456935,8.08688488981133,17.0512868378156));
#78235=CARTESIAN_POINT('Ctrl Pts',(1.02429457811477,8.06042853573832,17.0430664583545));
#78236=CARTESIAN_POINT('Ctrl Pts',(1.2324854313022,8.03397227957434,17.0348461093152));
#78237=CARTESIAN_POINT('Ctrl Pts',(1.43964223279993,7.99944683084303,17.0266257602759));
#78238=CARTESIAN_POINT('Ctrl Pts',(1.64513364442268,7.95696065432578,17.0184054112366));
#78239=CARTESIAN_POINT('Ctrl Pts',(1.850668992846,7.91446539369815,17.0101833045772));
#78240=CARTESIAN_POINT('Ctrl Pts',(2.05453795092107,7.86400606457075,17.0019611979178));
#78241=CARTESIAN_POINT('Ctrl Pts',(2.25612000826752,7.80574212172007,16.9937390912584));
#78242=CARTESIAN_POINT('Ctrl Pts',(2.34452468451809,7.78019021956866,16.9901332511013));
#78243=CARTESIAN_POINT('Ctrl Pts',(2.43248969275652,7.75313791034859,16.9865274109443));
#78244=CARTESIAN_POINT('Ctrl Pts',(2.51996359225185,7.72460167621769,16.9829215707872));
#78245=CARTESIAN_POINT('Ctrl Pts',(2.71942272518129,7.65953298087359,16.9746994867672));
#78246=CARTESIAN_POINT('Ctrl Pts',(2.91639318855617,7.58672398261398,16.9664774027471));
#78247=CARTESIAN_POINT('Ctrl Pts',(3.11027192380636,7.50639035239188,16.9582553187271));
#78248=CARTESIAN_POINT('Ctrl Pts',(3.30412189462654,7.42606864070784,16.9500344545601));
#78249=CARTESIAN_POINT('Ctrl Pts',(3.49488077973406,7.33822463680505,16.9418135903931));
#78250=CARTESIAN_POINT('Ctrl Pts',(3.68196493807873,7.24312237624485,16.9335927262261));
#78251=CARTESIAN_POINT('Ctrl Pts',(3.86902427864327,7.14803273154168,16.9253729526036));
#78252=CARTESIAN_POINT('Ctrl Pts',(4.05240960296455,7.04568688678982,16.9171531789811));
#78253=CARTESIAN_POINT('Ctrl Pts',(4.23156069383441,6.93639543688908,16.9089334053586));
#78254=CARTESIAN_POINT('Ctrl Pts',(4.41071458111957,6.82710228103009,16.9007135034315));
#78255=CARTESIAN_POINT('Ctrl Pts',(4.58563385038789,6.71086345612257,16.8924936015045));
#78256=CARTESIAN_POINT('Ctrl Pts',(4.75578533036544,6.58803411147672,16.8842736995774));
#78257=CARTESIAN_POINT('Ctrl Pts',(4.82013425799734,6.54158175848671,16.8811650467798));
#78258=CARTESIAN_POINT('Ctrl Pts',(4.88380156985135,6.49418724095744,16.8780563939822));
#78259=CARTESIAN_POINT('Ctrl Pts',(4.94675954817621,6.44587135576157,16.8749477411846));
#78260=CARTESIAN_POINT('Ctrl Pts',(4.94710325578446,6.44631862759455,18.8749389137103));
#78261=CARTESIAN_POINT('Ctrl Pts',(5.92706477576575,5.69317017844722,18.8265096717068));
#78262=CARTESIAN_POINT('Ctrl Pts',(7.61516726084699,3.64267874792156,18.7251492291908));
#78263=CARTESIAN_POINT('Ctrl Pts',(8.46357381179856,-0.330935089626715,
18.5708575861624));
#78264=CARTESIAN_POINT('Ctrl Pts',(7.27375726455099,-4.33981891403078,18.4120639846248));
#78265=CARTESIAN_POINT('Ctrl Pts',(4.31098181048916,-7.29088689580246,18.2532703830874));
#78266=CARTESIAN_POINT('Ctrl Pts',(0.297414436183603,-8.46481700753604,
18.0944767815498));
#78267=CARTESIAN_POINT('Ctrl Pts',(-3.78864659254454,-7.57546998599963,
17.9356831800123));
#78268=CARTESIAN_POINT('Ctrl Pts',(-6.95123456136923,-4.83962029144108,
17.7768895784748));
#78269=CARTESIAN_POINT('Ctrl Pts',(-8.03731400816114,-1.94327236285129,
17.6594276662081));
#78270=CARTESIAN_POINT('Ctrl Pts',(-8.12560543629606,-0.296289995508007,
17.594896954454));
#78271=CARTESIAN_POINT('Ctrl Pts',(-8.12529972492543,-0.000209360932384682,
17.5832974432124));
#78272=CARTESIAN_POINT('Origin',(-15.,0.,10.));
#78273=CARTESIAN_POINT('',(-18.5,4.28626379701574E-16,20.));
#78274=CARTESIAN_POINT('Origin',(-15.,0.,20.));
#78275=CARTESIAN_POINT('',(-18.5,4.28626379701574E-16,0.));
#78276=CARTESIAN_POINT('',(-18.5,4.28626379701574E-16,10.));
#78277=CARTESIAN_POINT('Origin',(-15.,0.,0.));
#78278=CARTESIAN_POINT('Origin',(15.,0.,10.));
#78279=CARTESIAN_POINT('',(11.5,4.28626379701574E-16,20.));
#78280=CARTESIAN_POINT('Origin',(15.,0.,20.));
#78281=CARTESIAN_POINT('',(11.5,4.28626379701574E-16,0.));
#78282=CARTESIAN_POINT('',(11.5,4.28626379701574E-16,10.));
#78283=CARTESIAN_POINT('Origin',(15.,0.,0.));
#78284=CARTESIAN_POINT('Ctrl Pts',(5.309423840314,4.57791301092332,19.9996006767769));
#78285=CARTESIAN_POINT('Ctrl Pts',(6.07080882312251,3.6948682496547,19.9466604262186));
#78286=CARTESIAN_POINT('Ctrl Pts',(7.14359879543109,1.54261656134898,19.8407889751478));
#78287=CARTESIAN_POINT('Ctrl Pts',(7.01054163748306,-2.06378246543655,19.6819863235645));
#78288=CARTESIAN_POINT('Ctrl Pts',(5.16894015188214,-5.16605670552577,19.523192722027));
#78289=CARTESIAN_POINT('Ctrl Pts',(2.06730382912507,-7.00954776020371,19.3643991204894));
#78290=CARTESIAN_POINT('Ctrl Pts',(-1.53817327458349,-7.1442614489232,19.2056055189519));
#78291=CARTESIAN_POINT('Ctrl Pts',(-4.7687545802584,-5.53768944867667,19.0468119174144));
#78292=CARTESIAN_POINT('Ctrl Pts',(-6.83694841393584,-2.58126320243491,
18.8880183158769));
#78293=CARTESIAN_POINT('Ctrl Pts',(-7.23866073718961,1.00431105009051,18.7292247143393));
#78294=CARTESIAN_POINT('Ctrl Pts',(-5.87596341879415,4.34510146585654,18.5704311128019));
#78295=CARTESIAN_POINT('Ctrl Pts',(-3.08101653625123,6.62677675416298,18.4116375112643));
#78296=CARTESIAN_POINT('Ctrl Pts',(0.464921543395092,7.2931953172938,18.2528439097268));
#78297=CARTESIAN_POINT('Ctrl Pts',(3.89753562459927,6.18191362226655,18.0940503081893));
#78298=CARTESIAN_POINT('Ctrl Pts',(6.38013528416437,3.56380671277158,17.9352567066518));
#78299=CARTESIAN_POINT('Ctrl Pts',(7.30759258545994,0.077030223116708,17.7764631051143));
#78300=CARTESIAN_POINT('Ctrl Pts',(6.45384230379842,-3.42852194289047,17.6176695035767));
#78301=CARTESIAN_POINT('Ctrl Pts',(4.02698385947594,-6.09838047713161,17.4588759020392));
#78302=CARTESIAN_POINT('Ctrl Pts',(0.618558059122632,-7.2817737614107,17.3000823005017));
#78303=CARTESIAN_POINT('Ctrl Pts',(-2.9406397499871,-6.69025270191448,17.1412886989642));
#78304=CARTESIAN_POINT('Ctrl Pts',(-5.78306387549879,-4.46799904689602,
16.9824950974267));
#78305=CARTESIAN_POINT('Ctrl Pts',(-7.21588046124865,-1.15668166355883,
16.8237014958892));
#78306=CARTESIAN_POINT('Ctrl Pts',(-6.88984399838259,2.4365740239086,16.6649078943516));
#78307=CARTESIAN_POINT('Ctrl Pts',(-4.88442507156545,5.43592080640939,16.5061142928141));
#78308=CARTESIAN_POINT('Ctrl Pts',(-1.68843959220725,7.11027531398814,16.3473206912766));
#78309=CARTESIAN_POINT('Ctrl Pts',(1.91909886907681,7.05151776748327,16.1885270897391));
#78310=CARTESIAN_POINT('Ctrl Pts',(5.05886171908715,5.27397017464772,16.0297334882016));
#78311=CARTESIAN_POINT('Ctrl Pts',(6.96553951464736,2.21090537228499,15.8709398866641));
#78312=CARTESIAN_POINT('Ctrl Pts',(7.17438425046917,-1.39106215608347,15.7121462851265));
#78313=CARTESIAN_POINT('Ctrl Pts',(5.63449053777354,-4.65396171828115,15.553352683589));
#78314=CARTESIAN_POINT('Ctrl Pts',(2.72120366726484,-6.78246960160486,15.3945590820515));
#78315=CARTESIAN_POINT('Ctrl Pts',(-0.855369878873554,-7.25776726450987,
15.235765480514));
#78316=CARTESIAN_POINT('Ctrl Pts',(-4.22344912882297,-5.9640020750913,15.0769718789765));
#78317=CARTESIAN_POINT('Ctrl Pts',(-6.56207308072387,-3.21652610415333,
14.9181782774389));
#78318=CARTESIAN_POINT('Ctrl Pts',(-7.30120792003263,0.314970163523136,
14.7593846759014));
#78319=CARTESIAN_POINT('Ctrl Pts',(-6.26069135448818,3.76969323145719,14.6005910743639));
#78320=CARTESIAN_POINT('Ctrl Pts',(-3.69414672805278,6.30556288106581,14.4417974728264));
#78321=CARTESIAN_POINT('Ctrl Pts',(-0.227162956982798,7.30446714596158,
14.2830038712889));
#78322=CARTESIAN_POINT('Ctrl Pts',(3.2951912240184,6.52292557773042,14.1242102697514));
#78323=CARTESIAN_POINT('Ctrl Pts',(6.01435067952836,4.15143700411245,13.9654166682138));
#78324=CARTESIAN_POINT('Ctrl Pts',(7.26752700548849,0.768045910055647,13.8066230666763));
#78325=CARTESIAN_POINT('Ctrl Pts',(6.74926156636189,-2.80255447837998,13.6478294651388));
#78326=CARTESIAN_POINT('Ctrl Pts',(4.58588028341133,-5.69003913182298,13.4890358636013));
#78327=CARTESIAN_POINT('Ctrl Pts',(1.30470200327209,-7.19059079478976,13.3302422620638));
#78328=CARTESIAN_POINT('Ctrl Pts',(-2.29449416903913,-6.938453704083,13.1714486605263));
#78329=CARTESIAN_POINT('Ctrl Pts',(-5.33441305243017,-4.99508565307144,
13.0126550589887));
#78330=CARTESIAN_POINT('Ctrl Pts',(-7.07408192420626,-1.83417780628703,
12.8538614574512));
#78331=CARTESIAN_POINT('Ctrl Pts',(-7.0894607918695,1.77380635245304,12.6950678559137));
#78332=CARTESIAN_POINT('Ctrl Pts',(-5.37680109439524,4.94942959206086,12.5362742543762));
#78333=CARTESIAN_POINT('Ctrl Pts',(-2.35355940472716,6.91864158804875,12.3774806528387));
#78334=CARTESIAN_POINT('Ctrl Pts',(1.24335657923632,7.20145177810193,12.2186870513011));
#78335=CARTESIAN_POINT('Ctrl Pts',(4.53720746668328,5.72892587661342,12.0598934497636));
#78336=CARTESIAN_POINT('Ctrl Pts',(6.72512523585276,2.85998843661194,11.9010998482261));
#78337=CARTESIAN_POINT('Ctrl Pts',(7.2738103321706,-0.706064123904859,11.7423062466886));
#78338=CARTESIAN_POINT('Ctrl Pts',(6.04952211803567,-4.10001529739278,11.5835126451511));
#78339=CARTESIAN_POINT('Ctrl Pts',(3.35067782304803,-6.49459786450181,11.4247190436135));
#78340=CARTESIAN_POINT('Ctrl Pts',(-0.164885918955666,-7.30613823638642,
11.2659254420761));
#78341=CARTESIAN_POINT('Ctrl Pts',(-3.64025912529407,-6.33682545097865,
11.1071318405385));
#78342=CARTESIAN_POINT('Ctrl Pts',(-6.22832815712936,-3.82292710662485,
10.948338239001));
#78343=CARTESIAN_POINT('Ctrl Pts',(-7.29825757752986,-0.377199718300082,
10.7895446374635));
#78344=CARTESIAN_POINT('Ctrl Pts',(-6.589254731778,3.16046917010732,10.630751035926));
#78345=CARTESIAN_POINT('Ctrl Pts',(-4.27413731309761,5.92778150105453,10.4719574343885));
#78346=CARTESIAN_POINT('Ctrl Pts',(-0.917209476593015,7.25021172597777,
10.313163832851));
#78347=CARTESIAN_POINT('Ctrl Pts',(2.66328590537004,6.80542074244604,10.1543702313134));
#78348=CARTESIAN_POINT('Ctrl Pts',(5.59461192317713,4.70182525456889,9.99557662977594));
#78349=CARTESIAN_POINT('Ctrl Pts',(7.16226509701906,1.45217146903525,9.8367830282384));
#78350=CARTESIAN_POINT('Ctrl Pts',(6.98413383608689,-2.15144552686879,9.67798942670091));
#78351=CARTESIAN_POINT('Ctrl Pts',(5.10363719545182,-5.2306529872147,9.51919582516338));
#78352=CARTESIAN_POINT('Ctrl Pts',(1.97914158858717,-7.03490169567296,9.36040222362587));
#78353=CARTESIAN_POINT('Ctrl Pts',(-1.62776489427362,-7.12441048399288,
9.20160862208835));
#78354=CARTESIAN_POINT('Ctrl Pts',(-4.83790770287762,-5.47736180600617,
9.04281502055083));
#78355=CARTESIAN_POINT('Ctrl Pts',(-6.86882245301825,-2.49521971064066,
8.88402141901332));
#78356=CARTESIAN_POINT('Ctrl Pts',(-7.22547868839144,1.09512602884728,8.7252278174758));
#78357=CARTESIAN_POINT('Ctrl Pts',(-5.82094233215892,4.41853750251569,8.56643421593827));
#78358=CARTESIAN_POINT('Ctrl Pts',(-2.99756565354991,6.66494136869301,8.40764061440078));
#78359=CARTESIAN_POINT('Ctrl Pts',(0.556460252544306,7.28678223105342,8.24884701286324));
#78360=CARTESIAN_POINT('Ctrl Pts',(3.97485034590289,6.13248791463411,8.09005341132574));
#78361=CARTESIAN_POINT('Ctrl Pts',(6.42438048079358,3.48341480927208,7.93125980978821));
#78362=CARTESIAN_POINT('Ctrl Pts',(7.30798373438186,-0.0147320557892091,
7.7724662082507));
#78363=CARTESIAN_POINT('Ctrl Pts',(6.41028399509764,-3.50928801862323,7.61367260671317));
#78364=CARTESIAN_POINT('Ctrl Pts',(3.95009335809719,-6.14846369085595,7.45487900517566));
#78365=CARTESIAN_POINT('Ctrl Pts',(0.527077217284989,-7.28896651813388,
7.29608540363814));
#78366=CARTESIAN_POINT('Ctrl Pts',(-3.02441269396098,-6.65280175204892,
7.13729180210062));
#78367=CARTESIAN_POINT('Ctrl Pts',(-5.83870947790314,-4.39503298373306,
6.9784982005631));
#78368=CARTESIAN_POINT('Ctrl Pts',(-7.22983524155821,-1.06598577635001,
6.81970459902561));
#78369=CARTESIAN_POINT('Ctrl Pts',(-6.85870651452891,2.52289283224952,6.66091099748806));
#78370=CARTESIAN_POINT('Ctrl Pts',(-4.81578500776411,5.49682254165551,6.50211739595056));
#78371=CARTESIAN_POINT('Ctrl Pts',(-1.59902779485203,7.13091532741401,6.34332379441303));
#78372=CARTESIAN_POINT('Ctrl Pts',(2.00748849528066,7.02686510734148,6.18453019287553));
#78373=CARTESIAN_POINT('Ctrl Pts',(5.12468442089522,5.21003386569524,6.02573659133799));
#78374=CARTESIAN_POINT('Ctrl Pts',(6.99275117104099,2.12326973212599,5.8669429898005));
#78375=CARTESIAN_POINT('Ctrl Pts',(7.1563520873638,-1.48103615659492,5.70814938826297));
#78376=CARTESIAN_POINT('Ctrl Pts',(5.57560985041754,-4.72434313861562,5.54935578672546));
#78377=CARTESIAN_POINT('Ctrl Pts',(2.63582647782784,-6.81610314433688,5.39056218518792));
#78378=CARTESIAN_POINT('Ctrl Pts',(-0.94643309124788,-7.2464548366252,5.23176858365042));
#78379=CARTESIAN_POINT('Ctrl Pts',(-4.29800193094195,-5.91050105296297,
5.07297498211289));
#78380=CARTESIAN_POINT('Ctrl Pts',(-6.60194341113072,-3.13387722983619,
4.91418138057538));
#78381=CARTESIAN_POINT('Ctrl Pts',(-7.29667748412521,0.406621430961608,
4.75538777903787));
#78382=CARTESIAN_POINT('Ctrl Pts',(-6.21286443483388,3.84800712185327,4.59659417750035));
#78383=CARTESIAN_POINT('Ctrl Pts',(-3.61468101823925,6.35145057698171,4.43780057596283));
#78384=CARTESIAN_POINT('Ctrl Pts',(-0.135428027587841,7.30674363480701,
4.27900697442531));
#78385=CARTESIAN_POINT('Ctrl Pts',(3.37683521043622,6.48103597097203,4.1202133728878));
#78386=CARTESIAN_POINT('Ctrl Pts',(6.06600320284556,4.0755917899732,3.96141977135028));
#78387=CARTESIAN_POINT('Ctrl Pts',(7.27659789067257,0.676732172240444,3.80262616981276));
#78388=CARTESIAN_POINT('Ctrl Pts',(6.71353980753754,-2.88707924173838,3.64383256827526));
#78389=CARTESIAN_POINT('Ctrl Pts',(4.51407297111273,-5.74717221829848,3.48503896673773));
#78390=CARTESIAN_POINT('Ctrl Pts',(1.21431199256477,-7.2064061556807,3.32624536520021));
#78391=CARTESIAN_POINT('Ctrl Pts',(-2.38143453615604,-6.9090963840742,3.16745176366269));
#78392=CARTESIAN_POINT('Ctrl Pts',(-5.39671227621279,-4.92771142671896,
3.00865816212518));
#78393=CARTESIAN_POINT('Ctrl Pts',(-7.09655472247411,-1.74520897437011,
2.84986456058766));
#78394=CARTESIAN_POINT('Ctrl Pts',(-7.06662947590349,1.86268385571119,2.69107095905014));
#78395=CARTESIAN_POINT('Ctrl Pts',(-5.31423074035417,5.01655209682087,2.53227735751262));
#78396=CARTESIAN_POINT('Ctrl Pts',(-2.26650138338798,6.94764814525486,2.37348375597511));
#78397=CARTESIAN_POINT('Ctrl Pts',(1.3336820929718,7.18527211938174,2.21469015443759));
#78398=CARTESIAN_POINT('Ctrl Pts',(4.6087838462063,5.67150373744236,2.05589655290007));
#78399=CARTESIAN_POINT('Ctrl Pts',(6.76050592645423,2.7753203538901,1.89710295136255));
#78400=CARTESIAN_POINT('Ctrl Pts',(7.26437135605648,-0.797340577473384,
1.73830934982504));
#78401=CARTESIAN_POINT('Ctrl Pts',(5.99756424523123,-4.17565158683848,1.57951574828752));
#78402=CARTESIAN_POINT('Ctrl Pts',(3.26886557238479,-6.5361580764171,1.42072214675001));
#78403=CARTESIAN_POINT('Ctrl Pts',(-0.256610847367315,-7.3034916889936,
1.26192854521248));
#78404=CARTESIAN_POINT('Ctrl Pts',(-3.71953933312641,-6.29061818321811,
1.10313494367497));
#78405=CARTESIAN_POINT('Ctrl Pts',(-6.27583864718436,-3.74442015813873,
0.944341342137453));
#78406=CARTESIAN_POINT('Ctrl Pts',(-7.30241904852373,-0.285532637982764,
0.785547740599942));
#78407=CARTESIAN_POINT('Ctrl Pts',(-6.54905035033283,3.24295998468523,0.626754139062419));
#78408=CARTESIAN_POINT('Ctrl Pts',(-4.19937168621273,5.98097490181152,0.467960537524906));
#78409=CARTESIAN_POINT('Ctrl Pts',(-0.826096925787518,7.26116991578662,
0.309166935987384));
#78410=CARTESIAN_POINT('Ctrl Pts',(2.74851800665292,6.77141768319735,0.15037333444987));
#78411=CARTESIAN_POINT('Ctrl Pts',(5.65322566751968,4.63125733214954,-0.00842026708764997));
#78412=CARTESIAN_POINT('Ctrl Pts',(7.17990031857721,1.36202628232418,-0.167213868625169));
#78413=CARTESIAN_POINT('Ctrl Pts',(6.95663626177777,-2.23877288639238,-0.326007470162682));
#78414=CARTESIAN_POINT('Ctrl Pts',(5.03742250863045,-5.29474283456939,-0.484801071700202));
#78415=CARTESIAN_POINT('Ctrl Pts',(2.9397676306177,-6.47024305947933,-0.590663472725211));
#78416=CARTESIAN_POINT('Ctrl Pts',(1.81369031944497,-6.77183848624123,-0.643594673237717));
#78417=CARTESIAN_POINT('Ctrl Pts',(5.59097265709334,4.82067117646242,20.2142331247627));
#78418=CARTESIAN_POINT('Ctrl Pts',(6.39273246162839,3.8908002029388,20.1612928742045));
#78419=CARTESIAN_POINT('Ctrl Pts',(7.5224104798795,1.62441863265741,20.0554214231337));
#78420=CARTESIAN_POINT('Ctrl Pts',(7.38229754968369,-2.17322098997506,19.8966187715504));
#78421=CARTESIAN_POINT('Ctrl Pts',(5.44303938139093,-5.44000303126678,19.7378251700128));
#78422=CARTESIAN_POINT('Ctrl Pts',(2.17692908499447,-7.38125096895092,19.5790315684753));
#78423=CARTESIAN_POINT('Ctrl Pts',(-1.6197397267044,-7.52310827264703,19.4202379669378));
#78424=CARTESIAN_POINT('Ctrl Pts',(-5.02163271731505,-5.83134276377425,
19.2614443654003));
#78425=CARTESIAN_POINT('Ctrl Pts',(-7.19949900213887,-2.71814276268464,
19.1026507638628));
#78426=CARTESIAN_POINT('Ctrl Pts',(-7.62251337862843,1.05756778685438,18.9438571623252));
#78427=CARTESIAN_POINT('Ctrl Pts',(-6.18755476990059,4.5755140705556,18.7850635607877));
#78428=CARTESIAN_POINT('Ctrl Pts',(-3.2443970811745,6.9781823323029,18.6262699592502));
#78429=CARTESIAN_POINT('Ctrl Pts',(0.489575463363619,7.67993982552714,18.4674763577127));
#78430=CARTESIAN_POINT('Ctrl Pts',(4.10421464975624,6.50972894048726,18.3086827561752));
#78431=CARTESIAN_POINT('Ctrl Pts',(6.71846192640929,3.75278871786083,18.1498891546376));
#78432=CARTESIAN_POINT('Ctrl Pts',(7.69510055389895,0.0811149917897368,
17.9910955531002));
#78433=CARTESIAN_POINT('Ctrl Pts',(6.7960774914506,-3.61033004963708,17.8323019515626));
#78434=CARTESIAN_POINT('Ctrl Pts',(4.24052728243949,-6.42176618888618,17.6735083500251));
#78435=CARTESIAN_POINT('Ctrl Pts',(0.651359036195312,-7.66791260589571,
17.5147147484876));
#78436=CARTESIAN_POINT('Ctrl Pts',(-3.09657637646184,-7.04502429085348,
17.3559211469501));
#78437=CARTESIAN_POINT('Ctrl Pts',(-6.08972893756129,-4.70492868047947,
17.1971275454125));
#78438=CARTESIAN_POINT('Ctrl Pts',(-7.59852510725709,-1.21801832899748,
17.038333943875));
#78439=CARTESIAN_POINT('Ctrl Pts',(-7.25519954050563,2.56578098761301,16.8795403423375));
#78440=CARTESIAN_POINT('Ctrl Pts',(-5.14343699845378,5.72417752073118,16.7207467408));
#78441=CARTESIAN_POINT('Ctrl Pts',(-1.77797438612968,7.48731991653589,16.5619531392625));
#78442=CARTESIAN_POINT('Ctrl Pts',(2.02086509308187,7.42544656722586,16.403159537725));
#78443=CARTESIAN_POINT('Ctrl Pts',(5.3271236951691,5.55363894984081,16.2443659361875));
#78444=CARTESIAN_POINT('Ctrl Pts',(7.33490904843519,2.3281455494303,16.0855723346499));
#78445=CARTESIAN_POINT('Ctrl Pts',(7.55482843002453,-1.46482758071166,15.9267787331124));
#78446=CARTESIAN_POINT('Ctrl Pts',(5.9332770335924,-4.90075260454817,15.7679851315749));
#78447=CARTESIAN_POINT('Ctrl Pts',(2.86550400865343,-7.14213128027408,15.6091915300374));
#78448=CARTESIAN_POINT('Ctrl Pts',(-0.900728543871616,-7.64263308936021,
15.4503979284999));
#78449=CARTESIAN_POINT('Ctrl Pts',(-4.4474107375985,-6.28026195149481,15.2916043269623));
#78450=CARTESIAN_POINT('Ctrl Pts',(-6.91004754406753,-3.38709246803788,
15.1328107254248));
#78451=CARTESIAN_POINT('Ctrl Pts',(-7.68837732160438,0.331672442250143,
14.9740171238873));
#78452=CARTESIAN_POINT('Ctrl Pts',(-6.59268410852166,3.96959301359157,14.8152235223498));
#78453=CARTESIAN_POINT('Ctrl Pts',(-3.89004042039568,6.63993508823676,14.6564299208123));
#78454=CARTESIAN_POINT('Ctrl Pts',(-0.239208983760499,7.69180937818906,
14.4976363192748));
#78455=CARTESIAN_POINT('Ctrl Pts',(3.46992905209301,6.86882412220246,14.3388427177373));
#78456=CARTESIAN_POINT('Ctrl Pts',(6.33328044826521,4.37157994458877,14.1800491161997));
#78457=CARTESIAN_POINT('Ctrl Pts',(7.65291037115065,0.808773948297097,14.0212555146622));
#78458=CARTESIAN_POINT('Ctrl Pts',(7.10716228502651,-2.95116870114297,13.8624619131247));
#78459=CARTESIAN_POINT('Ctrl Pts',(4.82906093851039,-5.99177126569951,13.7036683115872));
#78460=CARTESIAN_POINT('Ctrl Pts',(1.37388791050401,-7.57189437708162,13.5448747100497));
#78461=CARTESIAN_POINT('Ctrl Pts',(-2.41616690375189,-7.30638692799138,
13.3860811085121));
#78462=CARTESIAN_POINT('Ctrl Pts',(-5.61728700039421,-5.25996570364403,
13.2272875069746));
#78463=CARTESIAN_POINT('Ctrl Pts',(-7.44920725898131,-1.93144082514832,
13.0684939054371));
#78464=CARTESIAN_POINT('Ctrl Pts',(-7.46540163923577,1.86786798602179,12.9097003038996));
#78465=CARTESIAN_POINT('Ctrl Pts',(-5.66192280095226,5.21188858710221,12.7509067023621));
#78466=CARTESIAN_POINT('Ctrl Pts',(-2.47836425842699,7.28552421249568,12.5921131008245));
#78467=CARTESIAN_POINT('Ctrl Pts',(1.30928945335738,7.58333129802704,12.433319499287));
#78468=CARTESIAN_POINT('Ctrl Pts',(4.77780709333722,6.03272010184176,12.2745258977495));
#78469=CARTESIAN_POINT('Ctrl Pts',(7.08174605004928,3.01164827476927,12.115732296212));
#78470=CARTESIAN_POINT('Ctrl Pts',(7.6595268908959,-0.743505383942599,11.9569386946745));
#78471=CARTESIAN_POINT('Ctrl Pts',(6.37031696238033,-4.31743144092858,11.798145093137));
#78472=CARTESIAN_POINT('Ctrl Pts',(3.52835800170037,-6.83899424331869,11.6393514915994));
#78473=CARTESIAN_POINT('Ctrl Pts',(-0.173629510874831,-7.69356908341393,
11.4805578900619));
#78474=CARTESIAN_POINT('Ctrl Pts',(-3.83329525884111,-6.67285545376605,
11.3217642885244));
#78475=CARTESIAN_POINT('Ctrl Pts',(-6.55860475133126,-4.0256497816035,11.1629706869869));
#78476=CARTESIAN_POINT('Ctrl Pts',(-7.68527052795628,-0.397201913937679,
11.0041770854494));
#78477=CARTESIAN_POINT('Ctrl Pts',(-6.93867058724303,3.32806293961483,10.8453834839119));
#78478=CARTESIAN_POINT('Ctrl Pts',(-4.50078682149019,6.24212066815513,10.6865898823743));
#78479=CARTESIAN_POINT('Ctrl Pts',(-0.965847379808193,7.63467689474983,
10.5277962808368));
#78480=CARTESIAN_POINT('Ctrl Pts',(2.80451497616083,7.16629947719176,10.3690026792993));
#78481=CARTESIAN_POINT('Ctrl Pts',(5.89128373064334,4.95115425465278,10.2102090777618));
#78482=CARTESIAN_POINT('Ctrl Pts',(7.54206662053171,1.52917740624509,10.0514154762243));
#78483=CARTESIAN_POINT('Ctrl Pts',(7.35448939196629,-2.2655326596111,9.89262187468675));
#78484=CARTESIAN_POINT('Ctrl Pts',(5.37427353130809,-5.5080247329683,9.73382827314923));
#78485=CARTESIAN_POINT('Ctrl Pts',(2.08409176571836,-7.40794937620217,9.57503467161171));
#78486=CARTESIAN_POINT('Ctrl Pts',(-1.71408222243603,-7.50220464817096,
9.4162410700742));
#78487=CARTESIAN_POINT('Ctrl Pts',(-5.09445290069936,-5.76781605903527,
9.25744746853669));
#78488=CARTESIAN_POINT('Ctrl Pts',(-7.23306326190427,-2.62753654543564,
9.09865386699916));
#78489=CARTESIAN_POINT('Ctrl Pts',(-7.60863231043503,1.15319851409607,8.93986026546165));
#78490=CARTESIAN_POINT('Ctrl Pts',(-6.12961601793934,4.65284428290165,8.78106666392412));
#78491=CARTESIAN_POINT('Ctrl Pts',(-3.15652095423003,7.01837074496753,8.62227306238662));
#78492=CARTESIAN_POINT('Ctrl Pts',(0.585968299066983,7.67318666531695,8.46347946084909));
#78493=CARTESIAN_POINT('Ctrl Pts',(4.18562922613967,6.45768228001306,8.30468585931157));
#78494=CARTESIAN_POINT('Ctrl Pts',(6.76505336307016,3.66813378206446,8.14589225777407));
#78495=CARTESIAN_POINT('Ctrl Pts',(7.69551244471668,-0.0155132691564084,
7.98709865623654));
#78496=CARTESIAN_POINT('Ctrl Pts',(6.75020936710044,-3.69537899932045,7.82830505469903));
#78497=CARTESIAN_POINT('Ctrl Pts',(4.15955942157017,-6.47450522177069,7.6695114531615));
#78498=CARTESIAN_POINT('Ctrl Pts',(0.55502713639884,-7.67548678105631,7.51071785162399));
#78499=CARTESIAN_POINT('Ctrl Pts',(-3.18479164298584,-7.00558738715583,
7.35192425008647));
#78500=CARTESIAN_POINT('Ctrl Pts',(-6.14832532219495,-4.62809336344519,
7.19313064854895));
#78501=CARTESIAN_POINT('Ctrl Pts',(-7.61321988346879,-1.12251300850581,
7.03433704701144));
#78502=CARTESIAN_POINT('Ctrl Pts',(-7.22241089411526,2.65667712093025,6.87554344547392));
#78503=CARTESIAN_POINT('Ctrl Pts',(-5.07115708043697,5.78830876110143,6.71674984393641));
#78504=CARTESIAN_POINT('Ctrl Pts',(-1.68382124837509,7.5090544312736,6.55795624239888));
#78505=CARTESIAN_POINT('Ctrl Pts',(2.11394185586056,7.3994866226212,6.39916264086138));
#78506=CARTESIAN_POINT('Ctrl Pts',(5.39643685175506,5.48631221799571,6.24036903932385));
#78507=CARTESIAN_POINT('Ctrl Pts',(7.36356368807721,2.23586275516634,6.08157543778634));
#78508=CARTESIAN_POINT('Ctrl Pts',(7.53584005503271,-1.55957273420444,5.92278183624882));
#78509=CARTESIAN_POINT('Ctrl Pts',(5.87127401350223,-4.97486621997847,5.7639882347113));
#78510=CARTESIAN_POINT('Ctrl Pts',(2.7755994265296,-7.17754834687707,5.60519463317378));
#78511=CARTESIAN_POINT('Ctrl Pts',(-0.996620668095368,-7.63072078458088,
5.44640103163627));
#78512=CARTESIAN_POINT('Ctrl Pts',(-4.52591693538818,-6.22392387021847,
5.28760743009874));
#78513=CARTESIAN_POINT('Ctrl Pts',(-6.95203212353196,-3.30006087848231,
5.12881382856124));
#78514=CARTESIAN_POINT('Ctrl Pts',(-7.68360664515343,0.428183804998338,
4.97002022702371));
#78515=CARTESIAN_POINT('Ctrl Pts',(-6.54232101676206,4.05205974313583,4.81122662548621));
#78516=CARTESIAN_POINT('Ctrl Pts',(-3.80636079260434,6.68825612284975,4.65243302394867));
#78517=CARTESIAN_POINT('Ctrl Pts',(-0.14260952261873,7.69420658498056,4.49363942241117));
#78518=CARTESIAN_POINT('Ctrl Pts',(3.55590246642325,6.82471318793792,4.33484582087364));
#78519=CARTESIAN_POINT('Ctrl Pts',(6.38767200829543,4.29171280058643,4.17605221933613));
#78520=CARTESIAN_POINT('Ctrl Pts',(7.66246226841205,0.712618013736859,4.01725861779861));
#78521=CARTESIAN_POINT('Ctrl Pts',(7.06954626813712,-3.04017565462741,3.8584650162611));
#78522=CARTESIAN_POINT('Ctrl Pts',(4.75344581873176,-6.0519340129028,3.69967141472358));
#78523=CARTESIAN_POINT('Ctrl Pts',(1.27870468657267,-7.58854839698333,3.54087781318606));
#78524=CARTESIAN_POINT('Ctrl Pts',(-2.50771755594459,-7.27547284420542,
3.38208421164855));
#78525=CARTESIAN_POINT('Ctrl Pts',(-5.68288983550449,-5.18901874806867,
3.22329061011102));
#78526=CARTESIAN_POINT('Ctrl Pts',(-7.47287174771356,-1.83775414246081,
3.06449700857351));
#78527=CARTESIAN_POINT('Ctrl Pts',(-7.4413596212823,1.96145849706257,2.90570340703599));
#78528=CARTESIAN_POINT('Ctrl Pts',(-5.59603445805296,5.28257047275981,2.74690980549847));
#78529=CARTESIAN_POINT('Ctrl Pts',(-2.38668971302865,7.31606893318352,2.58811620396096));
#78530=CARTESIAN_POINT('Ctrl Pts',(1.40440476016309,7.56629366226348,2.42932260242343));
#78531=CARTESIAN_POINT('Ctrl Pts',(4.85317903440706,5.97225297401905,2.27052900088592));
#78532=CARTESIAN_POINT('Ctrl Pts',(7.1190029125058,2.92249040196356,2.1117353993484));
#78533=CARTESIAN_POINT('Ctrl Pts',(7.64958738353084,-0.839622057142283,
1.95294179781089));
#78534=CARTESIAN_POINT('Ctrl Pts',(6.3156038607506,-4.39707858135161,1.79414819627337));
#78535=CARTESIAN_POINT('Ctrl Pts',(3.44220740038646,-6.88275831554759,1.63535459473586));
#78536=CARTESIAN_POINT('Ctrl Pts',(-0.270218440699842,-7.69078219456233,
1.47656099319833));
#78537=CARTESIAN_POINT('Ctrl Pts',(-3.91677954782813,-6.62419790101118,
1.31776739166082));
#78538=CARTESIAN_POINT('Ctrl Pts',(-6.60863463382164,-3.94297975645974,
1.1589737901233));
#78539=CARTESIAN_POINT('Ctrl Pts',(-7.68965267397435,-0.300673899783249,
1.00018018858579));
#78540=CARTESIAN_POINT('Ctrl Pts',(-6.89633424263845,3.41492808781878,0.841386587048263));
#78541=CARTESIAN_POINT('Ctrl Pts',(-4.42205651323531,6.29813481547409,0.682592985510749));
#78542=CARTESIAN_POINT('Ctrl Pts',(-0.869903300828535,7.64621617687067,
0.523799383973227));
#78543=CARTESIAN_POINT('Ctrl Pts',(2.89426677637707,7.13049329930227,0.365005782435713));
#78544=CARTESIAN_POINT('Ctrl Pts',(5.95300565223129,4.87684424728084,0.206212180898193));
#78545=CARTESIAN_POINT('Ctrl Pts',(7.56063700490841,1.43425198886865,0.0474185793606738));
#78546=CARTESIAN_POINT('Ctrl Pts',(7.32553367271641,-2.35749082569408,-0.111375022176839));
#78547=CARTESIAN_POINT('Ctrl Pts',(5.30454760347664,-5.57551314506993,-0.27016862371436));
#78548=CARTESIAN_POINT('Ctrl Pts',(3.09565801023329,-6.81334794853324,-0.376031024739368));
#78549=CARTESIAN_POINT('Ctrl Pts',(1.9098669251939,-7.13093641674461,-0.428962225251874));
#78550=CARTESIAN_POINT('Ctrl Pts',(5.87252147387267,5.06342934200153,20.4288655727486));
#78551=CARTESIAN_POINT('Ctrl Pts',(6.71465610013426,4.08673215622288,20.3759253221903));
#78552=CARTESIAN_POINT('Ctrl Pts',(7.90122216432793,1.70622070396583,20.2700538711195));
#78553=CARTESIAN_POINT('Ctrl Pts',(7.75405346188429,-2.28265951451358,20.1112512195362));
#78554=CARTESIAN_POINT('Ctrl Pts',(5.71713861089972,-5.71394935700779,19.9524576179987));
#78555=CARTESIAN_POINT('Ctrl Pts',(2.28655434086387,-7.75295417769812,19.7936640164612));
#78556=CARTESIAN_POINT('Ctrl Pts',(-1.70130617882531,-7.90195509637086,
19.6348704149237));
#78557=CARTESIAN_POINT('Ctrl Pts',(-5.27451085437171,-6.12499607887182,
19.4760768133862));
#78558=CARTESIAN_POINT('Ctrl Pts',(-7.56204959034188,-2.85502232293436,
19.3172832118486));
#78559=CARTESIAN_POINT('Ctrl Pts',(-8.00636602006724,1.11082452361824,19.1584896103111));
#78560=CARTESIAN_POINT('Ctrl Pts',(-6.49914612100703,4.80592667525467,18.9996960087736));
#78561=CARTESIAN_POINT('Ctrl Pts',(-3.40777762609777,7.32958791044281,18.8409024072361));
#78562=CARTESIAN_POINT('Ctrl Pts',(0.514229383332149,8.0666843337605,18.6821088056986));
#78563=CARTESIAN_POINT('Ctrl Pts',(4.31089367491321,6.83754425870798,18.5233152041611));
#78564=CARTESIAN_POINT('Ctrl Pts',(7.05678856865421,3.94177072295006,18.3645216026235));
#78565=CARTESIAN_POINT('Ctrl Pts',(8.08260852233796,0.0851997604627655,
18.205728001086));
#78566=CARTESIAN_POINT('Ctrl Pts',(7.1383126791028,-3.79213815638369,18.0469343995485));
#78567=CARTESIAN_POINT('Ctrl Pts',(4.45407070540305,-6.74515190064075,17.888140798011));
#78568=CARTESIAN_POINT('Ctrl Pts',(0.684160013267999,-8.05405145038072,
17.7293471964735));
#78569=CARTESIAN_POINT('Ctrl Pts',(-3.25251300293659,-7.39979587979247,
17.570553594936));
#78570=CARTESIAN_POINT('Ctrl Pts',(-6.39639399962379,-4.94185831406292,
17.4117599933984));
#78571=CARTESIAN_POINT('Ctrl Pts',(-7.98116975326553,-1.27935499443613,
17.2529663918609));
#78572=CARTESIAN_POINT('Ctrl Pts',(-7.62055508262866,2.6949879513174,17.0941727903234));
#78573=CARTESIAN_POINT('Ctrl Pts',(-5.40244892534212,6.01243423505299,16.9353791887859));
#78574=CARTESIAN_POINT('Ctrl Pts',(-1.86750918005211,7.86436451908362,16.7765855872484));
#78575=CARTESIAN_POINT('Ctrl Pts',(2.12263131708691,7.79937536696847,16.6177919857108));
#78576=CARTESIAN_POINT('Ctrl Pts',(5.59538567125106,5.83330772503389,16.4589983841733));
#78577=CARTESIAN_POINT('Ctrl Pts',(7.70427858222301,2.4453857265756,16.3002047826358));
#78578=CARTESIAN_POINT('Ctrl Pts',(7.93527260957988,-1.53859300533986,16.1414111810983));
#78579=CARTESIAN_POINT('Ctrl Pts',(6.23206352941125,-5.1475434908152,15.9826175795608));
#78580=CARTESIAN_POINT('Ctrl Pts',(3.00980435004202,-7.50179295894329,15.8238239780233));
#78581=CARTESIAN_POINT('Ctrl Pts',(-0.94608720886968,-8.02749891421056,
15.6650303764857));
#78582=CARTESIAN_POINT('Ctrl Pts',(-4.67137234637402,-6.5965218278983,15.5062367749482));
#78583=CARTESIAN_POINT('Ctrl Pts',(-7.2580220074112,-3.55765883192241,15.3474431734107));
#78584=CARTESIAN_POINT('Ctrl Pts',(-8.07554672317612,0.348374720977148,
15.1886495718732));
#78585=CARTESIAN_POINT('Ctrl Pts',(-6.92467686255512,4.16949279572595,15.0298559703357));
#78586=CARTESIAN_POINT('Ctrl Pts',(-4.08593411273857,6.97430729540769,14.8710623687981));
#78587=CARTESIAN_POINT('Ctrl Pts',(-0.251255010538211,8.07915161041654,
14.7122687672607));
#78588=CARTESIAN_POINT('Ctrl Pts',(3.64466688016764,7.21472266667448,14.5534751657231));
#78589=CARTESIAN_POINT('Ctrl Pts',(6.65221021700204,4.5917228850651,14.3946815641856));
#78590=CARTESIAN_POINT('Ctrl Pts',(8.03829373681283,0.849501986538545,14.2358879626481));
#78591=CARTESIAN_POINT('Ctrl Pts',(7.46506300369113,-3.09978292390594,14.0770943611106));
#78592=CARTESIAN_POINT('Ctrl Pts',(5.07224159360946,-6.29350339957605,13.9183007595731));
#78593=CARTESIAN_POINT('Ctrl Pts',(1.44307381773593,-7.95319795937345,13.7595071580355));
#78594=CARTESIAN_POINT('Ctrl Pts',(-2.53783963846463,-7.67432015189977,
13.600713556498));
#78595=CARTESIAN_POINT('Ctrl Pts',(-5.90016094835825,-5.52484575421662,
13.4419199549605));
#78596=CARTESIAN_POINT('Ctrl Pts',(-7.82433259375634,-2.0287038440096,13.283126353423));
#78597=CARTESIAN_POINT('Ctrl Pts',(-7.84134248660204,1.96192961959055,13.1243327518854));
#78598=CARTESIAN_POINT('Ctrl Pts',(-5.94704450750926,5.47434758214355,12.965539150348));
#78599=CARTESIAN_POINT('Ctrl Pts',(-2.60316911212683,7.65240683694259,12.8067455488104));
#78600=CARTESIAN_POINT('Ctrl Pts',(1.37522232747844,7.96521081795215,12.6479519472729));
#78601=CARTESIAN_POINT('Ctrl Pts',(5.01840671999116,6.33651432707009,12.4891583457354));
#78602=CARTESIAN_POINT('Ctrl Pts',(7.43836686424581,3.1633081129266,12.3303647441979));
#78603=CARTESIAN_POINT('Ctrl Pts',(8.04524344962119,-0.780946643980331,
12.1715711426604));
#78604=CARTESIAN_POINT('Ctrl Pts',(6.691111806725,-4.53484758446439,12.0127775411229));
#78605=CARTESIAN_POINT('Ctrl Pts',(3.70603818035271,-7.18339062213555,11.8539839395853));
#78606=CARTESIAN_POINT('Ctrl Pts',(-0.182373102793984,-8.08099993044143,
11.6951903380478));
#78607=CARTESIAN_POINT('Ctrl Pts',(-4.02633139238815,-7.00888545655346,
11.5363967365103));
#78608=CARTESIAN_POINT('Ctrl Pts',(-6.88888134553315,-4.22837245658215,
11.3776031349728));
#78609=CARTESIAN_POINT('Ctrl Pts',(-8.07228347838272,-0.41720410957528,
11.2188095334353));
#78610=CARTESIAN_POINT('Ctrl Pts',(-7.28808644270806,3.49565670912235,11.0600159318977));
#78611=CARTESIAN_POINT('Ctrl Pts',(-4.72743632988278,6.55645983525572,10.9012223303602));
#78612=CARTESIAN_POINT('Ctrl Pts',(-1.01448528302337,8.01914206352189,10.7424287288227));
#78613=CARTESIAN_POINT('Ctrl Pts',(2.94574404695163,7.52717821193747,10.5836351272852));
#78614=CARTESIAN_POINT('Ctrl Pts',(6.18795553810953,5.20048325473668,10.4248415257477));
#78615=CARTESIAN_POINT('Ctrl Pts',(7.92186814404438,1.60618334345491,10.2660479242102));
#78616=CARTESIAN_POINT('Ctrl Pts',(7.72484494784568,-2.37961979235341,10.1072543226726));
#78617=CARTESIAN_POINT('Ctrl Pts',(5.64490986716436,-5.78539647872188,9.94846072113507));
#78618=CARTESIAN_POINT('Ctrl Pts',(2.18904194284954,-7.78099705673138,9.78966711959756));
#78619=CARTESIAN_POINT('Ctrl Pts',(-1.80039955059843,-7.87999881234902,
9.63087351806003));
#78620=CARTESIAN_POINT('Ctrl Pts',(-5.3509980985211,-6.05827031206438,9.47207991652253));
#78621=CARTESIAN_POINT('Ctrl Pts',(-7.59730407079027,-2.75985338023062,
9.31328631498499));
#78622=CARTESIAN_POINT('Ctrl Pts',(-7.99178593247863,1.21127099934486,9.15449271344749));
#78623=CARTESIAN_POINT('Ctrl Pts',(-6.43828970371974,4.88715106328761,8.99569911190997));
#78624=CARTESIAN_POINT('Ctrl Pts',(-3.31547625491016,7.37180012124203,8.83690551037245));
#78625=CARTESIAN_POINT('Ctrl Pts',(0.615476345589656,8.05959109958046,8.67811190883494));
#78626=CARTESIAN_POINT('Ctrl Pts',(4.39640810637647,6.78287664539203,8.51931830729741));
#78627=CARTESIAN_POINT('Ctrl Pts',(7.10572624534672,3.85285275485684,8.36052470575991));
#78628=CARTESIAN_POINT('Ctrl Pts',(8.08304115505151,-0.0162944825236051,
8.20173110422238));
#78629=CARTESIAN_POINT('Ctrl Pts',(7.09013473910324,-3.88146998001768,8.04293750268486));
#78630=CARTESIAN_POINT('Ctrl Pts',(4.36902548504316,-6.80054675268545,7.88414390114735));
#78631=CARTESIAN_POINT('Ctrl Pts',(0.582977055512693,-8.06200704397873,
7.72535029960982));
#78632=CARTESIAN_POINT('Ctrl Pts',(-3.3451705920107,-7.35837302226273,7.56655669807232));
#78633=CARTESIAN_POINT('Ctrl Pts',(-6.45794116648677,-4.86115374315731,
7.40776309653478));
#78634=CARTESIAN_POINT('Ctrl Pts',(-7.99660452537937,-1.17904024066161,
7.24896949499729));
#78635=CARTESIAN_POINT('Ctrl Pts',(-7.5861152737016,2.79046140961099,7.09017589345975));
#78636=CARTESIAN_POINT('Ctrl Pts',(-5.32652915310981,6.07979498054733,6.93138229192225));
#78637=CARTESIAN_POINT('Ctrl Pts',(-1.76861470189815,7.88719353513318,6.77258869038473));
#78638=CARTESIAN_POINT('Ctrl Pts',(2.22039521644045,7.77210813790092,6.61379508884721));
#78639=CARTESIAN_POINT('Ctrl Pts',(5.66818928261491,5.76259057029618,6.45500148730969));
#78640=CARTESIAN_POINT('Ctrl Pts',(7.73437620511342,2.3484557782067,6.29620788577219));
#78641=CARTESIAN_POINT('Ctrl Pts',(7.91532802270162,-1.63810931181399,6.13741428423465));
#78642=CARTESIAN_POINT('Ctrl Pts',(6.16693817658691,-5.2253893013413,5.97862068269715));
#78643=CARTESIAN_POINT('Ctrl Pts',(2.91537237523135,-7.53899354941726,5.81982708115961));
#78644=CARTESIAN_POINT('Ctrl Pts',(-1.04680824494286,-8.01498673253654,
5.66103347962212));
#78645=CARTESIAN_POINT('Ctrl Pts',(-4.7538319398344,-6.53734668747398,5.50223987808458));
#78646=CARTESIAN_POINT('Ctrl Pts',(-7.30212083593321,-3.46624452712843,
5.34344627654708));
#78647=CARTESIAN_POINT('Ctrl Pts',(-8.07053580618163,0.449746179035062,
5.18465267500954));
#78648=CARTESIAN_POINT('Ctrl Pts',(-6.87177759869027,4.25611236441841,5.02585907347205));
#78649=CARTESIAN_POINT('Ctrl Pts',(-3.99804056696941,7.02506166871776,4.86706547193452));
#78650=CARTESIAN_POINT('Ctrl Pts',(-0.149791017649627,8.08166953515412,
4.70827187039701));
#78651=CARTESIAN_POINT('Ctrl Pts',(3.73496972241026,7.16839040490381,4.54947826885948));
#78652=CARTESIAN_POINT('Ctrl Pts',(6.70934081374529,4.50783381119964,4.39068466732197));
#78653=CARTESIAN_POINT('Ctrl Pts',(8.04832664615152,0.748503855233274,4.23189106578445));
#78654=CARTESIAN_POINT('Ctrl Pts',(7.42555272873669,-3.19327206751645,4.07309746424694));
#78655=CARTESIAN_POINT('Ctrl Pts',(4.9928186663508,-6.35669580750712,3.91430386270942));
#78656=CARTESIAN_POINT('Ctrl Pts',(1.34309738058055,-7.97069063828595,3.7555102611719));
#78657=CARTESIAN_POINT('Ctrl Pts',(-2.63400057573315,-7.64184930433663,
3.59671665963439));
#78658=CARTESIAN_POINT('Ctrl Pts',(-5.96906739479618,-5.45032606941837,
3.43792305809687));
#78659=CARTESIAN_POINT('Ctrl Pts',(-7.84918877295303,-1.9302993105515,3.27912945655935));
#78660=CARTESIAN_POINT('Ctrl Pts',(-7.81608976666111,2.06023313841395,3.12033585502182));
#78661=CARTESIAN_POINT('Ctrl Pts',(-5.87783817575176,5.54858884869876,2.96154225348432));
#78662=CARTESIAN_POINT('Ctrl Pts',(-2.50687804266929,7.68448972111217,2.8027486519468));
#78663=CARTESIAN_POINT('Ctrl Pts',(1.47512742735437,7.94731520514522,2.64395505040928));
#78664=CARTESIAN_POINT('Ctrl Pts',(5.09757422260781,6.27300221059572,2.48516144887177));
#78665=CARTESIAN_POINT('Ctrl Pts',(7.47749989855737,3.06966045003703,2.32636784733424));
#78666=CARTESIAN_POINT('Ctrl Pts',(8.03480341100519,-0.88190353681118,2.16757424579673));
#78667=CARTESIAN_POINT('Ctrl Pts',(6.63364347627,-4.61850557586475,2.00878064425921));
#78668=CARTESIAN_POINT('Ctrl Pts',(3.61554922838812,-7.22935855467807,1.8499870427217));
#78669=CARTESIAN_POINT('Ctrl Pts',(-0.283826034032366,-8.07807270013105,
1.69119344118417));
#78670=CARTESIAN_POINT('Ctrl Pts',(-4.11401976252985,-6.95777761880423,
1.53239983964667));
#78671=CARTESIAN_POINT('Ctrl Pts',(-6.94143062045892,-4.14153935478073,
1.37360623810914));
#78672=CARTESIAN_POINT('Ctrl Pts',(-8.07688629942497,-0.315815161583738,
1.21481263657163));
#78673=CARTESIAN_POINT('Ctrl Pts',(-7.24361813494408,3.58689619095233,1.05601903503411));
#78674=CARTESIAN_POINT('Ctrl Pts',(-4.64474134025788,6.61529472913664,0.897225433496593));
#78675=CARTESIAN_POINT('Ctrl Pts',(-0.913709675869558,8.03126243795472,
0.73843183195907));
#78676=CARTESIAN_POINT('Ctrl Pts',(3.04001554610122,7.48956891540719,0.579638230421557));
#78677=CARTESIAN_POINT('Ctrl Pts',(6.25278563694289,5.12243116241214,0.420844628884037));
#78678=CARTESIAN_POINT('Ctrl Pts',(7.94137369123961,1.50647769541312,0.262051027346517));
#78679=CARTESIAN_POINT('Ctrl Pts',(7.69443108365505,-2.4762087649958,0.103257425809005));
#78680=CARTESIAN_POINT('Ctrl Pts',(5.57167269832283,-5.85628345557045,-0.0555361757285161));
#78681=CARTESIAN_POINT('Ctrl Pts',(3.25154838984888,-7.15645283758716,-0.161398576753524));
#78682=CARTESIAN_POINT('Ctrl Pts',(2.00604353094284,-7.49003434724797,-0.214329777266031));
#78683=CARTESIAN_POINT('Ctrl Pts',(6.15407029065202,5.30618750754062,20.6434980207344));
#78684=CARTESIAN_POINT('Ctrl Pts',(7.03657973864013,4.28266410950697,20.5905577701761));
#78685=CARTESIAN_POINT('Ctrl Pts',(8.28003384877634,1.78802277527426,20.4846863191053));
#78686=CARTESIAN_POINT('Ctrl Pts',(8.12580937408491,-2.39209803905211,20.325883667522));
#78687=CARTESIAN_POINT('Ctrl Pts',(5.9912378404085,-5.98789568274879,20.1670900659845));
#78688=CARTESIAN_POINT('Ctrl Pts',(2.39617959673327,-8.12465738644534,20.008296464447));
#78689=CARTESIAN_POINT('Ctrl Pts',(-1.78287263094621,-8.28080192009469,
19.8495028629095));
#78690=CARTESIAN_POINT('Ctrl Pts',(-5.52738899142837,-6.41864939396941,
19.6907092613719));
#78691=CARTESIAN_POINT('Ctrl Pts',(-7.92460017854491,-2.9919018831841,19.5319156598344));
#78692=CARTESIAN_POINT('Ctrl Pts',(-8.39021866150606,1.16408126038211,19.3731220582969));
#78693=CARTESIAN_POINT('Ctrl Pts',(-6.81073747211346,5.03633927995374,19.2143284567594));
#78694=CARTESIAN_POINT('Ctrl Pts',(-3.57115817102104,7.68099348858274,19.0555348552219));
#78695=CARTESIAN_POINT('Ctrl Pts',(0.538883303300684,8.45342884199385,18.8967412536844));
#78696=CARTESIAN_POINT('Ctrl Pts',(4.51757270007016,7.16535957692872,18.7379476521468));
#78697=CARTESIAN_POINT('Ctrl Pts',(7.39511521089914,4.13075272803929,18.5791540506093));
#78698=CARTESIAN_POINT('Ctrl Pts',(8.47011649077696,0.0892845291357988,
18.4203604490718));
#78699=CARTESIAN_POINT('Ctrl Pts',(7.48054786675499,-3.97394626313031,18.2615668475343));
#78700=CARTESIAN_POINT('Ctrl Pts',(4.66761412836659,-7.06853761239531,18.1027732459967));
#78701=CARTESIAN_POINT('Ctrl Pts',(0.716960990340684,-8.44019029486573,
17.9439796444593));
#78702=CARTESIAN_POINT('Ctrl Pts',(-3.40844962941133,-7.75456746873147,
17.7851860429217));
#78703=CARTESIAN_POINT('Ctrl Pts',(-6.70305906168629,-5.17878794764635,
17.6263924413842));
#78704=CARTESIAN_POINT('Ctrl Pts',(-8.36381439927396,-1.34069165987479,
17.4675988398467));
#78705=CARTESIAN_POINT('Ctrl Pts',(-7.98591062475169,2.82419491502181,17.3088052383092));
#78706=CARTESIAN_POINT('Ctrl Pts',(-5.66146085223045,6.30069094937478,17.1500116367717));
#78707=CARTESIAN_POINT('Ctrl Pts',(-1.95704397397453,8.24140912163137,16.9912180352342));
#78708=CARTESIAN_POINT('Ctrl Pts',(2.22439754109196,8.17330416671108,16.8324244336966));
#78709=CARTESIAN_POINT('Ctrl Pts',(5.86364764733302,6.11297650022698,16.6736308321591));
#78710=CARTESIAN_POINT('Ctrl Pts',(8.07364811601082,2.5626259037209,16.5148372306216));
#78711=CARTESIAN_POINT('Ctrl Pts',(8.31571678913525,-1.61235842996804,16.3560436290841));
#78712=CARTESIAN_POINT('Ctrl Pts',(6.53085002523011,-5.39433437708224,16.1972500275466));
#78713=CARTESIAN_POINT('Ctrl Pts',(3.1541046914306,-7.86145463761249,16.038456426009));
#78714=CARTESIAN_POINT('Ctrl Pts',(-0.991445873867747,-8.41236473906092,
15.8796628244715));
#78715=CARTESIAN_POINT('Ctrl Pts',(-4.89533395514954,-6.9127817043018,15.720869222934));
#78716=CARTESIAN_POINT('Ctrl Pts',(-7.60599647075488,-3.72822519580695,
15.5620756213965));
#78717=CARTESIAN_POINT('Ctrl Pts',(-8.46271612474785,0.365076999704155,
15.403282019859));
#78718=CARTESIAN_POINT('Ctrl Pts',(-7.25666961658859,4.36939257786033,15.2444884183215));
#78719=CARTESIAN_POINT('Ctrl Pts',(-4.28182780508147,7.30867950257863,15.0856948167839));
#78720=CARTESIAN_POINT('Ctrl Pts',(-0.26330103731591,8.46649384264402,14.9269012152464));
#78721=CARTESIAN_POINT('Ctrl Pts',(3.81940470824224,7.5606212111465,14.7681076137089));
#78722=CARTESIAN_POINT('Ctrl Pts',(6.97113998573889,4.81186582554143,14.6093140121714));
#78723=CARTESIAN_POINT('Ctrl Pts',(8.423677102475,0.890230024779997,14.4505204106339));
#78724=CARTESIAN_POINT('Ctrl Pts',(7.82296372235575,-3.24839714666893,14.2917268090964));
#78725=CARTESIAN_POINT('Ctrl Pts',(5.31542224870852,-6.59523553345258,14.1329332075588));
#78726=CARTESIAN_POINT('Ctrl Pts',(1.51225972496784,-8.33450154166531,13.9741396060213));
#78727=CARTESIAN_POINT('Ctrl Pts',(-2.65951237317739,-8.04225337580815,
13.8153460044838));
#78728=CARTESIAN_POINT('Ctrl Pts',(-6.18303489632227,-5.78972580478921,
13.6565524029463));
#78729=CARTESIAN_POINT('Ctrl Pts',(-8.19945792853139,-2.1259668628709,13.4977588014087));
#78730=CARTESIAN_POINT('Ctrl Pts',(-8.21728333396832,2.0559912531593,13.3389651998713));
#78731=CARTESIAN_POINT('Ctrl Pts',(-6.23216621406629,5.7368065771849,13.1801715983337));
#78732=CARTESIAN_POINT('Ctrl Pts',(-2.72797396582666,8.01928946138952,13.0213779967962));
#78733=CARTESIAN_POINT('Ctrl Pts',(1.4411552015995,8.34709033787726,12.8625843952587));
#78734=CARTESIAN_POINT('Ctrl Pts',(5.25900634664509,6.64030855229842,12.7037907937212));
#78735=CARTESIAN_POINT('Ctrl Pts',(7.79498767844233,3.31496795108393,12.5449971921837));
#78736=CARTESIAN_POINT('Ctrl Pts',(8.4309600083465,-0.81838790401807,12.3862035906461));
#78737=CARTESIAN_POINT('Ctrl Pts',(7.01190665106966,-4.75226372800019,12.2274099891087));
#78738=CARTESIAN_POINT('Ctrl Pts',(3.88371835900504,-7.52778700095242,12.0686163875711));
#78739=CARTESIAN_POINT('Ctrl Pts',(-0.191116694713139,-8.46843077746894,
11.9098227860336));
#78740=CARTESIAN_POINT('Ctrl Pts',(-4.21936752593521,-7.34491545934086,
11.7510291844961));
#78741=CARTESIAN_POINT('Ctrl Pts',(-7.21915793973503,-4.43109513156081,
11.5922355829586));
#78742=CARTESIAN_POINT('Ctrl Pts',(-8.45929642880916,-0.437206305212873,
11.4334419814211));
#78743=CARTESIAN_POINT('Ctrl Pts',(-7.63750229817309,3.66325047862986,11.2746483798835));
#78744=CARTESIAN_POINT('Ctrl Pts',(-4.95408583827537,6.87079900235633,11.115854778346));
#78745=CARTESIAN_POINT('Ctrl Pts',(-1.06312318623855,8.40360723229395,10.9570611768085));
#78746=CARTESIAN_POINT('Ctrl Pts',(3.08697311774242,7.88805694668319,10.798267575271));
#78747=CARTESIAN_POINT('Ctrl Pts',(6.48462734557574,5.44981225482057,10.6394739737334));
#78748=CARTESIAN_POINT('Ctrl Pts',(8.30166966755703,1.68318928066475,10.4806803721959));
#78749=CARTESIAN_POINT('Ctrl Pts',(8.09520050372507,-2.49370692509573,10.3218867706584));
#78750=CARTESIAN_POINT('Ctrl Pts',(5.91554620302062,-6.06276822447546,10.1630931691209));
#78751=CARTESIAN_POINT('Ctrl Pts',(2.29399211998073,-8.15404473726062,10.0042995675834));
#78752=CARTESIAN_POINT('Ctrl Pts',(-1.88671687876084,-8.25779297652708,
9.84550596604586));
#78753=CARTESIAN_POINT('Ctrl Pts',(-5.60754329634285,-6.3487245650935,9.68671236450838));
#78754=CARTESIAN_POINT('Ctrl Pts',(-7.96154487967629,-2.8921702150256,9.52791876297083));
#78755=CARTESIAN_POINT('Ctrl Pts',(-8.37493955452223,1.26934348459364,9.36912516143335));
#78756=CARTESIAN_POINT('Ctrl Pts',(-6.74696338950016,5.12145784367357,9.2103315598958));
#78757=CARTESIAN_POINT('Ctrl Pts',(-3.47443155559029,7.72522949751655,9.05153795835831));
#78758=CARTESIAN_POINT('Ctrl Pts',(0.644984392112331,8.44599553384399,8.89274435682078));
#78759=CARTESIAN_POINT('Ctrl Pts',(4.60718698661326,7.10807101077098,8.73395075528327));
#78760=CARTESIAN_POINT('Ctrl Pts',(7.44639912762328,4.03757172764921,8.57515715374574));
#78761=CARTESIAN_POINT('Ctrl Pts',(8.47056986538634,-0.0170756958908047,
8.41636355220823));
#78762=CARTESIAN_POINT('Ctrl Pts',(7.43006011110603,-4.06756096071491,8.2575699506707));
#78763=CARTESIAN_POINT('Ctrl Pts',(4.57849154851613,-7.12658828360019,8.09877634913321));
#78764=CARTESIAN_POINT('Ctrl Pts',(0.610926974626544,-8.44852730690116,
7.93998274759565));
#78765=CARTESIAN_POINT('Ctrl Pts',(-3.50554954103556,-7.71115865736963,
7.78118914605817));
#78766=CARTESIAN_POINT('Ctrl Pts',(-6.76755701077859,-5.09421412286944,
7.62239554452063));
#78767=CARTESIAN_POINT('Ctrl Pts',(-8.37998916728995,-1.23556747281741,
7.46360194298313));
#78768=CARTESIAN_POINT('Ctrl Pts',(-7.94981965328795,2.92424569829173,7.30480834144559));
#78769=CARTESIAN_POINT('Ctrl Pts',(-5.58190122578267,6.37128119999322,7.14601473990809));
#78770=CARTESIAN_POINT('Ctrl Pts',(-1.8534081554212,8.26533263899277,6.98722113837056));
#78771=CARTESIAN_POINT('Ctrl Pts',(2.32684857702034,8.14472965318062,6.82842753683306));
#78772=CARTESIAN_POINT('Ctrl Pts',(5.93994171347475,6.03886892259665,6.66963393529553));
#78773=CARTESIAN_POINT('Ctrl Pts',(8.10518872214963,2.46104880124704,6.51084033375802));
#78774=CARTESIAN_POINT('Ctrl Pts',(8.29481599037053,-1.71664588942351,6.3520467322205));
#78775=CARTESIAN_POINT('Ctrl Pts',(6.46260233967159,-5.47591238270415,6.19325313068298));
#78776=CARTESIAN_POINT('Ctrl Pts',(3.0551453239331,-7.90043875195744,6.03445952914546));
#78777=CARTESIAN_POINT('Ctrl Pts',(-1.09699582179035,-8.39925268049223,
5.87566592760795));
#78778=CARTESIAN_POINT('Ctrl Pts',(-4.98174694428061,-6.85076950472949,
5.71687232607043));
#78779=CARTESIAN_POINT('Ctrl Pts',(-7.65220954833444,-3.63242817577456,
5.55807872453291));
#78780=CARTESIAN_POINT('Ctrl Pts',(-8.45746496720986,0.471308553071791,
5.3992851229954));
#78781=CARTESIAN_POINT('Ctrl Pts',(-7.20123418061844,4.46016498570097,5.24049152145787));
#78782=CARTESIAN_POINT('Ctrl Pts',(-4.18972034133451,7.36186721458578,5.08169791992036));
#78783=CARTESIAN_POINT('Ctrl Pts',(-0.156972512680516,8.46913248532767,
4.92290431838285));
#78784=CARTESIAN_POINT('Ctrl Pts',(3.91403697839729,7.51206762186971,4.76411071684532));
#78785=CARTESIAN_POINT('Ctrl Pts',(7.03100961919515,4.72395482181285,4.60531711530781));
#78786=CARTESIAN_POINT('Ctrl Pts',(8.434191023891,0.78438969672969,4.44652351377029));
#78787=CARTESIAN_POINT('Ctrl Pts',(7.78155918933625,-3.34636848040548,4.28772991223278));
#78788=CARTESIAN_POINT('Ctrl Pts',(5.23219151396984,-6.66145760211143,4.12893631069526));
#78789=CARTESIAN_POINT('Ctrl Pts',(1.40749007458845,-8.3528328795886,3.97014270915774));
#78790=CARTESIAN_POINT('Ctrl Pts',(-2.7602835955217,-8.00822576446783,3.81134910762023));
#78791=CARTESIAN_POINT('Ctrl Pts',(-6.25524495408788,-5.7116333907681,3.65255550608271));
#78792=CARTESIAN_POINT('Ctrl Pts',(-8.22550579819248,-2.02284447864219,
3.49376190454519));
#78793=CARTESIAN_POINT('Ctrl Pts',(-8.19081991203992,2.15900777976532,3.33496830300767));
#78794=CARTESIAN_POINT('Ctrl Pts',(-6.15964189345056,5.81460722463769,3.17617470147015));
#78795=CARTESIAN_POINT('Ctrl Pts',(-2.62706637230996,8.05291050904083,3.01738109993264));
#78796=CARTESIAN_POINT('Ctrl Pts',(1.54585009454566,8.32833674802694,2.85858749839512));
#78797=CARTESIAN_POINT('Ctrl Pts',(5.34196941080857,6.57375144717241,2.6997938968576));
#78798=CARTESIAN_POINT('Ctrl Pts',(7.83599688460893,3.21683049811048,2.54100029532008));
#78799=CARTESIAN_POINT('Ctrl Pts',(8.42001943847956,-0.924185016480067,
2.38220669378257));
#78800=CARTESIAN_POINT('Ctrl Pts',(6.95168309178937,-4.8399325703779,2.22341309224505));
#78801=CARTESIAN_POINT('Ctrl Pts',(3.78889105638979,-7.57595879380855,2.06461949070754));
#78802=CARTESIAN_POINT('Ctrl Pts',(-0.297433627364896,-8.46536320569979,
1.90582588917001));
#78803=CARTESIAN_POINT('Ctrl Pts',(-4.31125997723156,-7.29135733659727,
1.74703228763251));
#78804=CARTESIAN_POINT('Ctrl Pts',(-7.27422660709621,-4.34009895310173,
1.58823868609498));
#78805=CARTESIAN_POINT('Ctrl Pts',(-8.46411992487559,-0.33095642338422,
1.42944508455747));
#78806=CARTESIAN_POINT('Ctrl Pts',(-7.5909020272497,3.75886429408588,1.27065148301995));
#78807=CARTESIAN_POINT('Ctrl Pts',(-4.86742616728046,6.93245464279921,1.11185788148243));
#78808=CARTESIAN_POINT('Ctrl Pts',(-0.957516050910578,8.41630869903879,
0.953064279944913));
#78809=CARTESIAN_POINT('Ctrl Pts',(3.18576431582538,7.8486445315121,0.7942706784074));
#78810=CARTESIAN_POINT('Ctrl Pts',(6.55256562165449,5.36801807754346,0.635477076869881));
#78811=CARTESIAN_POINT('Ctrl Pts',(8.32211037757082,1.57870340195759,0.476683475332361));
#78812=CARTESIAN_POINT('Ctrl Pts',(8.06332849459369,-2.5949267042975,0.317889873794848));
#78813=CARTESIAN_POINT('Ctrl Pts',(5.83879779316903,-6.13705376607098,0.159096272257328));
#78814=CARTESIAN_POINT('Ctrl Pts',(3.40743876946447,-7.49955772664107,0.0532338712323191));
#78815=CARTESIAN_POINT('Ctrl Pts',(2.10222013669177,-7.84913227775134,0.000302670719812688));
#78816=CARTESIAN_POINT('',(5.31060265091893,4.57808054062544,-0.000178101097113292));
#78817=CARTESIAN_POINT('Ctrl Pts',(2.10208451021607,-7.84862588447237,0.));
#78818=CARTESIAN_POINT('Ctrl Pts',(2.29937946956078,-7.78117163610351,1.31601965385565E-15));
#78819=CARTESIAN_POINT('Ctrl Pts',(2.49362179095633,-7.70610038324866,-7.24771166142834E-15));
#78820=CARTESIAN_POINT('Ctrl Pts',(2.68444863542622,-7.6237268130433,-1.66533453693773E-15));
#78821=CARTESIAN_POINT('Ctrl Pts',(2.87762389604612,-7.54033951008384,3.98574227512031E-15));
#78822=CARTESIAN_POINT('Ctrl Pts',(3.06729970067492,-7.44946870591119,-1.02390292508958E-15));
#78823=CARTESIAN_POINT('Ctrl Pts',(3.25307750518592,-7.35139244187101,3.99680288865056E-15));
#78824=CARTESIAN_POINT('Ctrl Pts',(3.43854675272667,-7.25347907196647,9.00916984954207E-15));
#78825=CARTESIAN_POINT('Ctrl Pts',(3.62013148795847,-7.14838371410984,-3.77592803097428E-15));
#78826=CARTESIAN_POINT('Ctrl Pts',(3.79740460673799,-7.03634117918246,-3.77475828372553E-15));
#78827=CARTESIAN_POINT('Ctrl Pts',(3.97213881931131,-6.92590331781892,-3.77360528960083E-15));
#78828=CARTESIAN_POINT('Ctrl Pts',(4.14268447199419,-6.80871537035203,-2.49906849866478E-16));
#78829=CARTESIAN_POINT('Ctrl Pts',(4.30859563250671,-6.68496847023835,-4.10782519111308E-15));
#78830=CARTESIAN_POINT('Ctrl Pts',(4.45093652015492,-6.57880175094424,-7.41766594848549E-15));
#78831=CARTESIAN_POINT('Ctrl Pts',(4.5898657756993,-6.46780662798986,3.44670256380473E-15));
#78832=CARTESIAN_POINT('Ctrl Pts',(4.7250759146848,-6.35208741176991,-4.55191440096314E-15));
#78833=CARTESIAN_POINT('Ctrl Pts',(4.74406958653759,-6.33583173126817,-6.88917332012633E-15));
#78834=CARTESIAN_POINT('Ctrl Pts',(4.76298982572575,-6.31948280724091,4.34243815445731E-15));
#78835=CARTESIAN_POINT('Ctrl Pts',(4.78183573755202,-6.30304090823604,2.77555756156289E-15));
#78836=CARTESIAN_POINT('Ctrl Pts',(4.79992876259441,-6.28725585664597,1.83748770952108E-16));
#78837=CARTESIAN_POINT('Ctrl Pts',(4.81794637150894,-6.27139112825568,1.2337470547172E-15));
#78838=CARTESIAN_POINT('Ctrl Pts',(4.83588620584108,-6.25544870534714,5.55111512312578E-16));
#78839=CARTESIAN_POINT('Ctrl Pts',(4.98981908389951,-6.11865463043536,9.29425087228634E-16));
#78840=CARTESIAN_POINT('Ctrl Pts',(5.1380716025988,-5.97610601005547,-9.7440776070667E-15));
#78841=CARTESIAN_POINT('Ctrl Pts',(5.28026270051223,-5.82804960322368,-8.32667268468867E-16));
#78842=CARTESIAN_POINT('Ctrl Pts',(5.3246867667692,-5.78179306731262,-3.31589168886096E-15));
#78843=CARTESIAN_POINT('Ctrl Pts',(5.36851891763432,-5.73499864303366,8.03106703488735E-17));
#78844=CARTESIAN_POINT('Ctrl Pts',(5.41174677480464,-5.68767313410808,2.16493489801906E-15));
#78845=CARTESIAN_POINT('Ctrl Pts',(5.55047476155044,-5.53579485457413,1.98172015419112E-16));
#78846=CARTESIAN_POINT('Ctrl Pts',(5.68298237898118,-5.37844899954852,4.23059200690762E-15));
#78847=CARTESIAN_POINT('Ctrl Pts',(5.80904637428058,-5.2160751247644,1.18238752122579E-14));
#78848=CARTESIAN_POINT('Ctrl Pts',(5.93507004847681,-5.05375318466423,3.32743196074342E-15));
#78849=CARTESIAN_POINT('Ctrl Pts',(6.05465451261215,-4.8864057750382,-6.33296793918175E-15));
#78850=CARTESIAN_POINT('Ctrl Pts',(6.16753013306389,-4.71444913744807,2.66453525910038E-15));
#78851=CARTESIAN_POINT('Ctrl Pts',(6.27942834154928,-4.54398150585057,1.15841273260136E-14));
#78852=CARTESIAN_POINT('Ctrl Pts',(6.3847336068269,-4.36898347249209,-4.56776605346051E-15));
#78853=CARTESIAN_POINT('Ctrl Pts',(6.48313375932835,-4.18984791395913,-1.08246744900953E-14));
#78854=CARTESIAN_POINT('Ctrl Pts',(6.52516299014066,-4.11333451896046,-1.34971606821353E-14));
#78855=CARTESIAN_POINT('Ctrl Pts',(6.56593183983806,-4.03606618794043,-3.37372497907E-15));
#78856=CARTESIAN_POINT('Ctrl Pts',(6.60541304448959,-3.95807326746694,3.49720252756924E-15));
#78857=CARTESIAN_POINT('Ctrl Pts',(6.62089391761463,-3.92749166497638,6.19134415573078E-15));
#78858=CARTESIAN_POINT('Ctrl Pts',(6.63617853869402,-3.8967948930452,4.15509497561339E-15));
#78859=CARTESIAN_POINT('Ctrl Pts',(6.65125079271779,-3.86601480613085,3.71924713249427E-15));
#78860=CARTESIAN_POINT('Ctrl Pts',(6.74017131234314,-3.68442409526434,1.14791197408907E-15));
#78861=CARTESIAN_POINT('Ctrl Pts',(6.82181117015341,-3.49972844317531,1.40770594749215E-15));
#78862=CARTESIAN_POINT('Ctrl Pts',(6.89596686685091,-3.31234655293863,-1.88737914186277E-15));
#78863=CARTESIAN_POINT('Ctrl Pts',(6.96963536814041,-3.1261957427205,-5.16081585629826E-15));
#78864=CARTESIAN_POINT('Ctrl Pts',(7.03591792826469,-2.93739321795531,8.91671270961761E-15));
#78865=CARTESIAN_POINT('Ctrl Pts',(7.09456670151815,-2.74633316537145,6.66133814775094E-16));
#78866=CARTESIAN_POINT('Ctrl Pts',(7.13773030830017,-2.60571912480418,-5.40602632405713E-15));
#78867=CARTESIAN_POINT('Ctrl Pts',(7.17675810666365,-2.46388192110481,-5.8964836676042E-15));
#78868=CARTESIAN_POINT('Ctrl Pts',(7.21153340893003,-2.32097605948004,-5.38458166943201E-15));
#78869=CARTESIAN_POINT('Ctrl Pts',(7.25901043149182,-2.12587366282507,-3.21840629948907E-15));
#78870=CARTESIAN_POINT('Ctrl Pts',(7.29856300119499,-1.928778789233,-3.33446677566107E-15));
#78871=CARTESIAN_POINT('Ctrl Pts',(7.33014868626891,-1.73017913744427,-1.66533453693773E-16));
#78872=CARTESIAN_POINT('Ctrl Pts',(7.35985712442043,-1.54338295245514,2.81311859258955E-15));
#78873=CARTESIAN_POINT('Ctrl Pts',(7.38251706409064,-1.35525506107842,-1.0991374320194E-14));
#78874=CARTESIAN_POINT('Ctrl Pts',(7.39805220869348,-1.16621087705598,-8.82627304576999E-15));
#78875=CARTESIAN_POINT('Ctrl Pts',(7.40002531232882,-1.14220055875708,-9.18622245425996E-15));
#78876=CARTESIAN_POINT('Ctrl Pts',(7.40188343167553,-1.11817547822278,-1.11028146407842E-14));
#78877=CARTESIAN_POINT('Ctrl Pts',(7.40362636499328,-1.09413650426559,-1.23789867245705E-14));
#78878=CARTESIAN_POINT('Ctrl Pts',(7.40526549208637,-1.07152925182423,-8.27837043642381E-15));
#78879=CARTESIAN_POINT('Ctrl Pts',(7.4068020798626,-1.04891882611431,9.35859446300662E-16));
#78880=CARTESIAN_POINT('Ctrl Pts',(7.40823612148754,-1.02630740886741,-4.9960036108132E-16));
#78881=CARTESIAN_POINT('Ctrl Pts',(7.42081956607134,-0.827896490427196,
-1.45086831496663E-15));
#78882=CARTESIAN_POINT('Ctrl Pts',(7.42551437130127,-0.629371956630587,
1.87479693411711E-15));
#78883=CARTESIAN_POINT('Ctrl Pts',(7.42235848357616,-0.431206060649004,
3.19189119579733E-15));
#78884=CARTESIAN_POINT('Ctrl Pts',(7.41922110448639,-0.234202367072023,
4.50126096931357E-15));
#78885=CARTESIAN_POINT('Ctrl Pts',(7.40832471147218,-0.0375524031725907,
-2.23129519337553E-15));
#78886=CARTESIAN_POINT('Ctrl Pts',(7.38965476442135,0.158275945628522,-1.30451205393456E-15));
#78887=CARTESIAN_POINT('Ctrl Pts',(7.37081960531058,0.355837197303689,-3.69527726178446E-16));
#78888=CARTESIAN_POINT('Ctrl Pts',(7.34407270537559,0.552562969772611,-9.04532103063896E-15));
#78889=CARTESIAN_POINT('Ctrl Pts',(7.30934707767143,0.747957904919255,-1.04916075827077E-14));
#78890=CARTESIAN_POINT('Ctrl Pts',(7.27462144996726,0.943352840065898,-1.19378941347765E-14));
#78891=CARTESIAN_POINT('Ctrl Pts',(7.231917026481,1.13741766010537,-9.36028213032184E-15));
#78892=CARTESIAN_POINT('Ctrl Pts',(7.18111561966283,1.32963115094122,-1.04638520070921E-14));
#78893=CARTESIAN_POINT('Ctrl Pts',(7.17837256944882,1.34000982527717,-1.04344473399599E-14));
#78894=CARTESIAN_POINT('Ctrl Pts',(7.17560590005785,1.35038309419168,-8.87834579902764E-15));
#78895=CARTESIAN_POINT('Ctrl Pts',(7.17281558869492,1.36075087284441,-9.57567358739198E-15));
#78896=CARTESIAN_POINT('Ctrl Pts',(7.14346945585713,1.46979039209583,-1.09940822433459E-14));
#78897=CARTESIAN_POINT('Ctrl Pts',(7.11150861106633,1.57822295528145,-1.49401620285407E-15));
#78898=CARTESIAN_POINT('Ctrl Pts',(7.07696325132472,1.68595868374967,-1.19626530903361E-14));
#78899=CARTESIAN_POINT('Ctrl Pts',(7.06510387588707,1.72294421412221,-9.56354954911704E-15));
#78900=CARTESIAN_POINT('Ctrl Pts',(7.05293843640282,1.7598514332514,-1.40814083866707E-14));
#78901=CARTESIAN_POINT('Ctrl Pts',(7.04047968047903,1.796643391524,-1.33226762955019E-14));
#78902=CARTESIAN_POINT('Ctrl Pts',(6.97810874276675,1.98083103849048,-9.52431694982914E-15));
#78903=CARTESIAN_POINT('Ctrl Pts',(6.90833674176368,2.16230548123818,-2.00936910819825E-14));
#78904=CARTESIAN_POINT('Ctrl Pts',(6.83140645991705,2.3406495722722,-1.18377530000657E-14));
#78905=CARTESIAN_POINT('Ctrl Pts',(6.7547604043449,2.5183347540269,-3.61231726997968E-15));
#78906=CARTESIAN_POINT('Ctrl Pts',(6.67100842573644,2.69291325589164,-1.08516979078709E-14));
#78907=CARTESIAN_POINT('Ctrl Pts',(6.58034816210955,2.86394370118305,-8.18789480661053E-15));
#78908=CARTESIAN_POINT('Ctrl Pts',(6.5107253472596,2.99528703231687,-6.1422194170154E-15));
#78909=CARTESIAN_POINT('Ctrl Pts',(6.43702745650996,3.12453738507979,1.75858176966081E-14));
#78910=CARTESIAN_POINT('Ctrl Pts',(6.35932929176472,3.25148000052063,3.38618022510673E-15));
#78911=CARTESIAN_POINT('Ctrl Pts',(6.34415551430166,3.27627079195817,7.2328019561982E-15));
#78912=CARTESIAN_POINT('Ctrl Pts',(6.32882961100114,3.30097264814734,1.79741789374078E-15));
#78913=CARTESIAN_POINT('Ctrl Pts',(6.31335914601642,3.3255730433318,4.9960036108132E-16));
#78914=CARTESIAN_POINT('Ctrl Pts',(6.21150098685578,3.48754302746538,5.53132638240168E-15));
#78915=CARTESIAN_POINT('Ctrl Pts',(6.10330153910545,3.64524546448351,6.66685612455958E-15));
#78916=CARTESIAN_POINT('Ctrl Pts',(5.98896545356102,3.79825919093505,4.9960036108132E-15));
#78917=CARTESIAN_POINT('Ctrl Pts',(5.87621798675758,3.94914690028266,1.33293757130128E-14));
#78918=CARTESIAN_POINT('Ctrl Pts',(5.75750276055192,4.09547574709246,-2.11923734512429E-15));
#78919=CARTESIAN_POINT('Ctrl Pts',(5.63298215922921,4.23680466115335,-8.91647866652079E-16));
#78920=CARTESIAN_POINT('Ctrl Pts',(5.56848507749013,4.31000782934764,-2.55801764930648E-16));
#78921=CARTESIAN_POINT('Ctrl Pts',(5.50242998150509,4.38186893166116,5.78872423977802E-15));
#78922=CARTESIAN_POINT('Ctrl Pts',(5.43483639892989,4.4523220498536,6.67695065903473E-15));
#78923=CARTESIAN_POINT('Ctrl Pts',(5.39406123916706,4.49482219617873,6.59768912781167E-15));
#78924=CARTESIAN_POINT('Ctrl Pts',(5.35272618362371,4.53680991131998,5.15696403806271E-15));
#78925=CARTESIAN_POINT('Ctrl Pts',(5.31084235969185,4.57827599247481,6.81887272341308E-15));
#78926=CARTESIAN_POINT('Ctrl Pts',(5.31037376991264,4.57794244025893,20.));
#78927=CARTESIAN_POINT('Ctrl Pts',(5.44258499059786,4.44692576935788,20.));
#78928=CARTESIAN_POINT('Ctrl Pts',(5.56920635744265,4.3107893129539,20.));
#78929=CARTESIAN_POINT('Ctrl Pts',(5.69011135105436,4.17000439600832,20.));
#78930=CARTESIAN_POINT('Ctrl Pts',(5.81400769402978,4.02573627411689,20.));
#78931=CARTESIAN_POINT('Ctrl Pts',(5.9319017845614,3.87658649463656,20.));
#78932=CARTESIAN_POINT('Ctrl Pts',(6.04363170607624,3.7230137251186,20.));
#78933=CARTESIAN_POINT('Ctrl Pts',(6.1562476207376,3.56822315808105,20.));
#78934=CARTESIAN_POINT('Ctrl Pts',(6.26260167109238,3.40893866919477,20.));
#78935=CARTESIAN_POINT('Ctrl Pts',(6.36249517847558,3.24558783962327,20.));
#78936=CARTESIAN_POINT('Ctrl Pts',(6.46242012910578,3.08218559249104,20.));
#78937=CARTESIAN_POINT('Ctrl Pts',(6.55588089924594,2.91471387316095,20.));
#78938=CARTESIAN_POINT('Ctrl Pts',(6.6426392681944,2.74356691388431,20.));
#78939=CARTESIAN_POINT('Ctrl Pts',(6.70659897553043,2.61739453928274,20.));
#78940=CARTESIAN_POINT('Ctrl Pts',(6.76691522639903,2.48922397464942,20.));
#78941=CARTESIAN_POINT('Ctrl Pts',(6.82347677867138,2.35920420123498,20.));
#78942=CARTESIAN_POINT('Ctrl Pts',(6.83289078394379,2.33756393884352,20.));
#78943=CARTESIAN_POINT('Ctrl Pts',(6.84220167879346,2.31587022651507,20.));
#78944=CARTESIAN_POINT('Ctrl Pts',(6.85140588189888,2.29413090399489,20.));
#78945=CARTESIAN_POINT('Ctrl Pts',(6.92787028024333,2.11353034598004,20.));
#78946=CARTESIAN_POINT('Ctrl Pts',(6.99681396504024,1.93016810899366,20.));
#78947=CARTESIAN_POINT('Ctrl Pts',(7.05806564428657,1.74450976178054,20.));
#78948=CARTESIAN_POINT('Ctrl Pts',(7.08071894120841,1.67584595178894,20.));
#78949=CARTESIAN_POINT('Ctrl Pts',(7.10231976439282,1.60686769755636,20.));
#78950=CARTESIAN_POINT('Ctrl Pts',(7.12285814961541,1.53759730827682,20.));
#78951=CARTESIAN_POINT('Ctrl Pts',(7.17789437546803,1.35197508199331,20.));
#78952=CARTESIAN_POINT('Ctrl Pts',(7.22530500077645,1.16425705287924,20.));
#78953=CARTESIAN_POINT('Ctrl Pts',(7.2651668680032,0.974923813898792,20.));
#78954=CARTESIAN_POINT('Ctrl Pts',(7.30539082871382,0.78387072743286,20.));
#78955=CARTESIAN_POINT('Ctrl Pts',(7.33792842648121,0.591172314156727,20.));
#78956=CARTESIAN_POINT('Ctrl Pts',(7.36281005306225,0.397300196653284,20.));
#78957=CARTESIAN_POINT('Ctrl Pts',(7.38777115856543,0.202808797010905,20.));
#78958=CARTESIAN_POINT('Ctrl Pts',(7.40502742979251,0.00713548946427733,
20.));
#78959=CARTESIAN_POINT('Ctrl Pts',(7.41455881759031,-0.189255710324768,
20.));
#78960=CARTESIAN_POINT('Ctrl Pts',(7.41891526848925,-0.279018988980004,
20.));
#78961=CARTESIAN_POINT('Ctrl Pts',(7.421657226845,-0.368932343342073,20.));
#78962=CARTESIAN_POINT('Ctrl Pts',(7.42277915309801,-0.458951694386215,
20.));
#78963=CARTESIAN_POINT('Ctrl Pts',(7.42308605705979,-0.483576570930439,
20.));
#78964=CARTESIAN_POINT('Ctrl Pts',(7.42327160494634,-0.508201841411565,
20.));
#78965=CARTESIAN_POINT('Ctrl Pts',(7.42333592375777,-0.532819998670914,
20.));
#78966=CARTESIAN_POINT('Ctrl Pts',(7.42385714235562,-0.732317488160773,
20.));
#78967=CARTESIAN_POINT('Ctrl Pts',(7.41642303419139,-0.93148134030672,20.));
#78968=CARTESIAN_POINT('Ctrl Pts',(7.40111949060241,-1.12981386430432,20.));
#78969=CARTESIAN_POINT('Ctrl Pts',(7.38567034974055,-1.33003331563027,20.));
#78970=CARTESIAN_POINT('Ctrl Pts',(7.36220146956873,-1.52940623904774,20.));
#78971=CARTESIAN_POINT('Ctrl Pts',(7.33075071423941,-1.72743673897839,20.));
#78972=CARTESIAN_POINT('Ctrl Pts',(7.30904615534814,-1.86410005923912,20.));
#78973=CARTESIAN_POINT('Ctrl Pts',(7.28353913344292,-2.00012438495812,20.));
#78974=CARTESIAN_POINT('Ctrl Pts',(7.25422772630418,-2.13534847915567,20.));
#78975=CARTESIAN_POINT('Ctrl Pts',(7.21189212614094,-2.33065787379803,20.));
#78976=CARTESIAN_POINT('Ctrl Pts',(7.16162247429041,-2.52429848791992,20.));
#78977=CARTESIAN_POINT('Ctrl Pts',(7.10366596787394,-2.71587264560239,20.));
#78978=CARTESIAN_POINT('Ctrl Pts',(7.0459594755488,-2.90662038634025,20.));
#78979=CARTESIAN_POINT('Ctrl Pts',(6.98063203506653,-3.09532008764642,20.));
#78980=CARTESIAN_POINT('Ctrl Pts',(6.90787782849201,-3.28156683212074,20.));
#78981=CARTESIAN_POINT('Ctrl Pts',(6.89581151404611,-3.31245592966111,20.));
#78982=CARTESIAN_POINT('Ctrl Pts',(6.88353870682705,-3.34328252123178,20.));
#78983=CARTESIAN_POINT('Ctrl Pts',(6.87107234116059,-3.37401523348661,20.));
#78984=CARTESIAN_POINT('Ctrl Pts',(6.79527663912565,-3.56087061404549,20.));
#78985=CARTESIAN_POINT('Ctrl Pts',(6.71226278618979,-3.74443472774651,20.));
#78986=CARTESIAN_POINT('Ctrl Pts',(6.62235335551551,-3.92432447229519,20.));
#78987=CARTESIAN_POINT('Ctrl Pts',(6.53088269512199,-4.10733790713164,20.));
#78988=CARTESIAN_POINT('Ctrl Pts',(6.4322747831017,-4.28654890171632,20.));
#78989=CARTESIAN_POINT('Ctrl Pts',(6.32681586246644,-4.46154936748218,20.));
#78990=CARTESIAN_POINT('Ctrl Pts',(6.22105095057789,-4.63705760074199,20.));
#78991=CARTESIAN_POINT('Ctrl Pts',(6.10839496565391,-4.80833150317585,20.));
#78992=CARTESIAN_POINT('Ctrl Pts',(5.98908635398953,-4.9749448495409,20.));
#78993=CARTESIAN_POINT('Ctrl Pts',(5.87055983530591,-5.14046601046456,20.));
#78994=CARTESIAN_POINT('Ctrl Pts',(5.74546730794022,-5.30138815195256,20.));
#78995=CARTESIAN_POINT('Ctrl Pts',(5.61399733100531,-5.45726932553109,20.));
#78996=CARTESIAN_POINT('Ctrl Pts',(5.59056995179115,-5.48504667402474,20.));
#78997=CARTESIAN_POINT('Ctrl Pts',(5.56693995540417,-5.51266387690693,20.));
#78998=CARTESIAN_POINT('Ctrl Pts',(5.54310826839702,-5.54011832860014,20.));
#78999=CARTESIAN_POINT('Ctrl Pts',(5.48873752541245,-5.60275421905749,20.));
#79000=CARTESIAN_POINT('Ctrl Pts',(5.4333170502013,-5.66454305419315,20.));
#79001=CARTESIAN_POINT('Ctrl Pts',(5.37687176772693,-5.72546775434948,20.));
#79002=CARTESIAN_POINT('Ctrl Pts',(5.34692970249771,-5.75778597947273,20.));
#79003=CARTESIAN_POINT('Ctrl Pts',(5.31669957407756,-5.78986069271576,20.));
#79004=CARTESIAN_POINT('Ctrl Pts',(5.28618389754254,-5.82169036550656,20.));
#79005=CARTESIAN_POINT('Ctrl Pts',(5.26222541995964,-5.8466804882441,20.));
#79006=CARTESIAN_POINT('Ctrl Pts',(5.23809317649021,-5.87151706999867,20.));
#79007=CARTESIAN_POINT('Ctrl Pts',(5.21380409728959,-5.8961838900846,20.));
#79008=CARTESIAN_POINT('Ctrl Pts',(5.06917294826217,-6.04306432562574,20.));
#79009=CARTESIAN_POINT('Ctrl Pts',(4.91885274484368,-6.18406632260094,20.));
#79010=CARTESIAN_POINT('Ctrl Pts',(4.76330525902998,-6.31898881110124,20.));
#79011=CARTESIAN_POINT('Ctrl Pts',(4.60608464123105,-6.4553625807319,20.));
#79012=CARTESIAN_POINT('Ctrl Pts',(4.44352323643732,-6.58552582901827,20.));
#79013=CARTESIAN_POINT('Ctrl Pts',(4.27605405044702,-6.70924078257424,20.));
#79014=CARTESIAN_POINT('Ctrl Pts',(4.18911861719913,-6.77346282451606,20.));
#79015=CARTESIAN_POINT('Ctrl Pts',(4.10085996926207,-6.83594665435447,20.));
#79016=CARTESIAN_POINT('Ctrl Pts',(4.01133472131358,-6.89665519792269,20.));
#79017=CARTESIAN_POINT('Ctrl Pts',(3.96858583980601,-6.92564391780859,20.));
#79018=CARTESIAN_POINT('Ctrl Pts',(3.92554812122795,-6.95422780963465,20.));
#79019=CARTESIAN_POINT('Ctrl Pts',(3.88222753925519,-6.98240260462403,20.));
#79020=CARTESIAN_POINT('Ctrl Pts',(3.83688314264079,-7.01189364607243,20.));
#79021=CARTESIAN_POINT('Ctrl Pts',(3.79122247495776,-7.04094023216963,20.));
#79022=CARTESIAN_POINT('Ctrl Pts',(3.74529296566859,-7.06951255916912,20.));
#79023=CARTESIAN_POINT('Ctrl Pts',(3.66342765985698,-7.12044021600156,20.));
#79024=CARTESIAN_POINT('Ctrl Pts',(3.5806901914544,-7.16987375606264,20.));
#79025=CARTESIAN_POINT('Ctrl Pts',(3.49712247540394,-7.21779315037648,20.));
#79026=CARTESIAN_POINT('Ctrl Pts',(3.30484647767293,-7.32804804051606,20.));
#79027=CARTESIAN_POINT('Ctrl Pts',(3.10818162093266,-7.43028820260646,20.));
#79028=CARTESIAN_POINT('Ctrl Pts',(2.90763049540401,-7.524222843759,20.));
#79029=CARTESIAN_POINT('Ctrl Pts',(2.70707936987535,-7.61815748491155,20.));
#79030=CARTESIAN_POINT('Ctrl Pts',(2.50264126591493,-7.70378717616298,20.));
#79031=CARTESIAN_POINT('Ctrl Pts',(2.2947819056922,-7.78077036713514,20.));
#79032=CARTESIAN_POINT('Ctrl Pts',(2.23095378491342,-7.80440987226034,20.));
#79033=CARTESIAN_POINT('Ctrl Pts',(2.16680283827967,-7.82723366713653,20.));
#79034=CARTESIAN_POINT('Ctrl Pts',(2.10234503241322,-7.84924105753589,20.));
#79035=CARTESIAN_POINT('Ctrl Pts',(5.31040305176835,4.57790847333905,-0.000178101097112471));
#79036=CARTESIAN_POINT('Ctrl Pts',(5.30882975752663,4.57973350470244,-0.00011873406474153));
#79037=CARTESIAN_POINT('Ctrl Pts',(5.30725552246937,4.58155772502242,-5.93670323709406E-5));
#79038=CARTESIAN_POINT('Ctrl Pts',(5.30568034743329,4.58338113332943,0.));
#79039=CARTESIAN_POINT('Ctrl Pts',(-2.10222011176618,-7.84913218468459,
19.999697384906));
#79040=CARTESIAN_POINT('Ctrl Pts',(-3.40743872906296,-7.49955763771916,
19.9467661843935));
#79041=CARTESIAN_POINT('Ctrl Pts',(-5.83879819321471,-6.13705586876475,
19.8409037833685));
#79042=CARTESIAN_POINT('Ctrl Pts',(-8.063328137307,-2.59492553977183,19.6821101818309));
#79043=CARTESIAN_POINT('Ctrl Pts',(-8.32211031922223,1.57870274228667,19.5233165802935));
#79044=CARTESIAN_POINT('Ctrl Pts',(-6.55256548103476,5.3680183485327,19.3645229787559));
#79045=CARTESIAN_POINT('Ctrl Pts',(-3.18576426764331,7.8486441896436,19.2057293772185));
#79046=CARTESIAN_POINT('Ctrl Pts',(0.957516033830517,8.41630867132718,19.0469357756809));
#79047=CARTESIAN_POINT('Ctrl Pts',(4.8674260860221,6.93245445843938,18.8881421741434));
#79048=CARTESIAN_POINT('Ctrl Pts',(7.59090189466519,3.75886426572798,18.7293485726058));
#79049=CARTESIAN_POINT('Ctrl Pts',(8.46411978115432,-0.330956437631908,
18.5705549710684));
#79050=CARTESIAN_POINT('Ctrl Pts',(7.27422648106118,-4.34009886765195,18.4117613695308));
#79051=CARTESIAN_POINT('Ctrl Pts',(4.31125990388258,-7.2913572173132,18.2529677679934));
#79052=CARTESIAN_POINT('Ctrl Pts',(0.297433621833983,-8.46536305708804,
18.0941741664558));
#79053=CARTESIAN_POINT('Ctrl Pts',(-3.78889099106759,-7.57595866543456,
17.9353805649183));
#79054=CARTESIAN_POINT('Ctrl Pts',(-6.95168297254158,-4.8399324863166,17.7765869633808));
#79055=CARTESIAN_POINT('Ctrl Pts',(-8.42001929378617,-0.924185001110069,
17.6177933618432));
#79056=CARTESIAN_POINT('Ctrl Pts',(-7.83599675007498,3.21683044313197,17.4589997603057));
#79057=CARTESIAN_POINT('Ctrl Pts',(-5.34196931903587,6.57375133412712,17.3002061587682));
#79058=CARTESIAN_POINT('Ctrl Pts',(-1.54585006801036,8.32833660506733,17.1414125572307));
#79059=CARTESIAN_POINT('Ctrl Pts',(2.62706632719926,8.05291037069421,16.9826189556932));
#79060=CARTESIAN_POINT('Ctrl Pts',(6.15964178765682,5.81460712479525,16.8238253541557));
#79061=CARTESIAN_POINT('Ctrl Pts',(8.19081977136801,2.15900774267334,16.6650317526181));
#79062=CARTESIAN_POINT('Ctrl Pts',(8.22550565692099,-2.02284444389487,16.5062381510806));
#79063=CARTESIAN_POINT('Ctrl Pts',(6.25524484665678,-5.71163329267625,16.3474445495431));
#79064=CARTESIAN_POINT('Ctrl Pts',(2.76028354811421,-8.00822562692782,16.1886509480056));
#79065=CARTESIAN_POINT('Ctrl Pts',(-1.40749005041534,-8.35283273613254,
16.0298573464681));
#79066=CARTESIAN_POINT('Ctrl Pts',(-5.23219142410912,-6.66145748770267,
15.8710637449305));
#79067=CARTESIAN_POINT('Ctrl Pts',(-7.7815590556908,-3.34636842293283,15.712270143393));
#79068=CARTESIAN_POINT('Ctrl Pts',(-8.43419087903681,0.784389683258458,
15.5534765418555));
#79069=CARTESIAN_POINT('Ctrl Pts',(-7.03100949843993,4.72395474068076,15.394682940318));
#79070=CARTESIAN_POINT('Ctrl Pts',(-3.91403691117488,7.51206749285283,15.2358893387805));
#79071=CARTESIAN_POINT('Ctrl Pts',(0.156972509984872,8.46913233987333,15.077095737243));
#79072=CARTESIAN_POINT('Ctrl Pts',(4.18972026937783,7.36186708814822,14.9183021357054));
#79073=CARTESIAN_POINT('Ctrl Pts',(7.20123405694,4.46016490909898,14.7595085341679));
#79074=CARTESIAN_POINT('Ctrl Pts',(8.45746482195596,0.471308544976929,14.6007149326304));
#79075=CARTESIAN_POINT('Ctrl Pts',(7.65220941691035,-3.63242811338918,14.4419213310929));
#79076=CARTESIAN_POINT('Ctrl Pts',(4.98174685872065,-6.85076938707017,14.2831277295554));
#79077=CARTESIAN_POINT('Ctrl Pts',(1.09699580294953,-8.39925253623812,14.1243341280179));
#79078=CARTESIAN_POINT('Ctrl Pts',(-3.05514527146234,-7.90043861627013,
13.9655405264804));
#79079=CARTESIAN_POINT('Ctrl Pts',(-6.46260222867888,-5.47591228865712,
13.8067469249428));
#79080=CARTESIAN_POINT('Ctrl Pts',(-8.2948158479101,-1.71664585994049,13.6479533234053));
#79081=CARTESIAN_POINT('Ctrl Pts',(-8.10518858294586,2.46104875897965,13.4891597218678));
#79082=CARTESIAN_POINT('Ctrl Pts',(-5.93994161145822,6.03886881888142,13.3303661203303));
#79083=CARTESIAN_POINT('Ctrl Pts',(-2.32684853705731,8.14472951329788,13.1715725187928));
#79084=CARTESIAN_POINT('Ctrl Pts',(1.85340812358983,8.2653324970386,13.0127789172552));
#79085=CARTESIAN_POINT('Ctrl Pts',(5.58190112991571,6.37128109056859,12.8539853157177));
#79086=CARTESIAN_POINT('Ctrl Pts',(7.94981951675275,2.92424564806863,12.6951917141802));
#79087=CARTESIAN_POINT('Ctrl Pts',(8.3799890233666,-1.23556745159722,12.5363981126427));
#79088=CARTESIAN_POINT('Ctrl Pts',(6.76755689454807,-5.09421403537837,12.3776045111052));
#79089=CARTESIAN_POINT('Ctrl Pts',(3.50554948082876,-7.71115852493337,12.2188109095677));
#79090=CARTESIAN_POINT('Ctrl Pts',(-0.610926964134399,-8.44852716180073,
12.0600173080301));
#79091=CARTESIAN_POINT('Ctrl Pts',(-4.57849146988245,-7.12658816120343,
11.9012237064926));
#79092=CARTESIAN_POINT('Ctrl Pts',(-7.43005998349757,-4.06756089085575,
11.7424301049551));
#79093=CARTESIAN_POINT('Ctrl Pts',(-8.47056971990735,-0.0170756955972321,
11.5836365034176));
#79094=CARTESIAN_POINT('Ctrl Pts',(-7.44639899973391,4.03757165830562,11.4248429018801));
#79095=CARTESIAN_POINT('Ctrl Pts',(-4.60718690748627,7.10807088869254,11.2660493003426));
#79096=CARTESIAN_POINT('Ctrl Pts',(-0.644984381034744,8.44599538878707,
11.107255698805));
#79097=CARTESIAN_POINT('Ctrl Pts',(3.47443149591835,7.72522936483841,10.9484620972675));
#79098=CARTESIAN_POINT('Ctrl Pts',(6.74696327362364,5.1214577557142,10.78966849573));
#79099=CARTESIAN_POINT('Ctrl Pts',(8.37493941068567,1.26934346279288,10.6308748941925));
#79100=CARTESIAN_POINT('Ctrl Pts',(7.96154474293954,-2.89217016535385,10.472081292655));
#79101=CARTESIAN_POINT('Ctrl Pts',(5.60754320003511,-6.34872445605661,10.3132876911175));
#79102=CARTESIAN_POINT('Ctrl Pts',(1.88671684635692,-8.2577928347025,10.1544940895799));
#79103=CARTESIAN_POINT('Ctrl Pts',(-2.29399208058248,-8.15404459721776,
9.99570048804245));
#79104=CARTESIAN_POINT('Ctrl Pts',(-5.91554610142342,-6.06276812034943,
9.83690688650493));
#79105=CARTESIAN_POINT('Ctrl Pts',(-8.09520036469299,-2.49370688226696,
9.67811328496741));
#79106=CARTESIAN_POINT('Ctrl Pts',(-8.30166952497879,1.68318925175681,9.5193196834299));
#79107=CARTESIAN_POINT('Ctrl Pts',(-6.48462723420443,5.4498121612222,9.36052608189237));
#79108=CARTESIAN_POINT('Ctrl Pts',(-3.08697306472453,7.88805681120873,9.20173248035486));
#79109=CARTESIAN_POINT('Ctrl Pts',(1.06312316798005,8.40360708796499,9.04293887881735));
#79110=CARTESIAN_POINT('Ctrl Pts',(4.95408575319091,6.87079888435267,8.88414527727982));
#79111=CARTESIAN_POINT('Ctrl Pts',(7.63750216700183,3.66325041571465,8.72535167574231));
#79112=CARTESIAN_POINT('Ctrl Pts',(8.45929628352375,-0.437206297704228,
8.56655807420478));
#79113=CARTESIAN_POINT('Ctrl Pts',(7.2191578157485,-4.43109505545849,8.40776447266728));
#79114=CARTESIAN_POINT('Ctrl Pts',(4.21936745346892,-7.34491533319468,8.24897087112975));
#79115=CARTESIAN_POINT('Ctrl Pts',(0.191116691430598,-8.46843063202667,
8.09017726959224));
#79116=CARTESIAN_POINT('Ctrl Pts',(-3.88371829230374,-7.52778687166532,
7.93138366805473));
#79117=CARTESIAN_POINT('Ctrl Pts',(-7.01190653064279,-4.75226364638159,
7.7725900665172));
#79118=CARTESIAN_POINT('Ctrl Pts',(-8.43095986354782,-0.818387889962332,
7.61379646497969));
#79119=CARTESIAN_POINT('Ctrl Pts',(-7.79498754456611,3.31496789415078,7.45500286344217));
#79120=CARTESIAN_POINT('Ctrl Pts',(-5.25900625632336,6.64030843825366,7.29620926190465));
#79121=CARTESIAN_POINT('Ctrl Pts',(-1.44115517684792,8.34709019451903,7.13741566036713));
#79122=CARTESIAN_POINT('Ctrl Pts',(2.72797391897493,8.01928932366103,6.97862205882962));
#79123=CARTESIAN_POINT('Ctrl Pts',(6.23216610703123,5.73680647865712,6.8198284572921));
#79124=CARTESIAN_POINT('Ctrl Pts',(8.21728319283949,2.05599121784817,6.66103485575458));
#79125=CARTESIAN_POINT('Ctrl Pts',(8.19945778770858,-2.12596682635838,6.50224125421707));
#79126=CARTESIAN_POINT('Ctrl Pts',(6.18303479013073,-5.7897257053529,6.34344765267954));
#79127=CARTESIAN_POINT('Ctrl Pts',(2.65951232750101,-8.04225323768542,6.18465405114204));
#79128=CARTESIAN_POINT('Ctrl Pts',(-1.51225969899553,-8.33450139852319,
6.02586044960451));
#79129=CARTESIAN_POINT('Ctrl Pts',(-5.3154221574182,-6.59523542018167,5.867066848067));
#79130=CARTESIAN_POINT('Ctrl Pts',(-7.82296358799924,-3.24839709087868,
5.70827324652947));
#79131=CARTESIAN_POINT('Ctrl Pts',(-8.42367695780134,0.890230009490827,
5.54947964499197));
#79132=CARTESIAN_POINT('Ctrl Pts',(-6.97113986601195,4.81186574289953,5.39068604345444));
#79133=CARTESIAN_POINT('Ctrl Pts',(-3.81940464264517,7.56062108129564,5.23189244191693));
#79134=CARTESIAN_POINT('Ctrl Pts',(0.263301032793999,8.46649369723502,5.07309884037941));
#79135=CARTESIAN_POINT('Ctrl Pts',(4.28182773154276,7.30867937705459,4.9143052388419));
#79136=CARTESIAN_POINT('Ctrl Pts',(7.25666949195797,4.36939250281743,4.75551163730438));
#79137=CARTESIAN_POINT('Ctrl Pts',(8.46271597940375,0.365076993433917,4.59671803576686));
#79138=CARTESIAN_POINT('Ctrl Pts',(7.60599634012455,-3.7282251317762,4.43792443422934));
#79139=CARTESIAN_POINT('Ctrl Pts',(4.89533387107377,-6.91278158557734,4.27913083269182));
#79140=CARTESIAN_POINT('Ctrl Pts',(0.991445856839866,-8.41236459458163,
4.12033723115431));
#79141=CARTESIAN_POINT('Ctrl Pts',(-3.15410463726016,-7.8614545025947,3.96154362961679));
#79142=CARTESIAN_POINT('Ctrl Pts',(-6.53084991306519,-5.39433428443648,
3.80275002807927));
#79143=CARTESIAN_POINT('Ctrl Pts',(-8.31571664631593,-1.61235840227592,
3.64395642654176));
#79144=CARTESIAN_POINT('Ctrl Pts',(-8.07364797734855,2.56262585970849,3.48516282500424));
#79145=CARTESIAN_POINT('Ctrl Pts',(-5.86364754662715,6.11297639523982,3.32636922346672));
#79146=CARTESIAN_POINT('Ctrl Pts',(-2.22439750288786,8.17330402633597,3.16757562192921));
#79147=CARTESIAN_POINT('Ctrl Pts',(1.957043940362,8.24140898009109,3.00878202039168));
#79148=CARTESIAN_POINT('Ctrl Pts',(5.66146075499942,6.3006908411568,2.84998841885417));
#79149=CARTESIAN_POINT('Ctrl Pts',(7.98591048759216,2.8241948665278,2.69119481731665));
#79150=CARTESIAN_POINT('Ctrl Pts',(8.36381425563696,-1.34069163686942,2.53240121577913));
#79151=CARTESIAN_POINT('Ctrl Pts',(6.7030589465472,-5.17878785866461,2.37360761424162));
#79152=CARTESIAN_POINT('Ctrl Pts',(3.40844957090335,-7.75456733562105,2.2148140127041));
#79153=CARTESIAN_POINT('Ctrl Pts',(-0.716960978086715,-8.44019014977505,
2.05602041116658));
#79154=CARTESIAN_POINT('Ctrl Pts',(-4.66761404808927,-7.06853749124428,
1.89722680962907));
#79155=CARTESIAN_POINT('Ctrl Pts',(-7.480547738494,-3.97394619441689,1.73843320809155));
#79156=CARTESIAN_POINT('Ctrl Pts',(-8.47011634489816,0.0892845267466103,
1.57963960655403));
#79157=CARTESIAN_POINT('Ctrl Pts',(-7.39511508466361,4.13075265867455,1.42084600501651));
#79158=CARTESIAN_POINT('Ctrl Pts',(-4.51757262101829,7.16535945096504,1.262052403479));
#79159=CARTESIAN_POINT('Ctrl Pts',(-0.53888329681407,8.45342870211286,1.10325880194148));
#79160=CARTESIAN_POINT('Ctrl Pts',(3.57115811491559,7.68099334702474,0.944465200403969));
#79161=CARTESIAN_POINT('Ctrl Pts',(6.81073734528766,5.03633921085957,0.785671598866447));
#79162=CARTESIAN_POINT('Ctrl Pts',(8.39021853594661,1.16408120921888,0.626877997328932));
#79163=CARTESIAN_POINT('Ctrl Pts',(7.92460000763248,-2.9919017765053,0.468084395791413));
#79164=CARTESIAN_POINT('Ctrl Pts',(5.52738896171523,-6.41864938067256,0.309290794253898));
#79165=CARTESIAN_POINT('Ctrl Pts',(1.78287247840694,-8.28080161037312,0.150497192716378));
#79166=CARTESIAN_POINT('Ctrl Pts',(-2.39617932800353,-8.12465753133514,
-0.00829640882114185));
#79167=CARTESIAN_POINT('Ctrl Pts',(-5.99123816337043,-5.9878951045908,-0.167090010358655));
#79168=CARTESIAN_POINT('Ctrl Pts',(-8.1258084234525,-2.39209880067588,-0.325883611896176));
#79169=CARTESIAN_POINT('Ctrl Pts',(-8.28003535986636,1.78802420893543,-0.484686260456206));
#79170=CARTESIAN_POINT('Ctrl Pts',(-7.03657972594842,4.28266391599147,-0.590557708503744));
#79171=CARTESIAN_POINT('Ctrl Pts',(-6.15407036887642,5.3061872692741,-0.64349795603877));
#79172=CARTESIAN_POINT('Ctrl Pts',(-2.00604353560581,-7.49003436465715,
20.2143297668606));
#79173=CARTESIAN_POINT('Ctrl Pts',(-3.25154839740679,-7.15645285422094,
20.1613985663481));
#79174=CARTESIAN_POINT('Ctrl Pts',(-5.57167315907976,-5.85628554511544,
20.0555361653231));
#79175=CARTESIAN_POINT('Ctrl Pts',(-7.69443085183093,-2.47620768886292,
19.8967425637855));
#79176=CARTESIAN_POINT('Ctrl Pts',(-7.94137374817917,1.5064770872859,19.737948962248));
#79177=CARTESIAN_POINT('Ctrl Pts',(-6.25278559142888,5.12243149364616,19.5791553607105));
#79178=CARTESIAN_POINT('Ctrl Pts',(-3.04001554323474,7.48956869539067,19.420361759173));
#79179=CARTESIAN_POINT('Ctrl Pts',(0.913709672528465,8.03126252540434,19.2615681576355));
#79180=CARTESIAN_POINT('Ctrl Pts',(4.64474132858538,6.61529464702449,19.102774556098));
#79181=CARTESIAN_POINT('Ctrl Pts',(7.24361811114894,3.58689621475851,18.9439809545604));
#79182=CARTESIAN_POINT('Ctrl Pts',(8.07688627681936,-0.315815179658241,
18.7851873530229));
#79183=CARTESIAN_POINT('Ctrl Pts',(6.94143059862823,-4.14153933197253,18.6263937514854));
#79184=CARTESIAN_POINT('Ctrl Pts',(4.11401975087856,-6.95777760364743,18.4676001499479));
#79185=CARTESIAN_POINT('Ctrl Pts',(0.283826032779512,-8.07807267287554,
18.3088065484104));
#79186=CARTESIAN_POINT('Ctrl Pts',(-3.61554921732747,-7.22935853469858,
18.1500129468728));
#79187=CARTESIAN_POINT('Ctrl Pts',(-6.63364345655119,-4.61850556114549,
17.9912193453353));
#79188=CARTESIAN_POINT('Ctrl Pts',(-8.03480338687517,-0.881903534650851,
17.8324257437978));
#79189=CARTESIAN_POINT('Ctrl Pts',(-7.47749987621871,3.06966044110543,17.6736321422603));
#79190=CARTESIAN_POINT('Ctrl Pts',(-5.09757420732374,6.27300219168134,17.5148385407228));
#79191=CARTESIAN_POINT('Ctrl Pts',(-1.47512742295223,7.94731518142893,17.3560449391853));
#79192=CARTESIAN_POINT('Ctrl Pts',(2.5068780351731,7.68448969807065,17.1972513376478));
#79193=CARTESIAN_POINT('Ctrl Pts',(5.87783815815324,5.54858883211008,17.0384577361102));
#79194=CARTESIAN_POINT('Ctrl Pts',(7.81608974326692,2.06023313223562,16.8796641345727));
#79195=CARTESIAN_POINT('Ctrl Pts',(7.84918874945609,-1.93029930476795,16.7208705330352));
#79196=CARTESIAN_POINT('Ctrl Pts',(5.96906737692894,-5.45032605310672,16.5620769314977));
#79197=CARTESIAN_POINT('Ctrl Pts',(2.634000567848,-7.64184928146013,16.4032833299602));
#79198=CARTESIAN_POINT('Ctrl Pts',(-1.34309737656017,-7.97069061442744,
16.2444897284227));
#79199=CARTESIAN_POINT('Ctrl Pts',(-4.99281865140567,-6.35669578847852,
16.0856961268851));
#79200=CARTESIAN_POINT('Ctrl Pts',(-7.4255527065092,-3.19327205795779,15.9269025253476));
#79201=CARTESIAN_POINT('Ctrl Pts',(-8.04832662205982,0.748503852993082,
15.7681089238101));
#79202=CARTESIAN_POINT('Ctrl Pts',(-6.70934079366152,4.5078337977061,15.6093153222726));
#79203=CARTESIAN_POINT('Ctrl Pts',(-3.73496971122986,7.16839038344626,15.4505217207351));
#79204=CARTESIAN_POINT('Ctrl Pts',(0.149791017201536,8.08166951096257,15.2917281191975));
#79205=CARTESIAN_POINT('Ctrl Pts',(3.998040555002,7.02506164768895,15.13293451766));
#79206=CARTESIAN_POINT('Ctrl Pts',(6.87177757812056,4.25611235167798,14.9741409161225));
#79207=CARTESIAN_POINT('Ctrl Pts',(8.07053578202346,0.449746177688511,14.815347314585));
#79208=CARTESIAN_POINT('Ctrl Pts',(7.30212081407504,-3.46624451675291,14.6565537130475));
#79209=CARTESIAN_POINT('Ctrl Pts',(4.75383192560413,-6.53734666790537,14.49776011151));
#79210=CARTESIAN_POINT('Ctrl Pts',(1.04680824180907,-8.01498670854467,14.3389665099724));
#79211=CARTESIAN_POINT('Ctrl Pts',(-2.91537236650478,-7.53899352685007,
14.180172908435));
#79212=CARTESIAN_POINT('Ctrl Pts',(-6.16693815812707,-5.22538928569952,
14.0213793068974));
#79213=CARTESIAN_POINT('Ctrl Pts',(-7.91532799900807,-1.63810930691027,
13.8625857053599));
#79214=CARTESIAN_POINT('Ctrl Pts',(-7.73437618196141,2.34845577117709,13.7037921038224));
#79215=CARTESIAN_POINT('Ctrl Pts',(-5.66818926564769,5.76259055304671,13.5449985022848));
#79216=CARTESIAN_POINT('Ctrl Pts',(-2.22039520979373,7.77210811463608,13.3862049007473));
#79217=CARTESIAN_POINT('Ctrl Pts',(1.76861469660425,7.88719351152376,13.2274112992098));
#79218=CARTESIAN_POINT('Ctrl Pts',(5.32652913716566,6.07979496234801,13.0686176976723));
#79219=CARTESIAN_POINT('Ctrl Pts',(7.58611525099355,2.79046140125786,12.9098240961348));
#79220=CARTESIAN_POINT('Ctrl Pts',(7.99660450144244,-1.17904023713253,12.7510304945973));
#79221=CARTESIAN_POINT('Ctrl Pts',(6.45794114715554,-4.86115372860623,12.5922368930598));
#79222=CARTESIAN_POINT('Ctrl Pts',(3.34517058199709,-7.35837300023643,12.4334432915223));
#79223=CARTESIAN_POINT('Ctrl Pts',(-0.582977053767915,-8.06200701984604,
12.2746496899847));
#79224=CARTESIAN_POINT('Ctrl Pts',(-4.36902547196524,-6.80054673232866,
12.1158560884472));
#79225=CARTESIAN_POINT('Ctrl Pts',(-7.0901347178799,-3.8814699683987,11.9570624869097));
#79226=CARTESIAN_POINT('Ctrl Pts',(-8.08304113085587,-0.0162944824745385,
11.7982688853722));
#79227=CARTESIAN_POINT('Ctrl Pts',(-7.10572622407645,3.85285274332402,11.6394752838346));
#79228=CARTESIAN_POINT('Ctrl Pts',(-4.39640809321612,6.7828766250884,11.4806816822971));
#79229=CARTESIAN_POINT('Ctrl Pts',(-0.615476343747107,8.05959107545505,
11.3218880807596));
#79230=CARTESIAN_POINT('Ctrl Pts',(3.31547624498585,7.37180009917534,11.1630944792221));
#79231=CARTESIAN_POINT('Ctrl Pts',(6.43828968444762,4.88715104865834,11.0043008776846));
#79232=CARTESIAN_POINT('Ctrl Pts',(7.99178590855619,1.21127099571882,10.845507276147));
#79233=CARTESIAN_POINT('Ctrl Pts',(7.59730404804857,-2.75985337196954,10.6867136746096));
#79234=CARTESIAN_POINT('Ctrl Pts',(5.35099808250333,-6.05827029392982,10.527920073072));
#79235=CARTESIAN_POINT('Ctrl Pts',(1.80039954520892,-7.87999878876122,10.3691264715345));
#79236=CARTESIAN_POINT('Ctrl Pts',(-2.18904193629713,-7.78099703343982,
10.210332869997));
#79237=CARTESIAN_POINT('Ctrl Pts',(-5.64490985026715,-5.78539646140382,
10.0515392684595));
#79238=CARTESIAN_POINT('Ctrl Pts',(-7.72484492472234,-2.37961978523008,
9.89274566692192));
#79239=CARTESIAN_POINT('Ctrl Pts',(-7.92186812033116,1.60618333864722,9.7339520653844));
#79240=CARTESIAN_POINT('Ctrl Pts',(-6.18795551958646,5.20048323916983,9.57515846384689));
#79241=CARTESIAN_POINT('Ctrl Pts',(-2.94574403813367,7.52717818940584,9.41636486230936));
#79242=CARTESIAN_POINT('Ctrl Pts',(1.01448527998687,8.0191420395175,9.25757126077186));
#79243=CARTESIAN_POINT('Ctrl Pts',(4.72743631573194,6.55645981562959,9.09877765923432));
#79244=CARTESIAN_POINT('Ctrl Pts',(7.28808642089212,3.49565669865832,8.93998405769683));
#79245=CARTESIAN_POINT('Ctrl Pts',(8.07228345421928,-0.417204108326629,
8.78119045615929));
#79246=CARTESIAN_POINT('Ctrl Pts',(6.88888132491199,-4.22837244392516,8.6223968546218));
#79247=CARTESIAN_POINT('Ctrl Pts',(4.02633138033566,-7.00888543557329,8.46360325308425));
#79248=CARTESIAN_POINT('Ctrl Pts',(0.182373102247894,-8.0809999062519,8.30480965154676));
#79249=CARTESIAN_POINT('Ctrl Pts',(-3.70603816925928,-7.18339060063285,
8.14601605000923));
#79250=CARTESIAN_POINT('Ctrl Pts',(-6.69111178669606,-4.53484757088968,
7.98722244847172));
#79251=CARTESIAN_POINT('Ctrl Pts',(-8.04524342553875,-0.780946641642448,
7.8284288469342));
#79252=CARTESIAN_POINT('Ctrl Pts',(-7.43836684197983,3.16330810345782,7.66963524539667));
#79253=CARTESIAN_POINT('Ctrl Pts',(-5.01840670496898,6.33651430810264,7.51084164385916));
#79254=CARTESIAN_POINT('Ctrl Pts',(-1.37522232336164,7.96521079410926,7.35204804232165));
#79255=CARTESIAN_POINT('Ctrl Pts',(2.60316910433477,7.65240681403595,7.19325444078413));
#79256=CARTESIAN_POINT('Ctrl Pts',(5.94704448970765,5.47434756575656,7.03446083924661));
#79257=CARTESIAN_POINT('Ctrl Pts',(7.84134246312996,1.96192961371753,6.87566723770909));
#79258=CARTESIAN_POINT('Ctrl Pts',(7.82433257033507,-2.02870383793711,6.71687363617158));
#79259=CARTESIAN_POINT('Ctrl Pts',(5.90016093069667,-5.52484573767879,6.55808003463406));
#79260=CARTESIAN_POINT('Ctrl Pts',(2.53783963086772,-7.67432012892767,6.39928643309655));
#79261=CARTESIAN_POINT('Ctrl Pts',(-1.44307381341645,-7.95319793556645,
6.24049283155902));
#79262=CARTESIAN_POINT('Ctrl Pts',(-5.07224157842644,-6.29350338073708,
6.08169923002151));
#79263=CARTESIAN_POINT('Ctrl Pts',(-7.46506298134543,-3.09978291462693,
5.92290562848398));
#79264=CARTESIAN_POINT('Ctrl Pts',(-8.03829371275112,0.849501983995867,
5.76411202694648));
#79265=CARTESIAN_POINT('Ctrl Pts',(-6.65221019708932,4.59172287132047,5.60531842540895));
#79266=CARTESIAN_POINT('Ctrl Pts',(-3.64466686925759,7.21472264507814,5.44652482387144));
#79267=CARTESIAN_POINT('Ctrl Pts',(0.251255009786289,8.07915158623255,5.28773122233392));
#79268=CARTESIAN_POINT('Ctrl Pts',(4.08593410050795,6.97430727453083,5.1289376207964));
#79269=CARTESIAN_POINT('Ctrl Pts',(6.92467684182701,4.16949278324492,4.9701440192589));
#79270=CARTESIAN_POINT('Ctrl Pts',(8.07554669900292,0.348374719934165,4.81135041772136));
#79271=CARTESIAN_POINT('Ctrl Pts',(7.2580219856851,-3.55765882127316,4.65255681618386));
#79272=CARTESIAN_POINT('Ctrl Pts',(4.67137233239066,-6.59652180815247,4.49376321464633));
#79273=CARTESIAN_POINT('Ctrl Pts',(0.946087206037529,-8.02749889018125,
4.33496961310882));
#79274=CARTESIAN_POINT('Ctrl Pts',(-3.00980434103269,-7.50179293648743,
4.1761760115713));
#79275=CARTESIAN_POINT('Ctrl Pts',(-6.23206351075639,-5.14754347540663,
4.01738241003379));
#79276=CARTESIAN_POINT('Ctrl Pts',(-7.9352725858267,-1.53859300073383,3.85858880849627));
#79277=CARTESIAN_POINT('Ctrl Pts',(-7.70427855916092,2.44538571925539,3.69979520695874));
#79278=CARTESIAN_POINT('Ctrl Pts',(-5.59538565450209,5.83330770757355,3.54100160542123));
#79279=CARTESIAN_POINT('Ctrl Pts',(-2.12263131073224,7.79937534362048,3.38220800388371));
#79280=CARTESIAN_POINT('Ctrl Pts',(1.86750917446099,7.86436449554542,3.22341440234619));
#79281=CARTESIAN_POINT('Ctrl Pts',(5.40244890917294,6.01243421704986,3.06462080080868));
#79282=CARTESIAN_POINT('Ctrl Pts',(7.62055505981324,2.69498794326032,2.90582719927116));
#79283=CARTESIAN_POINT('Ctrl Pts',(7.98116972938295,-1.27935499062613,2.74703359773365));
#79284=CARTESIAN_POINT('Ctrl Pts',(6.39639398046123,-4.94185829923385,2.58823999619613));
#79285=CARTESIAN_POINT('Ctrl Pts',(3.25251299323007,-7.39979585771028,2.42944639465861));
#79286=CARTESIAN_POINT('Ctrl Pts',(-0.6841600112769,-8.05405142614452,2.27065279312109));
#79287=CARTESIAN_POINT('Ctrl Pts',(-4.45407069196273,-6.74515188068711,
2.11185919158358));
#79288=CARTESIAN_POINT('Ctrl Pts',(-7.13831265794001,-3.79213814459122,
1.95306559004606));
#79289=CARTESIAN_POINT('Ctrl Pts',(-8.08260849775468,0.0851997593911264,
1.79427198850854));
#79290=CARTESIAN_POINT('Ctrl Pts',(-7.05678854826809,3.94177071265802,1.63547838697102));
#79291=CARTESIAN_POINT('Ctrl Pts',(-4.31089366061186,6.83754423547215,1.47668478543351));
#79292=CARTESIAN_POINT('Ctrl Pts',(-0.514229384434719,8.0666843146748,1.31789118389599));
#79293=CARTESIAN_POINT('Ctrl Pts',(3.40777762088571,7.32958787930388,1.15909758235848));
#79294=CARTESIAN_POINT('Ctrl Pts',(6.49914609214958,4.80592667747565,1.00030398082096));
#79295=CARTESIAN_POINT('Ctrl Pts',(8.00636601379248,1.11082449054863,0.841510379283439));
#79296=CARTESIAN_POINT('Ctrl Pts',(7.56204953448809,-2.85502226162395,0.682716777745918));
#79297=CARTESIAN_POINT('Ctrl Pts',(5.27451090081715,-6.12499615304347,0.523923176208404));
#79298=CARTESIAN_POINT('Ctrl Pts',(1.70130605739136,-7.90195491287871,0.365129574670885));
#79299=CARTESIAN_POINT('Ctrl Pts',(-2.28655411685474,-7.75295442590588,
0.206335973133365));
#79300=CARTESIAN_POINT('Ctrl Pts',(-5.71713900016235,-5.71394888633152,
0.0475423715958508));
#79301=CARTESIAN_POINT('Ctrl Pts',(-7.75405266470557,-2.28266027366405,
-0.111251229941669));
#79302=CARTESIAN_POINT('Ctrl Pts',(-7.90122371833486,1.70622209623335,-0.270053878501701));
#79303=CARTESIAN_POINT('Ctrl Pts',(-6.71465618324548,4.08673202951572,-0.375925326549237));
#79304=CARTESIAN_POINT('Ctrl Pts',(-5.87252163179806,5.0634291864415,-0.428865574084263));
#79305=CARTESIAN_POINT('Ctrl Pts',(-1.90986695944544,-7.13093654462969,
20.4289621488151));
#79306=CARTESIAN_POINT('Ctrl Pts',(-3.09565806575062,-6.81334807072271,
20.3760309483026));
#79307=CARTESIAN_POINT('Ctrl Pts',(-5.30454812494481,-5.57551522146613,
20.2701685472776));
#79308=CARTESIAN_POINT('Ctrl Pts',(-7.32553356635487,-2.35748983795403,
20.11137494574));
#79309=CARTESIAN_POINT('Ctrl Pts',(-7.56063717713609,1.43425143228512,19.9525813442025));
#79310=CARTESIAN_POINT('Ctrl Pts',(-5.953005701823,4.87684463875962,19.793787742665));
#79311=CARTESIAN_POINT('Ctrl Pts',(-2.89426681882617,7.13049320113776,19.6349941411275));
#79312=CARTESIAN_POINT('Ctrl Pts',(0.869903311226413,7.6462163794815,19.47620053959));
#79313=CARTESIAN_POINT('Ctrl Pts',(4.42205657114865,6.2981348356096,19.3174069380524));
#79314=CARTESIAN_POINT('Ctrl Pts',(6.89633432763268,3.41492816378902,19.1586133365149));
#79315=CARTESIAN_POINT('Ctrl Pts',(7.6896527724844,-0.300673921684578,18.9998197349774));
#79316=CARTESIAN_POINT('Ctrl Pts',(6.60863471619527,-3.9429797962931,18.8410261334399));
#79317=CARTESIAN_POINT('Ctrl Pts',(3.91677959787454,-6.62419798998166,18.6822325319024));
#79318=CARTESIAN_POINT('Ctrl Pts',(0.270218443725032,-7.69078228866305,
18.5234389303648));
#79319=CARTESIAN_POINT('Ctrl Pts',(-3.44220744358733,-6.8827584039626,18.3646453288273));
#79320=CARTESIAN_POINT('Ctrl Pts',(-6.31560394056081,-4.39707863597438,
18.2058517272898));
#79321=CARTESIAN_POINT('Ctrl Pts',(-7.64958747996416,-0.839622068191634,
18.0470581257523));
#79322=CARTESIAN_POINT('Ctrl Pts',(-7.11900300236244,2.92249043907889,17.8882645242148));
#79323=CARTESIAN_POINT('Ctrl Pts',(-4.85317909561161,5.97225304923554,17.7294709226773));
#79324=CARTESIAN_POINT('Ctrl Pts',(-1.4044047778941,7.56629375779054,17.5706773211398));
#79325=CARTESIAN_POINT('Ctrl Pts',(2.38668974314694,7.31606902544708,17.4118837196022));
#79326=CARTESIAN_POINT('Ctrl Pts',(5.59603452864965,5.28257053942491,17.2530901180647));
#79327=CARTESIAN_POINT('Ctrl Pts',(7.44135971516583,1.9614585217979,17.0942965165272));
#79328=CARTESIAN_POINT('Ctrl Pts',(7.47287184199119,-1.83775416564101,16.9355029149897));
#79329=CARTESIAN_POINT('Ctrl Pts',(5.6828899072011,-5.1890188135372,16.7767093134522));
#79330=CARTESIAN_POINT('Ctrl Pts',(2.50771758758178,-7.2754729359924,16.6179157119147));
#79331=CARTESIAN_POINT('Ctrl Pts',(-1.27870470270501,-7.58854849272236,
16.4591221103771));
#79332=CARTESIAN_POINT('Ctrl Pts',(-4.75344587870222,-6.05193408925435,
16.3003285088396));
#79333=CARTESIAN_POINT('Ctrl Pts',(-7.06954635732759,-3.04017569298274,
16.1415349073021));
#79334=CARTESIAN_POINT('Ctrl Pts',(-7.66246236508284,0.712618022727699,
15.9827413057646));
#79335=CARTESIAN_POINT('Ctrl Pts',(-6.3876720888831,4.29171285473144,15.8239477042271));
#79336=CARTESIAN_POINT('Ctrl Pts',(-3.55590251128483,6.82471327403968,15.6651541026895));
#79337=CARTESIAN_POINT('Ctrl Pts',(0.142609524418191,7.69420668205179,15.506360501152));
#79338=CARTESIAN_POINT('Ctrl Pts',(3.8063608406262,6.68825620722965,15.3475668996145));
#79339=CARTESIAN_POINT('Ctrl Pts',(6.5423210993011,4.05205979425698,15.188773298077));
#79340=CARTESIAN_POINT('Ctrl Pts',(7.68360674209098,0.428183810400089,15.0299796965395));
#79341=CARTESIAN_POINT('Ctrl Pts',(6.95203221123971,-3.30006092011662,14.871186095002));
#79342=CARTESIAN_POINT('Ctrl Pts',(4.52591699248759,-6.22392394874059,14.7123924934644));
#79343=CARTESIAN_POINT('Ctrl Pts',(0.996620680668604,-7.63072088085122,
14.5535988919269));
#79344=CARTESIAN_POINT('Ctrl Pts',(-2.77559946154721,-7.17754843743,14.3948052903894));
#79345=CARTESIAN_POINT('Ctrl Pts',(-5.87127408757524,-4.97486628274192,
14.2360116888519));
#79346=CARTESIAN_POINT('Ctrl Pts',(-7.53584015010604,-1.55957275388004,
14.0772180873144));
#79347=CARTESIAN_POINT('Ctrl Pts',(-7.36356378097696,2.23586278337454,13.9184244857769));
#79348=CARTESIAN_POINT('Ctrl Pts',(-5.39643691983716,5.48631228721201,13.7596308842393));
#79349=CARTESIAN_POINT('Ctrl Pts',(-2.11394188253015,7.39948671597428,13.6008372827018));
#79350=CARTESIAN_POINT('Ctrl Pts',(1.68382126961865,7.50905452600891,13.4420436811643));
#79351=CARTESIAN_POINT('Ctrl Pts',(5.0711571444156,5.78830883412743,13.2832500796268));
#79352=CARTESIAN_POINT('Ctrl Pts',(7.22241098523436,2.65667715444709,13.1244564780893));
#79353=CARTESIAN_POINT('Ctrl Pts',(7.61321997951827,-1.12251302266783,12.9656628765518));
#79354=CARTESIAN_POINT('Ctrl Pts',(6.14832539976301,-4.6280934218341,12.8068692750142));
#79355=CARTESIAN_POINT('Ctrl Pts',(3.18479168316541,-7.00558747553948,12.6480756734767));
#79356=CARTESIAN_POINT('Ctrl Pts',(-0.555027143401427,-7.67548687789136,
12.4892820719392));
#79357=CARTESIAN_POINT('Ctrl Pts',(-4.15955947404802,-6.47450530345387,
12.3304884704017));
#79358=CARTESIAN_POINT('Ctrl Pts',(-6.75020945226223,-3.69537904594167,
12.1716948688642));
#79359=CARTESIAN_POINT('Ctrl Pts',(-7.69551254180441,-0.0155132693518444,
12.0129012673267));
#79360=CARTESIAN_POINT('Ctrl Pts',(-6.76505344841895,3.6681338283424,11.8541076657891));
#79361=CARTESIAN_POINT('Ctrl Pts',(-4.18562927894601,6.45768236148427,11.6953140642516));
#79362=CARTESIAN_POINT('Ctrl Pts',(-0.585968306459459,7.67318676212303,
11.5365204627141));
#79363=CARTESIAN_POINT('Ctrl Pts',(3.15652099405334,7.01837083351226,11.3777268611766));
#79364=CARTESIAN_POINT('Ctrl Pts',(6.12961609527162,4.65284434160248,11.2189332596391));
#79365=CARTESIAN_POINT('Ctrl Pts',(7.6086324064267,1.15319852864476,11.0601396581015));
#79366=CARTESIAN_POINT('Ctrl Pts',(7.23306335315761,-2.62753657858524,10.901346056564));
#79367=CARTESIAN_POINT('Ctrl Pts',(5.09445296497157,-5.76781613180305,10.7425524550265));
#79368=CARTESIAN_POINT('Ctrl Pts',(1.71408224406093,-7.50220474281994,10.583758853489));
#79369=CARTESIAN_POINT('Ctrl Pts',(-2.08409179201178,-7.40794946966191,
10.4249652519515));
#79370=CARTESIAN_POINT('Ctrl Pts',(-5.37427359911089,-5.50802480245821,
10.266171650414));
#79371=CARTESIAN_POINT('Ctrl Pts',(-7.35448948475168,-2.26553268819318,
10.1073780488764));
#79372=CARTESIAN_POINT('Ctrl Pts',(-7.54206671568352,1.52917742553764,9.9485844473389));
#79373=CARTESIAN_POINT('Ctrl Pts',(-5.8912838049685,4.95115431711746,9.78979084580139));
#79374=CARTESIAN_POINT('Ctrl Pts',(-2.8045150115428,7.16629956760294,9.63099724426387));
#79375=CARTESIAN_POINT('Ctrl Pts',(0.965847391993691,7.63467699107004,9.47220364272635));
#79376=CARTESIAN_POINT('Ctrl Pts',(4.50078687827297,6.24212074690652,9.31341004118883));
#79377=CARTESIAN_POINT('Ctrl Pts',(6.9386706747824,3.32806298160199,9.15461643965132));
#79378=CARTESIAN_POINT('Ctrl Pts',(7.6852706249148,-0.397201918949031,8.9958228381138));
#79379=CARTESIAN_POINT('Ctrl Pts',(6.5586048340755,-4.02564983239184,8.83702923657629));
#79380=CARTESIAN_POINT('Ctrl Pts',(3.83329530720239,-6.67285553795188,8.67823563503877));
#79381=CARTESIAN_POINT('Ctrl Pts',(0.173629513065194,-7.69356918047714,
8.51944203350125));
#79382=CARTESIAN_POINT('Ctrl Pts',(-3.52835804621482,-6.83899432960039,
8.36064843196373));
#79383=CARTESIAN_POINT('Ctrl Pts',(-6.37031704274931,-4.31743149539779,
8.20185483042622));
#79384=CARTESIAN_POINT('Ctrl Pts',(-7.65952698752967,-0.743505393322568,
8.0430612288887));
#79385=CARTESIAN_POINT('Ctrl Pts',(-7.08174613939356,3.01164831276487,7.88426762735118));
#79386=CARTESIAN_POINT('Ctrl Pts',(-4.77780715361458,6.0327201779516,7.72547402581366));
#79387=CARTESIAN_POINT('Ctrl Pts',(-1.30928946987534,7.58333139369951,7.56668042427615));
#79388=CARTESIAN_POINT('Ctrl Pts',(2.47836428969461,7.28552430441087,7.40788682273863));
#79389=CARTESIAN_POINT('Ctrl Pts',(5.66192287238406,5.211888652856,7.24909322120111));
#79390=CARTESIAN_POINT('Ctrl Pts',(7.46540173342043,1.8678680095869,7.0902996196636));
#79391=CARTESIAN_POINT('Ctrl Pts',(7.44920735296156,-1.93144084951585,6.93150601812608));
#79392=CARTESIAN_POINT('Ctrl Pts',(5.61728707126261,-5.25996577000468,6.77271241658856));
#79393=CARTESIAN_POINT('Ctrl Pts',(2.41616693423443,-7.30638702016992,6.61391881505104));
#79394=CARTESIAN_POINT('Ctrl Pts',(-1.37388792783737,-7.57189447260971,
6.45512521351352));
#79395=CARTESIAN_POINT('Ctrl Pts',(-4.82906099943468,-5.99177134129249,
6.29633161197601));
#79396=CARTESIAN_POINT('Ctrl Pts',(-7.10716237469161,-2.95116873837517,
6.1375380104385));
#79397=CARTESIAN_POINT('Ctrl Pts',(-7.65291046770089,0.8087739585009,5.97874440890097));
#79398=CARTESIAN_POINT('Ctrl Pts',(-6.33328052816671,4.37157999974144,5.81995080736346));
#79399=CARTESIAN_POINT('Ctrl Pts',(-3.46992909587,6.86882420886064,5.66115720582594));
#79400=CARTESIAN_POINT('Ctrl Pts',(0.239208986778566,7.69180947523007,5.50236360428843));
#79401=CARTESIAN_POINT('Ctrl Pts',(3.89004046947315,6.63993517200708,5.34357000275091));
#79402=CARTESIAN_POINT('Ctrl Pts',(6.59268419169601,3.96959306367241,5.18477640121339));
#79403=CARTESIAN_POINT('Ctrl Pts',(7.6883774186021,0.331672446434416,5.02598279967587));
#79404=CARTESIAN_POINT('Ctrl Pts',(6.91004763124565,-3.3870925107701,4.86718919813835));
#79405=CARTESIAN_POINT('Ctrl Pts',(4.44741079370755,-6.28026203072761,4.70839559660083));
#79406=CARTESIAN_POINT('Ctrl Pts',(0.900728555235199,-7.64263318578086,
4.54960199506332));
#79407=CARTESIAN_POINT('Ctrl Pts',(-2.86550404480521,-7.14213137038015,
4.3908083935258));
#79408=CARTESIAN_POINT('Ctrl Pts',(-5.93327710844758,-4.9007526663768,4.23201479198829));
#79409=CARTESIAN_POINT('Ctrl Pts',(-7.55482852533749,-1.46482759919173,
4.07322119045077));
#79410=CARTESIAN_POINT('Ctrl Pts',(-7.33490914097327,2.32814557880231,3.91442758891325));
#79411=CARTESIAN_POINT('Ctrl Pts',(-5.32712376237705,5.55363901990728,3.75563398737573));
#79412=CARTESIAN_POINT('Ctrl Pts',(-2.02086511857661,7.42544666090499,3.59684038583822));
#79413=CARTESIAN_POINT('Ctrl Pts',(1.77797440855997,7.48732001099973,3.4380467843007));
#79414=CARTESIAN_POINT('Ctrl Pts',(5.14343706334645,5.72417759294292,3.27925318276318));
#79415=CARTESIAN_POINT('Ctrl Pts',(7.25519963203433,2.56578101999284,3.12045958122566));
#79416=CARTESIAN_POINT('Ctrl Pts',(7.59852520312894,-1.21801834438284,2.96166597968815));
#79417=CARTESIAN_POINT('Ctrl Pts',(6.08972901437527,-4.7049287398031,2.80287237815062));
#79418=CARTESIAN_POINT('Ctrl Pts',(3.09657641555679,-7.04502437979951,2.64407877661313));
#79419=CARTESIAN_POINT('Ctrl Pts',(-0.651359044467085,-7.66791270251401,
2.48528517507559));
#79420=CARTESIAN_POINT('Ctrl Pts',(-4.2405273358362,-6.42176627012995,2.32649157353808));
#79421=CARTESIAN_POINT('Ctrl Pts',(-6.79607757738601,-3.61033009476553,
2.16769797200056));
#79422=CARTESIAN_POINT('Ctrl Pts',(-7.69510065061119,0.0811149920356376,
2.00890437046304));
#79423=CARTESIAN_POINT('Ctrl Pts',(-6.7184620118726,3.75278876664151,1.85011076892552));
#79424=CARTESIAN_POINT('Ctrl Pts',(-4.10421470020542,6.50972901997924,1.69131716738801));
#79425=CARTESIAN_POINT('Ctrl Pts',(-0.489575472055369,7.67993992723675,
1.53252356585049));
#79426=CARTESIAN_POINT('Ctrl Pts',(3.24439712685584,6.97818241158302,1.37372996431298));
#79427=CARTESIAN_POINT('Ctrl Pts',(6.18755483901151,4.57551414409174,1.21493636277546));
#79428=CARTESIAN_POINT('Ctrl Pts',(7.62251349163834,1.05756777187836,1.05614276123794));
#79429=CARTESIAN_POINT('Ctrl Pts',(7.1994990613437,-2.71814274674258,0.897349159700425));
#79430=CARTESIAN_POINT('Ctrl Pts',(5.02163283991908,-5.83134292541437,0.73855555816291));
#79431=CARTESIAN_POINT('Ctrl Pts',(1.61973963637579,-7.52310821538431,0.579761956625391));
#79432=CARTESIAN_POINT('Ctrl Pts',(-2.17692890570593,-7.38125132047662,
0.42096835508787));
#79433=CARTESIAN_POINT('Ctrl Pts',(-5.44303983695429,-5.44000266807223,
0.262174753550357));
#79434=CARTESIAN_POINT('Ctrl Pts',(-7.38229690595861,-2.17322174665223,
0.103381152012836));
#79435=CARTESIAN_POINT('Ctrl Pts',(-7.52241207680334,1.62441998353129,-0.0554214965471939));
#79436=CARTESIAN_POINT('Ctrl Pts',(-6.39273264054252,3.89080014303998,-0.16129294459473));
#79437=CARTESIAN_POINT('Ctrl Pts',(-5.59097289471971,4.82067110360889,-0.214233192129757));
#79438=CARTESIAN_POINT('Ctrl Pts',(-1.81369038328508,-6.77183872460225,
20.6435945307695));
#79439=CARTESIAN_POINT('Ctrl Pts',(-2.93976773409445,-6.47024328722449,
20.590663330257));
#79440=CARTESIAN_POINT('Ctrl Pts',(-5.03742309080986,-5.29474489781683,
20.484800929232));
#79441=CARTESIAN_POINT('Ctrl Pts',(-6.95663628087881,-2.23877198704513,
20.3260073276945));
#79442=CARTESIAN_POINT('Ctrl Pts',(-7.17990060609302,1.36202577728435,20.167213726157));
#79443=CARTESIAN_POINT('Ctrl Pts',(-5.65322581221712,4.63125778387307,20.0084201246195));
#79444=CARTESIAN_POINT('Ctrl Pts',(-2.7485180944176,6.77141770688483,19.8496265230819));
#79445=CARTESIAN_POINT('Ctrl Pts',(0.826096949924359,7.26117023355868,19.6908329215445));
#79446=CARTESIAN_POINT('Ctrl Pts',(4.19937181371192,5.98097502419469,19.5320393200069));
#79447=CARTESIAN_POINT('Ctrl Pts',(6.54905054411643,3.24296011281956,19.3732457184694));
#79448=CARTESIAN_POINT('Ctrl Pts',(7.30241926814944,-0.285532663710926,
19.2144521169319));
#79449=CARTESIAN_POINT('Ctrl Pts',(6.27583883376233,-3.74442026061367,19.0556585153944));
#79450=CARTESIAN_POINT('Ctrl Pts',(3.71953944487051,-6.29061837631592,18.8968649138569));
#79451=CARTESIAN_POINT('Ctrl Pts',(0.256610854670558,-7.30349190445053,
18.7380713123193));
#79452=CARTESIAN_POINT('Ctrl Pts',(-3.26886566984719,-6.53615827322664,
18.5792777107818));
#79453=CARTESIAN_POINT('Ctrl Pts',(-5.99756442457044,-4.17565171080327,
18.4204841092443));
#79454=CARTESIAN_POINT('Ctrl Pts',(-7.26437157305314,-0.79734060173242,
18.2616905077068));
#79455=CARTESIAN_POINT('Ctrl Pts',(-6.76050612850616,2.77532043705234,18.1028969061693));
#79456=CARTESIAN_POINT('Ctrl Pts',(-4.60878398389947,5.67150390678975,17.9441033046317));
#79457=CARTESIAN_POINT('Ctrl Pts',(-1.33368213283598,7.18527233415214,17.7853097030942));
#79458=CARTESIAN_POINT('Ctrl Pts',(2.26650145112079,6.94764835282353,17.6265161015567));
#79459=CARTESIAN_POINT('Ctrl Pts',(5.31423089914606,5.01655224673973,17.4677225000192));
#79460=CARTESIAN_POINT('Ctrl Pts',(7.06662968706476,1.86268391136018,17.3089288984817));
#79461=CARTESIAN_POINT('Ctrl Pts',(7.09655493452627,-1.74520902651409,17.1501352969442));
#79462=CARTESIAN_POINT('Ctrl Pts',(5.39671243747327,-4.92771157396768,16.9913416954066));
#79463=CARTESIAN_POINT('Ctrl Pts',(2.38143460731556,-6.90909659052469,16.8325480938691));
#79464=CARTESIAN_POINT('Ctrl Pts',(-1.21431202884984,-7.20640637101727,
16.6737544923316));
#79465=CARTESIAN_POINT('Ctrl Pts',(-4.51407310599876,-5.74717239003019,
16.5149608907941));
#79466=CARTESIAN_POINT('Ctrl Pts',(-6.71354000814598,-2.88707932800769,
16.3561672892566));
#79467=CARTESIAN_POINT('Ctrl Pts',(-7.27659810810584,0.676732192462313,
16.1973736877191));
#79468=CARTESIAN_POINT('Ctrl Pts',(-6.06600338410468,4.07559191175679,16.0385800861815));
#79469=CARTESIAN_POINT('Ctrl Pts',(-3.3768353113398,6.4810361646331,15.879786484644));
#79470=CARTESIAN_POINT('Ctrl Pts',(0.135428031634848,7.30674385314103,15.7209928831065));
#79471=CARTESIAN_POINT('Ctrl Pts',(3.61468112625038,6.35145076677037,15.562199281569));
#79472=CARTESIAN_POINT('Ctrl Pts',(6.21286462048166,3.84800723683599,15.4034056800315));
#79473=CARTESIAN_POINT('Ctrl Pts',(7.2966777021585,0.406621443111669,15.244612078494));
#79474=CARTESIAN_POINT('Ctrl Pts',(6.60194360840439,-3.13387732348034,15.0858184769564));
#79475=CARTESIAN_POINT('Ctrl Pts',(4.29800205937108,-5.91050122957581,14.9270248754189));
#79476=CARTESIAN_POINT('Ctrl Pts',(0.94643311952814,-7.24645505315777,14.7682312738814));
#79477=CARTESIAN_POINT('Ctrl Pts',(-2.63582655658965,-6.81610334800993,
14.6094376723439));
#79478=CARTESIAN_POINT('Ctrl Pts',(-5.57561001702343,-4.72434327978433,
14.4506440708064));
#79479=CARTESIAN_POINT('Ctrl Pts',(-7.15635230120401,-1.4810362008498,14.2918504692689));
#79480=CARTESIAN_POINT('Ctrl Pts',(-6.9927513799925,2.12326979557197,14.1330568677313));
#79481=CARTESIAN_POINT('Ctrl Pts',(-5.12468457402663,5.2100340213773,13.9742632661938));
#79482=CARTESIAN_POINT('Ctrl Pts',(-2.00748855526656,7.02686531731248,13.8154696646563));
#79483=CARTESIAN_POINT('Ctrl Pts',(1.59902784263307,7.13091554049405,13.6566760631188));
#79484=CARTESIAN_POINT('Ctrl Pts',(4.81578515166555,5.49682270590684,13.4978824615813));
#79485=CARTESIAN_POINT('Ctrl Pts',(6.85870671947516,2.52289290763632,13.3390888600438));
#79486=CARTESIAN_POINT('Ctrl Pts',(7.22983545759411,-1.06598580820313,13.1802952585062));
#79487=CARTESIAN_POINT('Ctrl Pts',(5.83870965237047,-4.39503311506197,13.0215016569687));
#79488=CARTESIAN_POINT('Ctrl Pts',(3.02441278433374,-6.65280195084252,12.8627080554312));
#79489=CARTESIAN_POINT('Ctrl Pts',(-0.527077233034936,-7.2889667359367,
12.7039144538937));
#79490=CARTESIAN_POINT('Ctrl Pts',(-3.95009347613082,-6.14846387457909,
12.5451208523562));
#79491=CARTESIAN_POINT('Ctrl Pts',(-6.41028418664454,-3.50928812348463,
12.3863272508187));
#79492=CARTESIAN_POINT('Ctrl Pts',(-7.30798395275296,-0.0147320562291548,
12.2275336492811));
#79493=CARTESIAN_POINT('Ctrl Pts',(-6.42438067276146,3.4834149133608,12.0687400477436));
#79494=CARTESIAN_POINT('Ctrl Pts',(-3.97485046467588,6.13248809788012,11.9099464462061));
#79495=CARTESIAN_POINT('Ctrl Pts',(-0.55646026917181,7.28678244879102,11.7511528446686));
#79496=CARTESIAN_POINT('Ctrl Pts',(2.99756574312083,6.66494156784918,11.592359243131));
#79497=CARTESIAN_POINT('Ctrl Pts',(5.82094250609562,4.41853763454662,11.4335656415936));
#79498=CARTESIAN_POINT('Ctrl Pts',(7.22547890429721,1.0951260615707,11.274772040056));
#79499=CARTESIAN_POINT('Ctrl Pts',(6.86882265826663,-2.49521978520095,11.1159784385185));
#79500=CARTESIAN_POINT('Ctrl Pts',(4.83790784743979,-5.47736196967628,10.957184836981));
#79501=CARTESIAN_POINT('Ctrl Pts',(1.62776494291293,-7.12441069687865,10.7983912354435));
#79502=CARTESIAN_POINT('Ctrl Pts',(-1.97914164772644,-7.03490190588398,
10.639597633906));
#79503=CARTESIAN_POINT('Ctrl Pts',(-5.10363734795463,-5.23065314351258,
10.4808040323684));
#79504=CARTESIAN_POINT('Ctrl Pts',(-6.98413404478104,-2.15144559115629,
10.3220104308309));
#79505=CARTESIAN_POINT('Ctrl Pts',(-7.16226531103587,1.45217151242805,10.1632168292934));
#79506=CARTESIAN_POINT('Ctrl Pts',(-5.59461209035054,4.70182539506509,10.0044232277559));
#79507=CARTESIAN_POINT('Ctrl Pts',(-2.66328598495193,6.80542094580004,9.84562962621837));
#79508=CARTESIAN_POINT('Ctrl Pts',(0.917209504000515,7.25021194262256,9.68683602468087));
#79509=CARTESIAN_POINT('Ctrl Pts',(4.274137440814,5.92778167818344,9.52804242314334));
#79510=CARTESIAN_POINT('Ctrl Pts',(6.58925492867272,3.16046926454566,9.36924882160583));
#79511=CARTESIAN_POINT('Ctrl Pts',(7.2982577956103,-0.377199729571435,9.21045522006831));
#79512=CARTESIAN_POINT('Ctrl Pts',(6.22832834323901,-3.8229272208585,9.05166161853079));
#79513=CARTESIAN_POINT('Ctrl Pts',(3.64025923406912,-6.33682564033049,8.89286801699328));
#79514=CARTESIAN_POINT('Ctrl Pts',(0.1648859238825,-7.30613845470238,8.73407441545576));
#79515=CARTESIAN_POINT('Ctrl Pts',(-3.35067792317036,-6.49459805856793,
8.57528081391825));
#79516=CARTESIAN_POINT('Ctrl Pts',(-6.04952229880255,-4.10001541990588,
8.41648721238073));
#79517=CARTESIAN_POINT('Ctrl Pts',(-7.2738105495206,-0.706064145002688,
8.25769361084321));
#79518=CARTESIAN_POINT('Ctrl Pts',(-6.72512543680727,2.85998852207193,8.0989000093057));
#79519=CARTESIAN_POINT('Ctrl Pts',(-4.53720760226019,5.72892604780056,7.94010640776816));
#79520=CARTESIAN_POINT('Ctrl Pts',(-1.24335661638905,7.20145199328975,7.78131280623066));
#79521=CARTESIAN_POINT('Ctrl Pts',(2.35355947505446,6.91864179478579,7.62251920469314));
#79522=CARTESIAN_POINT('Ctrl Pts',(5.37680125506048,4.94942973995545,7.46372560315563));
#79523=CARTESIAN_POINT('Ctrl Pts',(7.08946100371092,1.77380640545626,7.30493200161811));
#79524=CARTESIAN_POINT('Ctrl Pts',(7.07408213558805,-1.83417786109458,7.14613840008059));
#79525=CARTESIAN_POINT('Ctrl Pts',(5.33441321182856,-4.99508580233056,6.98734479854307));
#79526=CARTESIAN_POINT('Ctrl Pts',(2.29449423760114,-6.93845391141215,6.82855119700556));
#79527=CARTESIAN_POINT('Ctrl Pts',(-1.30470204225829,-7.19059100965299,
6.66975759546803));
#79528=CARTESIAN_POINT('Ctrl Pts',(-4.58588042044292,-5.69003930184789,
6.51096399393052));
#79529=CARTESIAN_POINT('Ctrl Pts',(-6.74926176803779,-2.80255456212341,
6.352170392393));
#79530=CARTESIAN_POINT('Ctrl Pts',(-7.26752722265067,0.768045933005938,
6.19337679085548));
#79531=CARTESIAN_POINT('Ctrl Pts',(-6.0143508592441,4.15143712816239,6.03458318931797));
#79532=CARTESIAN_POINT('Ctrl Pts',(-3.29519132248241,6.52292577264314,5.87578958778045));
#79533=CARTESIAN_POINT('Ctrl Pts',(0.227162963770855,7.30446736422759,5.71699598624294));
#79534=CARTESIAN_POINT('Ctrl Pts',(3.69414683843833,6.30556306948332,5.55820238470542));
#79535=CARTESIAN_POINT('Ctrl Pts',(6.26069154156504,3.7696933440999,5.39940878316791));
#79536=CARTESIAN_POINT('Ctrl Pts',(7.30120813820126,0.314970172934666,5.24061518163038));
#79537=CARTESIAN_POINT('Ctrl Pts',(6.56207327680621,-3.21652620026706,5.08182158009287));
#79538=CARTESIAN_POINT('Ctrl Pts',(4.22344925502444,-5.96400225330274,4.92302797855534));
#79539=CARTESIAN_POINT('Ctrl Pts',(0.85536990443287,-7.25776748138049,4.76423437701783));
#79540=CARTESIAN_POINT('Ctrl Pts',(-2.72120374857774,-6.78246980427286,
4.60544077548031));
#79541=CARTESIAN_POINT('Ctrl Pts',(-5.63449070613878,-4.65396185734695,
4.4466471739428));
#79542=CARTESIAN_POINT('Ctrl Pts',(-7.17438446484828,-1.39106219764965,
4.28785357240528));
#79543=CARTESIAN_POINT('Ctrl Pts',(-6.96553972278562,2.21090543834923,4.12905997086776));
#79544=CARTESIAN_POINT('Ctrl Pts',(-5.05886187025201,5.27397033224099,3.97026636933025));
#79545=CARTESIAN_POINT('Ctrl Pts',(-1.91909892642098,7.05151797818953,3.81147276779273));
#79546=CARTESIAN_POINT('Ctrl Pts',(1.68843964265895,7.11027552645404,3.6526791662552));
#79547=CARTESIAN_POINT('Ctrl Pts',(4.88442521751996,5.43592096883599,3.4938855647177));
#79548=CARTESIAN_POINT('Ctrl Pts',(6.88984420425543,2.43657409672536,3.33509196318017));
#79549=CARTESIAN_POINT('Ctrl Pts',(7.21588067687493,-1.15668169813955,3.17629836164266));
#79550=CARTESIAN_POINT('Ctrl Pts',(5.7830640482893,-4.46799918037234,3.01750476010513));
#79551=CARTESIAN_POINT('Ctrl Pts',(2.94063983788352,-6.69025290188873,2.85871115856763));
#79552=CARTESIAN_POINT('Ctrl Pts',(-0.618558077657272,-7.28177397888349,
2.6999175570301));
#79553=CARTESIAN_POINT('Ctrl Pts',(-4.02698397970966,-6.09838065957278,
2.54112395549259));
#79554=CARTESIAN_POINT('Ctrl Pts',(-6.45384249683203,-3.42852204493986,
2.38233035395507));
#79555=CARTESIAN_POINT('Ctrl Pts',(-7.3075928034677,0.0770302246801563,
2.22353675241756));
#79556=CARTESIAN_POINT('Ctrl Pts',(-6.38013547547711,3.56380682062498,2.06474315088003));
#79557=CARTESIAN_POINT('Ctrl Pts',(-3.89753573979897,6.18191380448636,1.90594954934252));
#79558=CARTESIAN_POINT('Ctrl Pts',(-0.464921559676021,7.29319553979868,
1.747155947805));
#79559=CARTESIAN_POINT('Ctrl Pts',(3.08101663282597,6.62677694386218,1.58836234626749));
#79560=CARTESIAN_POINT('Ctrl Pts',(5.87596358587343,4.34510161070782,1.42956874472997));
#79561=CARTESIAN_POINT('Ctrl Pts',(7.23866096948422,1.00431105320811,1.27077514319245));
#79562=CARTESIAN_POINT('Ctrl Pts',(6.8369485881993,-2.58126323186122,1.11198154165493));
#79563=CARTESIAN_POINT('Ctrl Pts',(4.768754779021,-5.53768969778528,0.953187940117417));
#79564=CARTESIAN_POINT('Ctrl Pts',(1.53817321536023,-7.14426151788992,0.794394338579897));
#79565=CARTESIAN_POINT('Ctrl Pts',(-2.06730369455713,-7.00954821504736,
0.635600737042377));
#79566=CARTESIAN_POINT('Ctrl Pts',(-5.16894067374621,-5.16605644981294,
0.476807135504864));
#79567=CARTESIAN_POINT('Ctrl Pts',(-7.01054114721167,-2.06378321964041,
0.318013533967343));
#79568=CARTESIAN_POINT('Ctrl Pts',(-7.14360043527182,1.54261787082922,0.159210885407313));
#79569=CARTESIAN_POINT('Ctrl Pts',(-6.07080909783958,3.69486825656423,0.0533394373597762));
#79570=CARTESIAN_POINT('Ctrl Pts',(-5.30942415764135,4.57791302077629,0.000399189824749598));
#79571=CARTESIAN_POINT('Ctrl Pts',(-5.31037376991248,4.57794244025912,-1.11022302462516E-16));
#79572=CARTESIAN_POINT('Ctrl Pts',(-5.44252110837334,4.44698907439619,1.26508291621284E-16));
#79573=CARTESIAN_POINT('Ctrl Pts',(-5.56908400938008,4.31092088233243,4.32413578291971E-15));
#79574=CARTESIAN_POINT('Ctrl Pts',(-5.68993613636022,4.17020851221304,1.99840144432528E-15));
#79575=CARTESIAN_POINT('Ctrl Pts',(-5.81376161366555,4.02603416602499,-3.84553425878751E-16));
#79576=CARTESIAN_POINT('Ctrl Pts',(-5.93159233267655,3.87698397375777,-9.83144615789292E-15));
#79577=CARTESIAN_POINT('Ctrl Pts',(-6.04326669365349,3.72351578252423,-8.21565038222616E-15));
#79578=CARTESIAN_POINT('Ctrl Pts',(-6.15586096386687,3.56878340848829,-6.58654460912372E-15));
#79579=CARTESIAN_POINT('Ctrl Pts',(-6.26219748724818,3.40955944596802,-1.19427616521068E-14));
#79580=CARTESIAN_POINT('Ctrl Pts',(-6.36207781039616,3.24627111619497,-9.10382880192628E-15));
#79581=CARTESIAN_POINT('Ctrl Pts',(-6.46207486290856,3.08279195260851,-6.26157811278843E-15));
#79582=CARTESIAN_POINT('Ctrl Pts',(-6.55560105221217,2.91523834903128,1.65940183112773E-14));
#79583=CARTESIAN_POINT('Ctrl Pts',(-6.64241781295179,2.7440052051437,9.99200722162641E-15));
#79584=CARTESIAN_POINT('Ctrl Pts',(-6.69138001066649,2.64743455478877,6.2686596844429E-15));
#79585=CARTESIAN_POINT('Ctrl Pts',(-6.73820743199069,2.54969301070825,-5.70522088311913E-15));
#79586=CARTESIAN_POINT('Ctrl Pts',(-6.7828509533718,2.4508477193249,-6.21724893790088E-15));
#79587=CARTESIAN_POINT('Ctrl Pts',(-6.79660110048274,2.42040349683309,-6.92406093104009E-15));
#79588=CARTESIAN_POINT('Ctrl Pts',(-6.81014404104715,2.38985455306603,7.73134273691482E-16));
#79589=CARTESIAN_POINT('Ctrl Pts',(-6.82347824501989,2.35920280883552,1.99840144432528E-15));
#79590=CARTESIAN_POINT('Ctrl Pts',(-6.83289223867303,2.33756257247543,2.6022547736133E-15));
#79591=CARTESIAN_POINT('Ctrl Pts',(-6.84220312213329,2.31586888580966,6.65976333931259E-16));
#79592=CARTESIAN_POINT('Ctrl Pts',(-6.85140731350048,2.29412958992203,-3.33066907387547E-16));
#79593=CARTESIAN_POINT('Ctrl Pts',(-6.92787174140525,2.11352895301797,1.48312058419164E-15));
#79594=CARTESIAN_POINT('Ctrl Pts',(-6.9968154363246,1.93016662573821,-4.84967905120705E-15));
#79595=CARTESIAN_POINT('Ctrl Pts',(-7.05806709983238,1.74450817174022,-7.38298311375729E-15));
#79596=CARTESIAN_POINT('Ctrl Pts',(-7.08072012930876,1.6758451152598,-8.31988846971198E-15));
#79597=CARTESIAN_POINT('Ctrl Pts',(-7.10232070581907,1.60686761954515,-1.29953418837246E-14));
#79598=CARTESIAN_POINT('Ctrl Pts',(-7.12285886516232,1.53759799276406,-1.52655665885959E-14));
#79599=CARTESIAN_POINT('Ctrl Pts',(-7.17789503540859,1.35197595581785,-1.15950958872121E-14));
#79600=CARTESIAN_POINT('Ctrl Pts',(-7.2253056020522,1.16425810273759,-1.12411624720764E-15));
#79601=CARTESIAN_POINT('Ctrl Pts',(-7.26516741253555,0.974925030014523,
-2.38697950294409E-15));
#79602=CARTESIAN_POINT('Ctrl Pts',(-7.30539133219011,0.783872034357297,
-3.66131475057827E-15));
#79603=CARTESIAN_POINT('Ctrl Pts',(-7.33792888466284,0.591173700608657,
-1.51778296889488E-15));
#79604=CARTESIAN_POINT('Ctrl Pts',(-7.36281046690392,0.397301655480222,
1.66533453693773E-15));
#79605=CARTESIAN_POINT('Ctrl Pts',(-7.38777154345532,0.202810207438947,
4.85862180321062E-15));
#79606=CARTESIAN_POINT('Ctrl Pts',(-7.40502777710334,0.00713684282182964,
4.74315758813333E-15));
#79607=CARTESIAN_POINT('Ctrl Pts',(-7.41455912394538,-0.189254417725043,
1.94289029309402E-15));
#79608=CARTESIAN_POINT('Ctrl Pts',(-7.41891547422354,-0.279016036590548,
6.63013963776067E-16));
#79609=CARTESIAN_POINT('Ctrl Pts',(-7.42165739195025,-0.368927726290736,
-8.85908993222617E-15));
#79610=CARTESIAN_POINT('Ctrl Pts',(-7.42277933840189,-0.458945409812431,
5.55111512312578E-16));
#79611=CARTESIAN_POINT('Ctrl Pts',(-7.42308627605976,-0.48357209044044,
-2.85004532978439E-15));
#79612=CARTESIAN_POINT('Ctrl Pts',(-7.42327183994005,-0.508199168176247,
4.55160162443761E-15));
#79613=CARTESIAN_POINT('Ctrl Pts',(-7.42333615702577,-0.532819130412786,
9.04831765069503E-15));
#79614=CARTESIAN_POINT('Ctrl Pts',(-7.4238573231957,-0.732316531096511,
5.3206392005416E-15));
#79615=CARTESIAN_POINT('Ctrl Pts',(-7.41642317468771,-0.931480295265724,
2.0508515330919E-15));
#79616=CARTESIAN_POINT('Ctrl Pts',(-7.40111960803424,-1.12981272812747,
-3.88578058618805E-15));
#79617=CARTESIAN_POINT('Ctrl Pts',(-7.38567043395387,-1.3300322162014,1.32328955243151E-15));
#79618=CARTESIAN_POINT('Ctrl Pts',(-7.36220152785829,-1.52940517206027,
-1.20070939886438E-14));
#79619=CARTESIAN_POINT('Ctrl Pts',(-7.33075075935929,-1.72743569513311,
-6.99440505513849E-15));
#79620=CARTESIAN_POINT('Ctrl Pts',(-7.30904612801572,-1.86409943033589,
-3.61599122083957E-15));
#79621=CARTESIAN_POINT('Ctrl Pts',(-7.28353901753502,-2.00012416283928,
4.47127839975347E-15));
#79622=CARTESIAN_POINT('Ctrl Pts',(-7.25422750746073,-2.13534865261956,
6.77236045021345E-15));
#79623=CARTESIAN_POINT('Ctrl Pts',(-7.21194426750884,-2.33041637633158,
3.05948464044368E-15));
#79624=CARTESIAN_POINT('Ctrl Pts',(-7.16174660423667,-2.52381943143324,
-4.47725060636341E-15));
#79625=CARTESIAN_POINT('Ctrl Pts',(-7.10388082685099,-2.71516162535246,
-5.55111512312578E-15));
#79626=CARTESIAN_POINT('Ctrl Pts',(-7.0646932418533,-2.84474147075709,-9.08304634261343E-15));
#79627=CARTESIAN_POINT('Ctrl Pts',(-7.02198779033188,-2.97337609690067,
5.42360386022428E-15));
#79628=CARTESIAN_POINT('Ctrl Pts',(-6.97582777173374,-3.10093944226419,
-9.10382880192628E-15));
#79629=CARTESIAN_POINT('Ctrl Pts',(-6.95395173385994,-3.16139393641793,
1.05087312514034E-15));
#79630=CARTESIAN_POINT('Ctrl Pts',(-6.93129965751152,-3.22160777669937,
-3.3264548240337E-15));
#79631=CARTESIAN_POINT('Ctrl Pts',(-6.90787748303903,-3.28156724782363,
-4.38538094726937E-15));
#79632=CARTESIAN_POINT('Ctrl Pts',(-6.89397770438652,-3.31714991235063,
5.87276203710888E-15));
#79633=CARTESIAN_POINT('Ctrl Pts',(-6.8798046872329,-3.35264758566453,1.41800447596743E-14));
#79634=CARTESIAN_POINT('Ctrl Pts',(-6.86537571403821,-3.38801888857102,
1.18793863634892E-14));
#79635=CARTESIAN_POINT('Ctrl Pts',(-6.78527926138308,-3.58436798773231,
-8.91763310105958E-16));
#79636=CARTESIAN_POINT('Ctrl Pts',(-6.69720860879802,-3.77706587145206,
1.31933643606969E-14));
#79637=CARTESIAN_POINT('Ctrl Pts',(-6.60153595221269,-3.96566681700067,
7.7715611723761E-15));
#79638=CARTESIAN_POINT('Ctrl Pts',(-6.50894990986814,-4.14818307351552,
2.52467750159629E-15));
#79639=CARTESIAN_POINT('Ctrl Pts',(-6.40924387087696,-4.32686313181129,
2.03372667533341E-14));
#79640=CARTESIAN_POINT('Ctrl Pts',(-6.30270053211344,-4.50129762818047,
1.2712053631958E-14));
#79641=CARTESIAN_POINT('Ctrl Pts',(-6.1908293138171,-4.68445501603969,4.70552885474135E-15));
#79642=CARTESIAN_POINT('Ctrl Pts',(-6.07142002024269,-4.86293253556795,
7.3181577952022E-15));
#79643=CARTESIAN_POINT('Ctrl Pts',(-5.94474116946604,-5.03623808905791,
7.46624984060418E-15));
#79644=CARTESIAN_POINT('Ctrl Pts',(-5.82468128040108,-5.20048843865281,
7.60660408626838E-15));
#79645=CARTESIAN_POINT('Ctrl Pts',(-5.69809095197815,-5.36009364644713,
2.44554910442882E-14));
#79646=CARTESIAN_POINT('Ctrl Pts',(-5.56515303095831,-5.51460913021791,
5.27355936696949E-16));
#79647=CARTESIAN_POINT('Ctrl Pts',(-5.55782409690619,-5.52312764609283,
-7.91814115371847E-16));
#79648=CARTESIAN_POINT('Ctrl Pts',(-5.55047585952526,-5.5316306845626,5.34033577522075E-15));
#79649=CARTESIAN_POINT('Ctrl Pts',(-5.54310834577199,-5.54011816828261,
4.46864767411626E-15));
#79650=CARTESIAN_POINT('Ctrl Pts',(-5.46343909916247,-5.63189830690586,
1.04620899136104E-14));
#79651=CARTESIAN_POINT('Ctrl Pts',(-5.38151618195913,-5.72185994455588,
-5.7452322777736E-15));
#79652=CARTESIAN_POINT('Ctrl Pts',(-5.29741727864766,-5.80994862150633,
3.10862446895044E-15));
#79653=CARTESIAN_POINT('Ctrl Pts',(-5.27398864270865,-5.83448874582851,
-2.19216472326236E-15));
#79654=CARTESIAN_POINT('Ctrl Pts',(-5.2503884899981,-5.8588860528994,1.27922499778416E-14));
#79655=CARTESIAN_POINT('Ctrl Pts',(-5.22663715390791,-5.88312049455735,
1.47937218031302E-14));
#79656=CARTESIAN_POINT('Ctrl Pts',(-5.08244539987714,-6.0302451294557,6.10094433106069E-15));
#79657=CARTESIAN_POINT('Ctrl Pts',(-4.93255824560136,-6.17150517691054,
4.5988494700527E-15));
#79658=CARTESIAN_POINT('Ctrl Pts',(-4.77743786746376,-6.30670076408454,
6.46704911844154E-15));
#79659=CARTESIAN_POINT('Ctrl Pts',(-4.62024030664534,-6.44370672546966,
8.36026541519431E-15));
#79660=CARTESIAN_POINT('Ctrl Pts',(-4.4576680003625,-6.57448521633667,2.56788104009255E-14));
#79661=CARTESIAN_POINT('Ctrl Pts',(-4.29015760295661,-6.69879808025457,
1.60982338570648E-14));
#79662=CARTESIAN_POINT('Ctrl Pts',(-4.16413488960682,-6.79232209224324,
8.89050066431821E-15));
#79663=CARTESIAN_POINT('Ctrl Pts',(-4.03531626522646,-6.88218600290244,
8.03682837398228E-15));
#79664=CARTESIAN_POINT('Ctrl Pts',(-3.90387378481224,-6.96827480951185,
-1.36002320516582E-15));
#79665=CARTESIAN_POINT('Ctrl Pts',(-3.87679878053257,-6.98600769769256,
-2.77050060624404E-15));
#79666=CARTESIAN_POINT('Ctrl Pts',(-3.84961241206961,-7.00358036772389,
5.09502761441384E-15));
#79667=CARTESIAN_POINT('Ctrl Pts',(-3.82231612917412,-7.02099174562584,
6.86950496486816E-15));
#79668=CARTESIAN_POINT('Ctrl Pts',(-3.79414288534319,-7.03896250732048,
3.1539969567683E-15));
#79669=CARTESIAN_POINT('Ctrl Pts',(-3.7658597368087,-7.05675683475663,-6.31539703715498E-15));
#79670=CARTESIAN_POINT('Ctrl Pts',(-3.73747339603306,-7.07437079137119,
-9.56179579958416E-15));
#79671=CARTESIAN_POINT('Ctrl Pts',(-3.55786207395122,-7.18582108570944,
-4.03029781972554E-15));
#79672=CARTESIAN_POINT('Ctrl Pts',(-3.37406099776166,-7.29009223339221,
-7.83203303092207E-15));
#79673=CARTESIAN_POINT('Ctrl Pts',(-3.18652216952045,-7.38694978403964,
-6.44623243672982E-15));
#79674=CARTESIAN_POINT('Ctrl Pts',(-2.99883762064898,-7.48388259453305,
-5.05935505359788E-15));
#79675=CARTESIAN_POINT('Ctrl Pts',(-2.80740895502159,-7.57339073115159,
-1.95077283645645E-15));
#79676=CARTESIAN_POINT('Ctrl Pts',(-2.61265463314995,-7.65520051975289,
-4.70110061989715E-15));
#79677=CARTESIAN_POINT('Ctrl Pts',(-2.50764369183966,-7.69931211032946,
-7.77693376164546E-15));
#79678=CARTESIAN_POINT('Ctrl Pts',(-2.40166532647539,-7.74118482989975,
-1.74561535473132E-14));
#79679=CARTESIAN_POINT('Ctrl Pts',(-2.2947818331751,-7.78077040809537,-1.54546514474774E-14));
#79680=CARTESIAN_POINT('Ctrl Pts',(-2.23095371052338,-7.80440991558425,
-1.29169104133784E-14));
#79681=CARTESIAN_POINT('Ctrl Pts',(-2.16680276244212,-7.82723371232969,
-4.1499230043281E-15));
#79682=CARTESIAN_POINT('Ctrl Pts',(-2.10234495552166,-7.84924110414384,
5.60532523175006E-16));
#79683=CARTESIAN_POINT('Ctrl Pts',(-2.10208451021637,-7.84862588447229,
20.));
#79684=CARTESIAN_POINT('Ctrl Pts',(-2.29993845398409,-7.78098052187409,
20.));
#79685=CARTESIAN_POINT('Ctrl Pts',(-2.49472245171096,-7.70567498120029,
20.));
#79686=CARTESIAN_POINT('Ctrl Pts',(-2.68607054417264,-7.62302655375222,
20.));
#79687=CARTESIAN_POINT('Ctrl Pts',(-2.87904124585084,-7.53967727740421,
20.));
#79688=CARTESIAN_POINT('Ctrl Pts',(-3.06851811319142,-7.44885967635279,
20.));
#79689=CARTESIAN_POINT('Ctrl Pts',(-3.25410368317141,-7.35085088042121,
20.));
#79690=CARTESIAN_POINT('Ctrl Pts',(-3.43972446834445,-7.25282348714573,
20.));
#79691=CARTESIAN_POINT('Ctrl Pts',(-3.62145303987379,-7.14760173869536,
20.));
#79692=CARTESIAN_POINT('Ctrl Pts',(-3.79886106473171,-7.03542097986013,
20.));
#79693=CARTESIAN_POINT('Ctrl Pts',(-3.97379582767289,-6.92480414350723,
20.));
#79694=CARTESIAN_POINT('Ctrl Pts',(-4.14453011452454,-6.80742049724289,
20.));
#79695=CARTESIAN_POINT('Ctrl Pts',(-4.3106161353842,-6.68346179753878,20.));
#79696=CARTESIAN_POINT('Ctrl Pts',(-4.40985285404803,-6.60939623473704,
20.));
#79697=CARTESIAN_POINT('Ctrl Pts',(-4.50742935975488,-6.53298270634048,
20.));
#79698=CARTESIAN_POINT('Ctrl Pts',(-4.60324267526068,-6.4542572598369,20.));
#79699=CARTESIAN_POINT('Ctrl Pts',(-4.64330692333192,-6.42133828817218,
20.));
#79700=CARTESIAN_POINT('Ctrl Pts',(-4.68306280802542,-6.38801504068871,
20.));
#79701=CARTESIAN_POINT('Ctrl Pts',(-4.72250247928215,-6.35428998788552,
20.));
#79702=CARTESIAN_POINT('Ctrl Pts',(-4.74163073925796,-6.337933320673,20.));
#79703=CARTESIAN_POINT('Ctrl Pts',(-4.76068461484216,-6.32148213722302,
20.));
#79704=CARTESIAN_POINT('Ctrl Pts',(-4.77966319360128,-6.3049367117326,20.));
#79705=CARTESIAN_POINT('Ctrl Pts',(-4.79836161285379,-6.28863552783164,
20.));
#79706=CARTESIAN_POINT('Ctrl Pts',(-4.8169807385683,-6.27224825184192,20.));
#79707=CARTESIAN_POINT('Ctrl Pts',(-4.83551632979225,-6.25577849640647,
20.));
#79708=CARTESIAN_POINT('Ctrl Pts',(-4.90102249955029,-6.19757314528533,
20.));
#79709=CARTESIAN_POINT('Ctrl Pts',(-4.96549967896505,-6.1383253473394,20.));
#79710=CARTESIAN_POINT('Ctrl Pts',(-5.02891936957257,-6.07805489113583,
20.));
#79711=CARTESIAN_POINT('Ctrl Pts',(-5.16122131629022,-5.95232266808482,
20.));
#79712=CARTESIAN_POINT('Ctrl Pts',(-5.2889225499224,-5.8221413942123,20.));
#79713=CARTESIAN_POINT('Ctrl Pts',(-5.41174699713132,-5.6876741775399,20.));
#79714=CARTESIAN_POINT('Ctrl Pts',(-5.55047495102833,-5.5357959296903,20.));
#79715=CARTESIAN_POINT('Ctrl Pts',(-5.68298253274711,-5.37845008269323,
20.));
#79716=CARTESIAN_POINT('Ctrl Pts',(-5.80904649119039,-5.21607619935368,
20.));
#79717=CARTESIAN_POINT('Ctrl Pts',(-5.93507016833321,-5.05375419944903,
20.));
#79718=CARTESIAN_POINT('Ctrl Pts',(-6.05465463020608,-4.88640671026504,
20.));
#79719=CARTESIAN_POINT('Ctrl Pts',(-6.16753024467367,-4.71444998079642,
20.));
#79720=CARTESIAN_POINT('Ctrl Pts',(-6.2794284648384,-4.54398223128607,20.));
#79721=CARTESIAN_POINT('Ctrl Pts',(-6.38473373606294,-4.36898406647204,
20.));
#79722=CARTESIAN_POINT('Ctrl Pts',(-6.48313389007494,-4.18984837043746,
20.));
#79723=CARTESIAN_POINT('Ctrl Pts',(-6.51307646148177,-4.13533846215649,
20.));
#79724=CARTESIAN_POINT('Ctrl Pts',(-6.54237929342843,-4.08044538787204,
20.));
#79725=CARTESIAN_POINT('Ctrl Pts',(-6.57103262208241,-4.02518012273521,
20.));
#79726=CARTESIAN_POINT('Ctrl Pts',(-6.58804424164497,-3.99236886799811,
20.));
#79727=CARTESIAN_POINT('Ctrl Pts',(-6.60482744441781,-3.95942536090239,
20.));
#79728=CARTESIAN_POINT('Ctrl Pts',(-6.62137866989648,-3.92635476092985,
20.));
#79729=CARTESIAN_POINT('Ctrl Pts',(-6.63484032288851,-3.8994573603934,20.));
#79730=CARTESIAN_POINT('Ctrl Pts',(-6.64814497160758,-3.87248289700163,
20.));
#79731=CARTESIAN_POINT('Ctrl Pts',(-6.66128676665324,-3.84544327824432,
20.));
#79732=CARTESIAN_POINT('Ctrl Pts',(-6.74965857407903,-3.66361575975182,
20.));
#79733=CARTESIAN_POINT('Ctrl Pts',(-6.83074267432777,-3.47869940087201,
20.));
#79734=CARTESIAN_POINT('Ctrl Pts',(-6.90433376409663,-3.29111212276483,
20.));
#79735=CARTESIAN_POINT('Ctrl Pts',(-6.97742456607799,-3.10480010263551,
20.));
#79736=CARTESIAN_POINT('Ctrl Pts',(-7.04312408996378,-2.91585269867224,
20.));
#79737=CARTESIAN_POINT('Ctrl Pts',(-7.10118275135911,-2.72466342156463,
20.));
#79738=CARTESIAN_POINT('Ctrl Pts',(-7.14172675958846,-2.5911505323915,20.));
#79739=CARTESIAN_POINT('Ctrl Pts',(-7.17854360492222,-2.45654402833867,
20.));
#79740=CARTESIAN_POINT('Ctrl Pts',(-7.21153332547604,-2.32097579245235,
20.));
#79741=CARTESIAN_POINT('Ctrl Pts',(-7.25901033828673,-2.12587335557664,
20.));
#79742=CARTESIAN_POINT('Ctrl Pts',(-7.29856290209612,-1.92877846178032,
20.));
#79743=CARTESIAN_POINT('Ctrl Pts',(-7.33014858423521,-1.730178804948,20.));
#79744=CARTESIAN_POINT('Ctrl Pts',(-7.35985701969858,-1.54338261476073,
20.));
#79745=CARTESIAN_POINT('Ctrl Pts',(-7.38251695926489,-1.35525473159528,
20.));
#79746=CARTESIAN_POINT('Ctrl Pts',(-7.39805210559582,-1.16621056513693,
20.));
#79747=CARTESIAN_POINT('Ctrl Pts',(-7.40002520954372,-1.14220024793611,
20.));
#79748=CARTESIAN_POINT('Ctrl Pts',(-7.40188332922168,-1.11817516864935,
20.));
#79749=CARTESIAN_POINT('Ctrl Pts',(-7.40362626288781,-1.09413619608073,
20.));
#79750=CARTESIAN_POINT('Ctrl Pts',(-7.4091558560377,-1.01787067856313,20.));
#79751=CARTESIAN_POINT('Ctrl Pts',(-7.41351801792253,-0.941576962387156,
20.));
#79752=CARTESIAN_POINT('Ctrl Pts',(-7.41671582489737,-0.865287042356737,
20.));
#79753=CARTESIAN_POINT('Ctrl Pts',(-7.4249990299845,-0.667675035545347,
20.));
#79754=CARTESIAN_POINT('Ctrl Pts',(-7.42547448855069,-0.470077078890568,
20.));
#79755=CARTESIAN_POINT('Ctrl Pts',(-7.41816552412071,-0.272959537946737,
20.));
#79756=CARTESIAN_POINT('Ctrl Pts',(-7.41087952338355,-0.0764613113672781,
20.));
#79757=CARTESIAN_POINT('Ctrl Pts',(-7.3958578295149,0.119560215190561,20.));
#79758=CARTESIAN_POINT('Ctrl Pts',(-7.37307242525166,0.314636346146562,
20.));
#79759=CARTESIAN_POINT('Ctrl Pts',(-7.35064888899275,0.506614361774566,
20.));
#79760=CARTESIAN_POINT('Ctrl Pts',(-7.32070608982365,0.697677381348684,
20.));
#79761=CARTESIAN_POINT('Ctrl Pts',(-7.28317013661821,0.887362522537855,
20.));
#79762=CARTESIAN_POINT('Ctrl Pts',(-7.25381516542289,1.03570568103745,20.));
#79763=CARTESIAN_POINT('Ctrl Pts',(-7.21981527655707,1.18320590660905,20.));
#79764=CARTESIAN_POINT('Ctrl Pts',(-7.18111555074975,1.32963115529216,20.));
#79765=CARTESIAN_POINT('Ctrl Pts',(-7.17837251511031,1.34000977341598,20.));
#79766=CARTESIAN_POINT('Ctrl Pts',(-7.17560586053976,1.35038298620668,20.));
#79767=CARTESIAN_POINT('Ctrl Pts',(-7.17281556424333,1.36075070882595,20.));
#79768=CARTESIAN_POINT('Ctrl Pts',(-7.15343328756475,1.4327681747096,20.));
#79769=CARTESIAN_POINT('Ctrl Pts',(-7.13291033139403,1.50452079254417,20.));
#79770=CARTESIAN_POINT('Ctrl Pts',(-7.11125559528035,1.57598286207429,20.));
#79771=CARTESIAN_POINT('Ctrl Pts',(-7.09847134652633,1.6181717333011,20.));
#79772=CARTESIAN_POINT('Ctrl Pts',(-7.08529281884788,1.66025871253416,20.));
#79773=CARTESIAN_POINT('Ctrl Pts',(-7.07172104727107,1.70224044505357,20.));
#79774=CARTESIAN_POINT('Ctrl Pts',(-7.06082391348468,1.73594868669759,20.));
#79775=CARTESIAN_POINT('Ctrl Pts',(-7.04967416834453,1.76958585825288,20.));
#79776=CARTESIAN_POINT('Ctrl Pts',(-7.03828051620722,1.80312734962223,20.));
#79777=CARTESIAN_POINT('Ctrl Pts',(-6.97573795221415,1.98724486041761,20.));
#79778=CARTESIAN_POINT('Ctrl Pts',(-6.9057979512053,2.16864460803966,20.));
#79779=CARTESIAN_POINT('Ctrl Pts',(-6.82870273039878,2.34690919602424,20.));
#79780=CARTESIAN_POINT('Ctrl Pts',(-6.75168682671949,2.52499038178417,20.));
#79781=CARTESIAN_POINT('Ctrl Pts',(-6.66752999543998,2.69994345768324,20.));
#79782=CARTESIAN_POINT('Ctrl Pts',(-6.57643092848617,2.87132309777343,20.));
#79783=CARTESIAN_POINT('Ctrl Pts',(-6.53499184911887,2.94928014766549,20.));
#79784=CARTESIAN_POINT('Ctrl Pts',(-6.49211576930227,3.02649734441682,20.));
#79785=CARTESIAN_POINT('Ctrl Pts',(-6.4478188151391,3.10293025460452,20.));
#79786=CARTESIAN_POINT('Ctrl Pts',(-6.41797151466939,3.15443077149655,20.));
#79787=CARTESIAN_POINT('Ctrl Pts',(-6.38747890509194,3.20557549284086,20.));
#79788=CARTESIAN_POINT('Ctrl Pts',(-6.35634612436391,3.25634942223226,20.));
#79789=CARTESIAN_POINT('Ctrl Pts',(-6.3377211957493,3.2867245056101,20.));
#79790=CARTESIAN_POINT('Ctrl Pts',(-6.31886976855288,3.31696247069953,20.));
#79791=CARTESIAN_POINT('Ctrl Pts',(-6.29980107815861,3.34704799429116,20.));
#79792=CARTESIAN_POINT('Ctrl Pts',(-6.19740680540357,3.50860000677472,20.));
#79793=CARTESIAN_POINT('Ctrl Pts',(-6.08868419402615,3.66586865351991,20.));
#79794=CARTESIAN_POINT('Ctrl Pts',(-5.97383605057998,3.81843153287768,20.));
#79795=CARTESIAN_POINT('Ctrl Pts',(-5.86059869604879,3.96885465979773,20.));
#79796=CARTESIAN_POINT('Ctrl Pts',(-5.74140596609826,4.11470355191866,20.));
#79797=CARTESIAN_POINT('Ctrl Pts',(-5.61641870165742,4.25553580582496,20.));
#79798=CARTESIAN_POINT('Ctrl Pts',(-5.55718805385751,4.32227529058214,20.));
#79799=CARTESIAN_POINT('Ctrl Pts',(-5.49665565046419,4.38788757250809,20.));
#79800=CARTESIAN_POINT('Ctrl Pts',(-5.43483636697226,4.45232211452012,20.));
#79801=CARTESIAN_POINT('Ctrl Pts',(-5.39406120686288,4.49482226364363,20.));
#79802=CARTESIAN_POINT('Ctrl Pts',(-5.35272615103,4.53680998101336,20.));
#79803=CARTESIAN_POINT('Ctrl Pts',(-5.3108423268622,4.57827606387112,20.));
#79804=CARTESIAN_POINT('Origin',(0.,0.,20.));
#79805=CARTESIAN_POINT('',(-60.,43.,20.));
#79806=CARTESIAN_POINT('',(-60.,-40.,20.));
#79807=CARTESIAN_POINT('',(-60.,40.,20.));
#79808=CARTESIAN_POINT('',(60.,-40.,20.));
#79809=CARTESIAN_POINT('',(-60.,-40.,20.));
#79810=CARTESIAN_POINT('',(60.,43.,20.));
#79811=CARTESIAN_POINT('',(60.,-40.,20.));
#79812=CARTESIAN_POINT('',(30.,43.,20.));
#79813=CARTESIAN_POINT('',(29.,7.34788079488412E-16,20.));
#79814=CARTESIAN_POINT('Origin',(35.,0.,20.));
#79815=CARTESIAN_POINT('',(-41.,7.34788079488412E-16,20.));
#79816=CARTESIAN_POINT('Origin',(-35.,0.,20.));
#79817=CARTESIAN_POINT('Origin',(-35.,0.,10.));
#79818=CARTESIAN_POINT('',(-41.,7.34788079488412E-16,0.));
#79819=CARTESIAN_POINT('',(-41.,7.34788079488412E-16,10.));
#79820=CARTESIAN_POINT('Origin',(-35.,0.,0.));
#79821=CARTESIAN_POINT('Origin',(35.,0.,10.));
#79822=CARTESIAN_POINT('',(29.,7.34788079488412E-16,0.));
#79823=CARTESIAN_POINT('',(29.,7.34788079488412E-16,10.));
#79824=CARTESIAN_POINT('Origin',(35.,0.,0.));
#79825=CARTESIAN_POINT('Origin',(60.,43.,0.));
#79826=CARTESIAN_POINT('',(60.,43.,0.));
#79827=CARTESIAN_POINT('',(-60.,43.,0.));
#79828=CARTESIAN_POINT('',(30.,43.,0.));
#79829=CARTESIAN_POINT('',(-60.,43.,0.));
#79830=CARTESIAN_POINT('',(60.,43.,0.));
#79831=CARTESIAN_POINT('Origin',(60.,-40.,0.));
#79832=CARTESIAN_POINT('',(60.,-40.,0.));
#79833=CARTESIAN_POINT('',(60.,-40.,0.));
#79834=CARTESIAN_POINT('',(60.,-40.,0.));
#79835=CARTESIAN_POINT('Origin',(-60.,-40.,0.));
#79836=CARTESIAN_POINT('',(-60.,-40.,0.));
#79837=CARTESIAN_POINT('',(-60.,-40.,0.));
#79838=CARTESIAN_POINT('',(-60.,-40.,0.));
#79839=CARTESIAN_POINT('Origin',(-60.,40.,0.));
#79840=CARTESIAN_POINT('',(-60.,40.,0.));
#79841=CARTESIAN_POINT('Origin',(0.,0.,0.));
#105785=UNCERTAINTY_MEASURE_WITH_UNIT(LENGTH_MEASURE(0.01),#105807,
'DISTANCE_ACCURACY_VALUE',
'Maximum model space distance between geometric entities at asserted c
onnectivities');
#105792=UNCERTAINTY_MEASURE_WITH_UNIT(LENGTH_MEASURE(0.01),#105807,
'DISTANCE_ACCURACY_VALUE',
'Maximum model space distance between geometric entities at asserted c
onnectivities');
#105799=(
GEOMETRIC_REPRESENTATION_CONTEXT(3)
GLOBAL_UNCERTAINTY_ASSIGNED_CONTEXT((#105785))
GLOBAL_UNIT_ASSIGNED_CONTEXT((#105807,#105809,#105810))
REPRESENTATION_CONTEXT('','3D')
);
#105806=(
GEOMETRIC_REPRESENTATION_CONTEXT(3)
GLOBAL_UNCERTAINTY_ASSIGNED_CONTEXT((#105792))
GLOBAL_UNIT_ASSIGNED_CONTEXT((#105807,#105809,#105810))
REPRESENTATION_CONTEXT('','3D')
);
#105807=(
LENGTH_UNIT()
NAMED_UNIT(*)
SI_UNIT(.MILLI.,.METRE.)
);
#105809=(
NAMED_UNIT(*)
PLANE_ANGLE_UNIT()
SI_UNIT($,.RADIAN.)
);
#105810=(
NAMED_UNIT(*)
SI_UNIT($,.STERADIAN.)
SOLID_ANGLE_UNIT()
);
#105817=SHAPE_DEFINITION_REPRESENTATION(#105830,#105864);
#105830=PRODUCT_DEFINITION_SHAPE('',$,#105878);
#105864=SHAPE_REPRESENTATION('',(#7538),#105799);
#105871=PRODUCT_DEFINITION_CONTEXT('part definition',#105912,'design');
#105878=PRODUCT_DEFINITION('End support','End support',#105891,#105871);
#105891=PRODUCT_DEFINITION_FORMATION('',$,#105920);
#105912=APPLICATION_CONTEXT(
'Core Data for Automotive Mechanical Design Process');
#105913=PRODUCT_CONTEXT('part definition',#105912,'mechanical');
#105920=PRODUCT('End support','End support',$,(#105913));
#105931=PRESENTATION_STYLE_ASSIGNMENT((#105937));
#105937=SURFACE_STYLE_USAGE(.BOTH.,#105943);
#105943=SURFACE_SIDE_STYLE('',(#105949));
#105949=SURFACE_STYLE_FILL_AREA(#105955);
#105955=FILL_AREA_STYLE('Opaque(23,69,131)',(#105961));
#105961=FILL_AREA_STYLE_COLOUR('Opaque(23,69,131)',#105967);
#105967=COLOUR_RGB('Opaque(23,69,131)',0.0901960784313725,0.270588235294118,
0.513725490196078);
ENDSEC;
END-ISO-10303-21;
